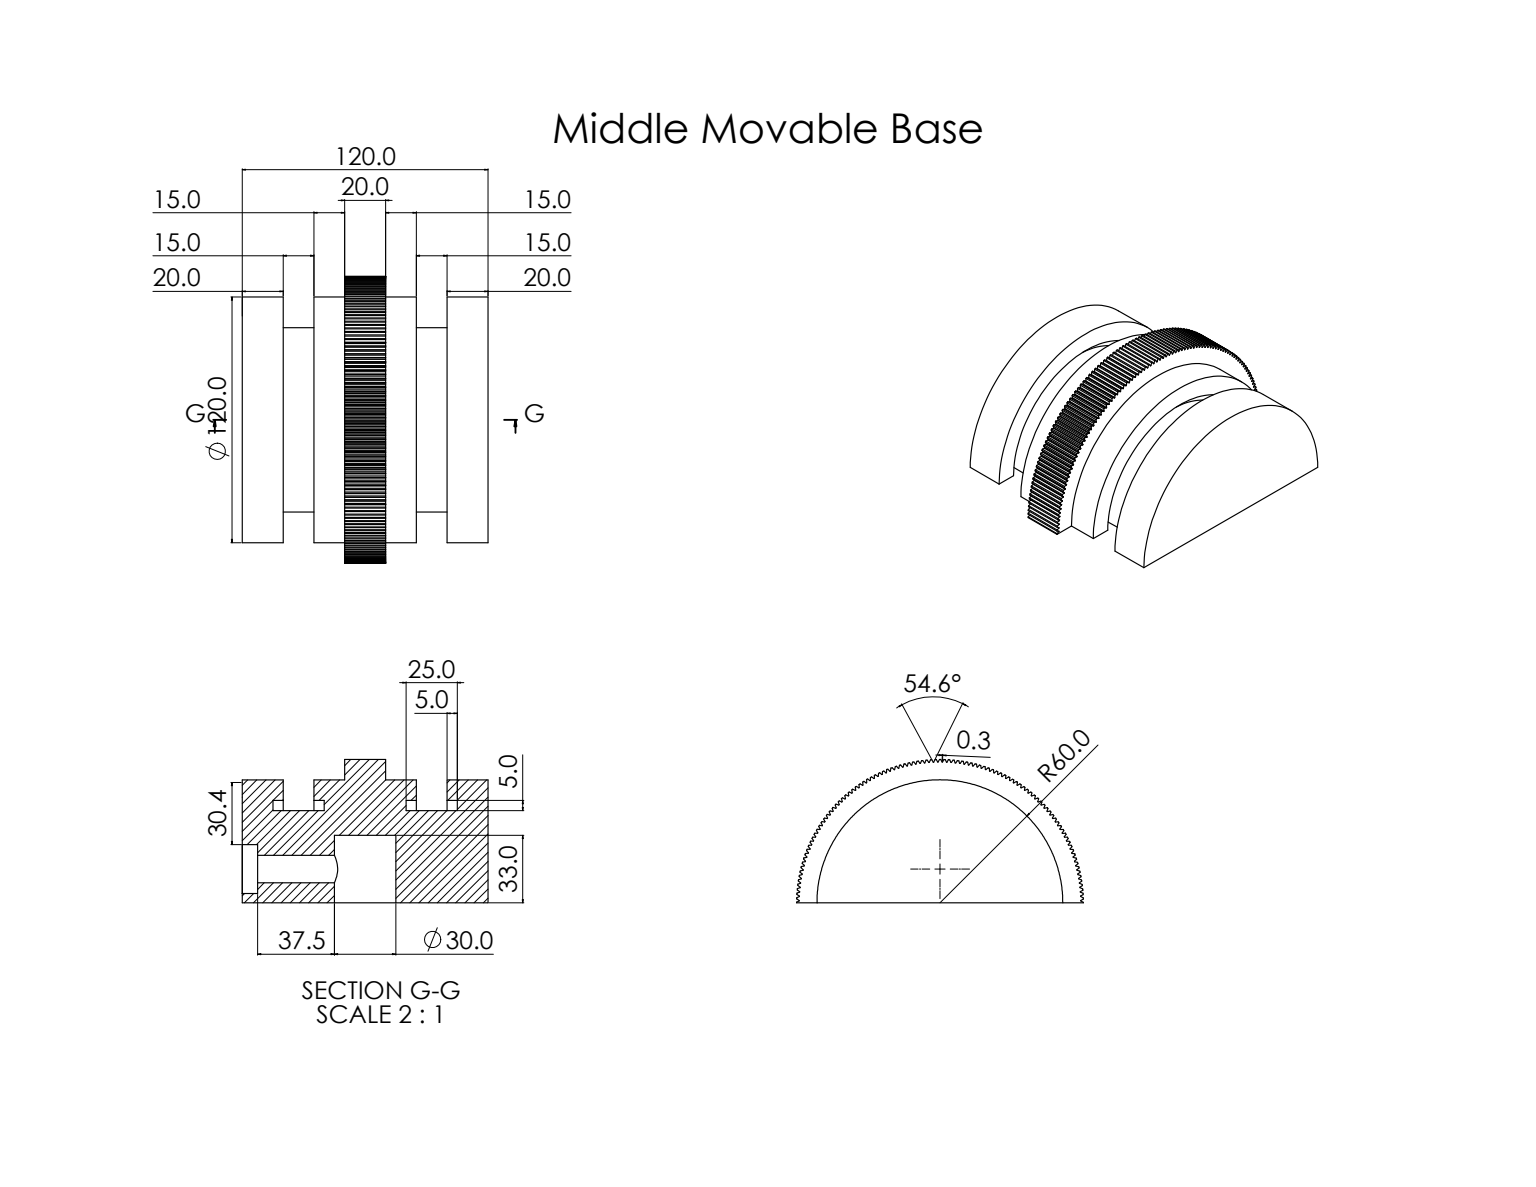
ISO-10303-21;
HEADER;
FILE_DESCRIPTION (('STEP AP214'),
    '1' );
FILE_NAME ('Middle Movable Base.step',
    '2026-10-24T22:31:37',
    ( '' ),
    ( '' ),
    'SwSTEP 2.0',
    'SolidWorks 2025',
    '' );
FILE_SCHEMA (( 'AUTOMOTIVE_DESIGN' ));
ENDSEC;

DATA;
#7=DIRECTION ( 'NONE',  ( -0.5866775868892348811, -0.8098206029990989707, 0.000000000000000000 ) ) ;
#27=DIRECTION ( 'NONE',  ( 0.06115825522547173321, -0.9981280818701455670, 0.000000000000000000 ) ) ;
#30=CARTESIAN_POINT ( 'NONE',  ( 30.34687108590969373, 93.06504152958497400, 45.00000000000000711 ) ) ;
#31=CARTESIAN_POINT ( 'NONE',  ( -19.65312891409030271, 93.06504152958497400, -10.00000000000000888 ) ) ;
#36=VECTOR ( 'NONE', #79966, 1000.000000000000000 ) ;
#39=DIRECTION ( 'NONE',  ( 0.000000000000000000, 0.000000000000000000, 1.000000000000000000 ) ) ;
#58=DIRECTION ( 'NONE',  ( -0.5866775868892348811, -0.8098206029990989707, 0.000000000000000000 ) ) ;
#69=EDGE_LOOP ( 'NONE', ( #91985, #84994, #72800, #59520 ) ) ;
#74=LINE ( 'NONE', #15241, #89935 ) ;
#76=CARTESIAN_POINT ( 'NONE',  ( 47.43014843991451102, 113.9519901285712251, 10.00000000000000000 ) ) ;
#82=LINE ( 'NONE', #92802, #76218 ) ;
#92=ORIENTED_EDGE ( 'NONE', *, *, #79784, .F. ) ;
#93=LINE ( 'NONE', #62359, #20761 ) ;
#99=ORIENTED_EDGE ( 'NONE', *, *, #21399, .F. ) ;
#100=CARTESIAN_POINT ( 'NONE',  ( -11.19568923542803773, 72.02527638617826256, 14.65695210810445737 ) ) ;
#102=FACE_OUTER_BOUND ( 'NONE', #93953, .T. ) ;
#105=ORIENTED_EDGE ( 'NONE', *, *, #46073, .T. ) ;
#118=CARTESIAN_POINT ( 'NONE',  ( 22.66956910419568061, 38.88013629349138256, -10.00000000000000000 ) ) ;
#128=AXIS2_PLACEMENT_3D ( 'NONE', #29113, #74733, #4299 ) ;
#144=DIRECTION ( 'NONE',  ( 1.000000000000000000, 0.000000000000000000, 0.000000000000000000 ) ) ;
#147=DIRECTION ( 'NONE',  ( -0.9979398670145497308, -0.06415622980648832963, 0.000000000000000000 ) ) ;
#157=DIRECTION ( 'NONE',  ( -1.000000000000000000, 0.000000000000000000, 0.000000000000000000 ) ) ;
#166=VERTEX_POINT ( 'NONE', #35811 ) ;
#179=VERTEX_POINT ( 'NONE', #22103 ) ;
#180=CARTESIAN_POINT ( 'NONE',  ( 43.35468487962021555, 120.5828561944265687, -10.00000000000000000 ) ) ;
#182=DIRECTION ( 'NONE',  ( -0.8770933717188628131, -0.4803199113995136327, 0.000000000000000000 ) ) ;
#185=CARTESIAN_POINT ( 'NONE',  ( -77.58047734835668052, 56.02942318228900120, 10.00000000000000000 ) ) ;
#186=EDGE_CURVE ( 'NONE', #58877, #48375, #99124, .T. ) ;
#187=CARTESIAN_POINT ( 'NONE',  ( -37.40701240123932791, 25.35389310390295847, 177.5919119679930134 ) ) ;
#191=VECTOR ( 'NONE', #26487, 1000.000000000000000 ) ;
#192=DIRECTION ( 'NONE',  ( -0.2575544297740129385, 0.9662637919863205083, 0.000000000000000000 ) ) ;
#195=LINE ( 'NONE', #21507, #68091 ) ;
#198=LINE ( 'NONE', #694, #6256 ) ;
#199=DIRECTION ( 'NONE',  ( -0.1269555777209495084, -0.9919084036772447543, 0.000000000000000000 ) ) ;
#201=DIRECTION ( 'NONE',  ( -0.9956898167541090583, 0.09274582908232942291, 0.000000000000000000 ) ) ;
#205=ORIENTED_EDGE ( 'NONE', *, *, #96749, .F. ) ;
#209=ORIENTED_EDGE ( 'NONE', *, *, #18748, .T. ) ;
#210=ADVANCED_FACE ( 'NONE', ( #82475 ), #75330, .F. ) ;
#211=EDGE_CURVE ( 'NONE', #97533, #84233, #8682, .T. ) ;
#212=ORIENTED_EDGE ( 'NONE', *, *, #13551, .F. ) ;
#213=VERTEX_POINT ( 'NONE', #51000 ) ;
#215=ORIENTED_EDGE ( 'NONE', *, *, #48377, .F. ) ;
#216=CARTESIAN_POINT ( 'NONE',  ( -34.42581292930597670, 25.91608375674935161, -10.00000000000000000 ) ) ;
#223=EDGE_CURVE ( 'NONE', #61495, #4321, #98638, .T. ) ;
#226=CARTESIAN_POINT ( 'NONE',  ( -38.08094845355783065, 65.40755614729289391, -10.00000000000000000 ) ) ;
#231=EDGE_LOOP ( 'NONE', ( #23374, #30336, #91707, #91795 ) ) ;
#234=CARTESIAN_POINT ( 'NONE',  ( 32.49301573174289359, 102.6727471919249552, 59.99999999999999289 ) ) ;
#235=EDGE_CURVE ( 'NONE', #80145, #45676, #581, .T. ) ;
#237=PLANE ( 'NONE',  #70015 ) ;
#241=ORIENTED_EDGE ( 'NONE', *, *, #65257, .F. ) ;
#243=CARTESIAN_POINT ( 'NONE',  ( -5.171971415982786979, 24.31384663199769491, -10.00000000000000000 ) ) ;
#249=CARTESIAN_POINT ( 'NONE',  ( 19.31801425620939483, 115.5650415295850451, 45.00000000000000711 ) ) ;
#251=DIRECTION ( 'NONE',  ( -0.7299047266382377996, 0.6835488936653758563, 0.000000000000000000 ) ) ;
#253=LINE ( 'NONE', #93489, #65775 ) ;
#260=VECTOR ( 'NONE', #98642, 1000.000000000000000 ) ;
#270=DIRECTION ( 'NONE',  ( 0.000000000000000000, 0.000000000000000000, 1.000000000000000000 ) ) ;
#280=FACE_OUTER_BOUND ( 'NONE', #77196, .T. ) ;
#282=CARTESIAN_POINT ( 'NONE',  ( 45.86253193465722688, 68.41350641406140198, -10.00000000000000000 ) ) ;
#287=EDGE_CURVE ( 'NONE', #95521, #97948, #4932, .T. ) ;
#289=CARTESIAN_POINT ( 'NONE',  ( 48.58805178314242568, 84.67719436603331928, -10.00000000000000000 ) ) ;
#295=DIRECTION ( 'NONE',  ( -0.000000000000000000, 0.000000000000000000, -1.000000000000000000 ) ) ;
#297=ORIENTED_EDGE ( 'NONE', *, *, #4120, .T. ) ;
#303=EDGE_CURVE ( 'NONE', #60481, #57725, #20128, .T. ) ;
#304=ORIENTED_EDGE ( 'NONE', *, *, #16098, .T. ) ;
#317=CARTESIAN_POINT ( 'NONE',  ( -19.77952770554638207, 93.00072136042149396, 59.99999999999999289 ) ) ;
#326=DIRECTION ( 'NONE',  ( 0.2091919045418403900, 0.9778746070300412541, 0.000000000000000000 ) ) ;
#333=ORIENTED_EDGE ( 'NONE', *, *, #33379, .F. ) ;
#337=CARTESIAN_POINT ( 'NONE',  ( 48.83428215874786815, 87.09189275153327969, -10.00000000000000000 ) ) ;
#353=DIRECTION ( 'NONE',  ( -0.000000000000000000, -0.000000000000000000, 1.000000000000000000 ) ) ;
#354=CARTESIAN_POINT ( 'NONE',  ( -19.56589364647650697, 93.17686168307763239, 59.99999999999999289 ) ) ;
#357=CARTESIAN_POINT ( 'NONE',  ( -54.25007008209492199, 32.21233689110872689, 10.00000000000000000 ) ) ;
#366=LINE ( 'NONE', #79411, #99707 ) ;
#367=ORIENTED_EDGE ( 'NONE', *, *, #49379, .F. ) ;
#372=PLANE ( 'NONE',  #40302 ) ;
#384=CARTESIAN_POINT ( 'NONE',  ( 45.79324619304848909, 117.8999360398438512, 177.5919119679930134 ) ) ;
#390=CARTESIAN_POINT ( 'NONE',  ( -59.85755863633952600, 35.44530052843370527, 10.00000000000000000 ) ) ;
#392=DIRECTION ( 'NONE',  ( -1.000000000000000000, 0.000000000000000000, 0.000000000000000000 ) ) ;
#393=EDGE_CURVE ( 'NONE', #90851, #29361, #37739, .T. ) ;
#414=DIRECTION ( 'NONE',  ( -0.2270762630343793331, 0.9738769792773321887, 0.000000000000000000 ) ) ;
#433=CARTESIAN_POINT ( 'NONE',  ( 32.24342178309110096, 47.97677246190463052, 10.00000000000000000 ) ) ;
#438=CARTESIAN_POINT ( 'NONE',  ( -47.78078991586326651, 28.96484896693080913, -10.00000000000000000 ) ) ;
#442=LINE ( 'NONE', #39415, #16658 ) ;
#451=AXIS2_PLACEMENT_3D ( 'NONE', #67847, #36429, #6548 ) ;
#466=VECTOR ( 'NONE', #65332, 1000.000000000000114 ) ;
#472=ORIENTED_EDGE ( 'NONE', *, *, #57842, .T. ) ;
#477=DIRECTION ( 'NONE',  ( -0.000000000000000000, 0.000000000000000000, 1.000000000000000000 ) ) ;
#484=ADVANCED_BREP_SHAPE_REPRESENTATION ( '', ( #42857, #68784 ), #81782 ) ;
#485=ORIENTED_EDGE ( 'NONE', *, *, #51159, .T. ) ;
#494=CARTESIAN_POINT ( 'NONE',  ( -80.08603253397791377, 57.73992072201551906, 177.5919119679930134 ) ) ;
#498=CARTESIAN_POINT ( 'NONE',  ( -59.87889494062799400, 37.30571521936384016, 10.00000000000000000 ) ) ;
#509=FACE_OUTER_BOUND ( 'NONE', #80990, .T. ) ;
#511=VERTEX_POINT ( 'NONE', #55477 ) ;
#515=CARTESIAN_POINT ( 'NONE',  ( -29.31672308591111431, 23.47304723416778316, -10.00000000000000000 ) ) ;
#518=CIRCLE ( 'NONE', #92746, 0.1418229129680845801 ) ;
#521=FACE_OUTER_BOUND ( 'NONE', #76798, .T. ) ;
#525=CARTESIAN_POINT ( 'NONE',  ( 48.98007068238331385, 88.97864505566217019, 10.00000000000000000 ) ) ;
#526=VERTEX_POINT ( 'NONE', #86463 ) ;
#527=VECTOR ( 'NONE', #79353, 1000.000000000000000 ) ;
#540=EDGE_CURVE ( 'NONE', #56147, #90103, #63596, .T. ) ;
#553=PLANE ( 'NONE',  #11961 ) ;
#560=DIRECTION ( 'NONE',  ( -0.000000000000000000, -0.000000000000000000, -1.000000000000000000 ) ) ;
#561=ORIENTED_EDGE ( 'NONE', *, *, #16214, .T. ) ;
#566=VERTEX_POINT ( 'NONE', #60825 ) ;
#575=ORIENTED_EDGE ( 'NONE', *, *, #83693, .F. ) ;
#581=CIRCLE ( 'NONE', #62027, 70.00000000000001421 ) ;
#582=ORIENTED_EDGE ( 'NONE', *, *, #61102, .F. ) ;
#583=DIRECTION ( 'NONE',  ( -0.000000000000000000, -0.000000000000000000, -1.000000000000000000 ) ) ;
#590=CARTESIAN_POINT ( 'NONE',  ( -8.413379660334708632, 72.70744834316617755, 14.99993878877685916 ) ) ;
#591=LINE ( 'NONE', #85759, #53118 ) ;
#627=ADVANCED_FACE ( 'NONE', ( #24842 ), #553, .F. ) ;
#642=DIRECTION ( 'NONE',  ( -0.000000000000000000, 0.000000000000000000, 1.000000000000000000 ) ) ;
#652=DIRECTION ( 'NONE',  ( 0.000000000000000000, 0.000000000000000000, 1.000000000000000000 ) ) ;
#654=DIRECTION ( 'NONE',  ( 0.3074612162317589825, -0.9515606131578205895, 0.000000000000000000 ) ) ;
#673=VECTOR ( 'NONE', #77839, 1000.000000000000227 ) ;
#676=ORIENTED_EDGE ( 'NONE', *, *, #27395, .T. ) ;
#694=CARTESIAN_POINT ( 'NONE',  ( 48.58805178314242568, 84.67719436603331928, 10.00000000000000000 ) ) ;
#697=CARTESIAN_POINT ( 'NONE',  ( -74.97640825042664403, 52.25402898078436920, -10.00000000000000000 ) ) ;
#701=ORIENTED_EDGE ( 'NONE', *, *, #49835, .T. ) ;
#703=DIRECTION ( 'NONE',  ( 0.000000000000000000, 0.000000000000000000, 1.000000000000000000 ) ) ;
#706=ORIENTED_EDGE ( 'NONE', *, *, #49315, .T. ) ;
#709=VERTEX_POINT ( 'NONE', #54730 ) ;
#710=DIRECTION ( 'NONE',  ( -0.6141984594095433181, -0.7891516029629183082, 0.000000000000000000 ) ) ;
#717=DIRECTION ( 'NONE',  ( 1.000000000000000000, -2.577303450022684150E-15, 0.000000000000000000 ) ) ;
#720=EDGE_CURVE ( 'NONE', #17180, #93223, #32942, .T. ) ;
#724=ORIENTED_EDGE ( 'NONE', *, *, #71091, .F. ) ;
#726=CARTESIAN_POINT ( 'NONE',  ( -72.48190909937208914, 49.06123820388767598, -10.00000000000000000 ) ) ;
#728=DIRECTION ( 'NONE',  ( -0.000000000000000000, -0.000000000000000000, -1.000000000000000000 ) ) ;
#760=CARTESIAN_POINT ( 'NONE',  ( -14.53296615039140960, 35.34728565592875071, 59.99999999999999289 ) ) ;
#764=LINE ( 'NONE', #54961, #11155 ) ;
#771=LINE ( 'NONE', #16967, #7881 ) ;
#775=ORIENTED_EDGE ( 'NONE', *, *, #59166, .F. ) ;
#782=FACE_OUTER_BOUND ( 'NONE', #41307, .T. ) ;
#796=ADVANCED_FACE ( 'NONE', ( #63846 ), #32453, .F. ) ;
#797=ORIENTED_EDGE ( 'NONE', *, *, #34932, .T. ) ;
#802=CARTESIAN_POINT ( 'NONE',  ( 39.77289032284285497, 58.49985355908045648, -10.00000000000000000 ) ) ;
#812=CIRCLE ( 'NONE', #62261, 70.00000000000001421 ) ;
#820=CARTESIAN_POINT ( 'NONE',  ( 18.86034532297697908, 34.61239144260639478, -10.00000000000000000 ) ) ;
#824=ORIENTED_EDGE ( 'NONE', *, *, #18196, .F. ) ;
#843=VECTOR ( 'NONE', #25615, 1000.000000000000000 ) ;
#861=VERTEX_POINT ( 'NONE', #26360 ) ;
#871=ORIENTED_EDGE ( 'NONE', *, *, #19349, .T. ) ;
#877=ADVANCED_FACE ( 'NONE', ( #35443 ), #33453, .F. ) ;
#880=VECTOR ( 'NONE', #94818, 999.9999999999998863 ) ;
#882=FACE_OUTER_BOUND ( 'NONE', #77373, .T. ) ;
#895=DIRECTION ( 'NONE',  ( 1.000000000000000000, 0.000000000000000000, 0.000000000000000000 ) ) ;
#899=EDGE_CURVE ( 'NONE', #47394, #59009, #20762, .T. ) ;
#910=EDGE_CURVE ( 'NONE', #22139, #62627, #36935, .T. ) ;
#913=CARTESIAN_POINT ( 'NONE',  ( -54.24312371938221133, 45.66933727564025247, 59.99999999999999289 ) ) ;
#915=CARTESIAN_POINT ( 'NONE',  ( -37.96271243472389756, 25.23297040071578223, -10.00000000000000000 ) ) ;
#916=VECTOR ( 'NONE', #19818, 1000.000000000000000 ) ;
#926=PLANE ( 'NONE',  #45711 ) ;
#934=VERTEX_POINT ( 'NONE', #51650 ) ;
#942=DIRECTION ( 'NONE',  ( -0.000000000000000000, -0.000000000000000000, -1.000000000000000000 ) ) ;
#943=ORIENTED_EDGE ( 'NONE', *, *, #73759, .T. ) ;
#946=FACE_OUTER_BOUND ( 'NONE', #38925, .T. ) ;
#953=ORIENTED_EDGE ( 'NONE', *, *, #83634, .T. ) ;
#956=AXIS2_PLACEMENT_3D ( 'NONE', #84126, #36465, #99782 ) ;
#961=CYLINDRICAL_SURFACE ( 'NONE', #15742, 70.00000000000002842 ) ;
#981=DIRECTION ( 'NONE',  ( -0.9999990636452668058, -0.001368469433204011270, 0.000000000000000000 ) ) ;
#984=ORIENTED_EDGE ( 'NONE', *, *, #57106, .F. ) ;
#988=LINE ( 'NONE', #76978, #61278 ) ;
#989=EDGE_CURVE ( 'NONE', #100173, #64867, #53135, .T. ) ;
#991=VECTOR ( 'NONE', #68257, 1000.000000000000000 ) ;
#996=EDGE_LOOP ( 'NONE', ( #34380, #44799, #80487, #3308 ) ) ;
#1005=CARTESIAN_POINT ( 'NONE',  ( 50.33662733789741139, 94.26254718190894266, -10.00000000000000000 ) ) ;
#1023=LINE ( 'NONE', #92751, #45256 ) ;
#1027=EDGE_CURVE ( 'NONE', #65437, #26008, #58647, .T. ) ;
#1030=VERTEX_POINT ( 'NONE', #52623 ) ;
#1052=CARTESIAN_POINT ( 'NONE',  ( -4.696103426644111956, 79.65490786025929992, 13.63766756523351020 ) ) ;
#1054=DIRECTION ( 'NONE',  ( -0.9954067278227237692, 0.09573633691163400961, 0.000000000000000000 ) ) ;
#1064=VECTOR ( 'NONE', #92848, 999.9999999999998863 ) ;
#1080=ORIENTED_EDGE ( 'NONE', *, *, #21239, .T. ) ;
#1085=EDGE_CURVE ( 'NONE', #56387, #18338, #31160, .T. ) ;
#1091=CIRCLE ( 'NONE', #54496, 70.00000000000001421 ) ;
#1098=VERTEX_POINT ( 'NONE', #99752 ) ;
#1101=DIRECTION ( 'NONE',  ( 1.000000000000000000, 1.070572202317114942E-14, 0.000000000000000000 ) ) ;
#1102=CIRCLE ( 'NONE', #14042, 70.00000000000001421 ) ;
#1103=VERTEX_POINT ( 'NONE', #60710 ) ;
#1122=DIRECTION ( 'NONE',  ( -1.000000000000000000, 0.000000000000000000, 0.000000000000000000 ) ) ;
#1126=EDGE_CURVE ( 'NONE', #56387, #14902, #59211, .T. ) ;
#1143=ORIENTED_EDGE ( 'NONE', *, *, #74016, .T. ) ;
#1144=CARTESIAN_POINT ( 'NONE',  ( -19.70914744582199774, 92.93475084401866582, 59.99999999999999289 ) ) ;
#1150=CARTESIAN_POINT ( 'NONE',  ( -30.95603806669010183, 23.98360954755323604, 177.5919119679930134 ) ) ;
#1152=VECTOR ( 'NONE', #12982, 1000.000000000000000 ) ;
#1153=EDGE_CURVE ( 'NONE', #7407, #88206, #54605, .T. ) ;
#1156=ORIENTED_EDGE ( 'NONE', *, *, #93985, .F. ) ;
#1161=CIRCLE ( 'NONE', #65869, 0.1418229129681522482 ) ;
#1162=CARTESIAN_POINT ( 'NONE',  ( 49.07456115661583596, 91.13648234292965356, -10.00000000000000000 ) ) ;
#1170=ORIENTED_EDGE ( 'NONE', *, *, #72286, .F. ) ;
#1173=DIRECTION ( 'NONE',  ( -0.8965230319888208843, 0.4429971254010250936, 0.000000000000000000 ) ) ;
#1174=VECTOR ( 'NONE', #10627, 1000.000000000000000 ) ;
#1178=DIRECTION ( 'NONE',  ( 0.000000000000000000, 0.000000000000000000, 1.000000000000000000 ) ) ;
#1184=ORIENTED_EDGE ( 'NONE', *, *, #47229, .T. ) ;
#1186=EDGE_CURVE ( 'NONE', #36969, #71264, #84573, .T. ) ;
#1197=VERTEX_POINT ( 'NONE', #62209 ) ;
#1199=FACE_OUTER_BOUND ( 'NONE', #92317, .T. ) ;
#1203=CARTESIAN_POINT ( 'NONE',  ( 10.24016918245798990, 49.27098784156451217, 59.99999999999999289 ) ) ;
#1204=ORIENTED_EDGE ( 'NONE', *, *, #57213, .F. ) ;
#1210=ORIENTED_EDGE ( 'NONE', *, *, #81477, .F. ) ;
#1216=ORIENTED_EDGE ( 'NONE', *, *, #59052, .T. ) ;
#1217=ORIENTED_EDGE ( 'NONE', *, *, #67248, .F. ) ;
#1218=VERTEX_POINT ( 'NONE', #22738 ) ;
#1220=ORIENTED_EDGE ( 'NONE', *, *, #11993, .T. ) ;
#1228=FACE_OUTER_BOUND ( 'NONE', #56169, .T. ) ;
#1229=DIRECTION ( 'NONE',  ( -0.9515606131578174809, -0.3074612162317687525, 0.000000000000000000 ) ) ;
#1235=VERTEX_POINT ( 'NONE', #433 ) ;
#1247=VECTOR ( 'NONE', #98615, 1000.000000000000000 ) ;
#1257=DIRECTION ( 'NONE',  ( -0.9054088711727240613, 0.4245406647209821749, 0.000000000000000000 ) ) ;
#1261=EDGE_LOOP ( 'NONE', ( #21247, #73872, #79004, #53676 ) ) ;
#1262=ORIENTED_EDGE ( 'NONE', *, *, #86789, .T. ) ;
#1272=AXIS2_PLACEMENT_3D ( 'NONE', #72427, #95248, #88660 ) ;
#1277=CIRCLE ( 'NONE', #57894, 0.1418229129681557177 ) ;
#1280=VECTOR ( 'NONE', #33335, 1000.000000000000227 ) ;
#1281=DIRECTION ( 'NONE',  ( 0.8599083858334037878, -0.5104483989331242144, 0.000000000000000000 ) ) ;
#1290=VERTEX_POINT ( 'NONE', #69581 ) ;
#1297=PLANE ( 'NONE',  #6369 ) ;
#1298=VECTOR ( 'NONE', #47765, 1000.000000000000114 ) ;
#1300=DIRECTION ( 'NONE',  ( 0.9616534368410327716, -0.2742675106749429270, 0.000000000000000000 ) ) ;
#1304=EDGE_CURVE ( 'NONE', #56569, #52500, #99009, .T. ) ;
#1316=EDGE_CURVE ( 'NONE', #35809, #20300, #83330, .T. ) ;
#1319=AXIS2_PLACEMENT_3D ( 'NONE', #28738, #47412, #55498 ) ;
#1320=ORIENTED_EDGE ( 'NONE', *, *, #44937, .T. ) ;
#1324=ORIENTED_EDGE ( 'NONE', *, *, #63685, .T. ) ;
#1333=CARTESIAN_POINT ( 'NONE',  ( 38.19908180566553568, 96.33262850695970769, 59.99999999999999289 ) ) ;
#1334=DIRECTION ( 'NONE',  ( -0.1344185706417126702, 0.9909246428798905715, 0.000000000000000000 ) ) ;
#1336=ORIENTED_EDGE ( 'NONE', *, *, #16346, .T. ) ;
#1339=ORIENTED_EDGE ( 'NONE', *, *, #72669, .F. ) ;
#1353=VECTOR ( 'NONE', #63954, 1000.000000000000000 ) ;
#1359=AXIS2_PLACEMENT_3D ( 'NONE', #81029, #56669, #96213 ) ;
#1363=EDGE_CURVE ( 'NONE', #22179, #13198, #68582, .T. ) ;
#1368=DIRECTION ( 'NONE',  ( 0.9481851146622169990, 0.3177184104407523302, 0.000000000000000000 ) ) ;
#1371=DIRECTION ( 'NONE',  ( -0.000000000000000000, 0.000000000000000000, 1.000000000000000000 ) ) ;
#1376=VERTEX_POINT ( 'NONE', #59470 ) ;
#1377=EDGE_CURVE ( 'NONE', #70239, #29279, #92426, .T. ) ;
#1379=EDGE_CURVE ( 'NONE', #37194, #36369, #53381, .T. ) ;
#1380=VECTOR ( 'NONE', #44212, 1000.000000000000000 ) ;
#1398=AXIS2_PLACEMENT_3D ( 'NONE', #5621, #66429, #99340 ) ;
#1428=EDGE_CURVE ( 'NONE', #28142, #18551, #60972, .T. ) ;
#1434=PLANE ( 'NONE',  #38359 ) ;
#1436=VECTOR ( 'NONE', #17514, 1000.000000000000000 ) ;
#1438=DIRECTION ( 'NONE',  ( 1.000000000000000000, 0.000000000000000000, 0.000000000000000000 ) ) ;
#1442=AXIS2_PLACEMENT_3D ( 'NONE', #13783, #67983, #44661 ) ;
#1454=ORIENTED_EDGE ( 'NONE', *, *, #94923, .T. ) ;
#1455=CARTESIAN_POINT ( 'NONE',  ( -42.18579364100346396, 26.51648975995176372, -10.00000000000000000 ) ) ;
#1459=VECTOR ( 'NONE', #70154, 1000.000000000000227 ) ;
#1466=DIRECTION ( 'NONE',  ( -0.000000000000000000, 0.000000000000000000, -1.000000000000000000 ) ) ;
#1468=LINE ( 'NONE', #48042, #82103 ) ;
#1473=CARTESIAN_POINT ( 'NONE',  ( -19.65312891409030271, 93.06504152958497400, 10.00000000000000888 ) ) ;
#1479=DIRECTION ( 'NONE',  ( -0.4805540241036398430, -0.8769651246872923744, 0.000000000000000000 ) ) ;
#1484=ORIENTED_EDGE ( 'NONE', *, *, #28389, .T. ) ;
#1487=ORIENTED_EDGE ( 'NONE', *, *, #98535, .T. ) ;
#1499=VECTOR ( 'NONE', #42114, 1000.000000000000000 ) ;
#1513=EDGE_CURVE ( 'NONE', #39405, #4020, #94422, .T. ) ;
#1517=CARTESIAN_POINT ( 'NONE',  ( -4.164184202058353712, 36.47075635815506445, 59.99999999999999289 ) ) ;
#1534=LINE ( 'NONE', #95271, #4496 ) ;
#1538=CARTESIAN_POINT ( 'NONE',  ( -19.65312891409030271, 93.06504152958497400, -20.00000000000000355 ) ) ;
#1545=LINE ( 'NONE', #8630, #17652 ) ;
#1568=FACE_OUTER_BOUND ( 'NONE', #50419, .T. ) ;
#1569=ORIENTED_EDGE ( 'NONE', *, *, #56933, .F. ) ;
#1571=LINE ( 'NONE', #30084, #19936 ) ;
#1579=CIRCLE ( 'NONE', #89003, 70.00000000000001421 ) ;
#1583=EDGE_CURVE ( 'NONE', #75006, #51318, #47275, .T. ) ;
#1592=VERTEX_POINT ( 'NONE', #42660 ) ;
#1595=ORIENTED_EDGE ( 'NONE', *, *, #6391, .T. ) ;
#1603=AXIS2_PLACEMENT_3D ( 'NONE', #71225, #8410, #94542 ) ;
#1621=CARTESIAN_POINT ( 'NONE',  ( 20.94141239725287917, 35.71947554534623492, -10.00000000000000000 ) ) ;
#1624=LINE ( 'NONE', #53298, #100278 ) ;
#1628=EDGE_CURVE ( 'NONE', #64662, #76974, #18907, .T. ) ;
#1636=ORIENTED_EDGE ( 'NONE', *, *, #79163, .F. ) ;
#1644=VERTEX_POINT ( 'NONE', #91305 ) ;
#1653=PLANE ( 'NONE',  #7779 ) ;
#1666=ORIENTED_EDGE ( 'NONE', *, *, #83634, .F. ) ;
#1673=DIRECTION ( 'NONE',  ( 0.4140345431502788220, 0.9102611697080897901, 0.000000000000000000 ) ) ;
#1691=CARTESIAN_POINT ( 'NONE',  ( 31.79857739925353499, 98.44139654353648439, 59.99999999999999289 ) ) ;
#1696=CARTESIAN_POINT ( 'NONE',  ( -0.2492734796364602656, 27.10516647459198225, -10.00000000000000000 ) ) ;
#1707=EDGE_CURVE ( 'NONE', #24773, #78854, #42513, .T. ) ;
#1711=ORIENTED_EDGE ( 'NONE', *, *, #9867, .F. ) ;
#1716=CARTESIAN_POINT ( 'NONE',  ( 27.76992210170819675, 43.29297894285233639, -10.00000000000000000 ) ) ;
#1725=VERTEX_POINT ( 'NONE', #61355 ) ;
#1731=CARTESIAN_POINT ( 'NONE',  ( 3.854092266844447501, 28.45370138451379560, 10.00000000000000000 ) ) ;
#1733=VERTEX_POINT ( 'NONE', #59861 ) ;
#1734=VERTEX_POINT ( 'NONE', #21866 ) ;
#1745=ORIENTED_EDGE ( 'NONE', *, *, #19548, .F. ) ;
#1754=ADVANCED_FACE ( 'NONE', ( #98395 ), #22860, .F. ) ;
#1756=LINE ( 'NONE', #79786, #92698 ) ;
#1766=DIRECTION ( 'NONE',  ( -0.9182972510888883777, 0.3958915996110437541, 0.000000000000000000 ) ) ;
#1789=DIRECTION ( 'NONE',  ( -0.5803476755362181327, -0.8143688203140567738, 0.000000000000000000 ) ) ;
#1802=DIRECTION ( 'NONE',  ( -0.2197389712097134185, -0.9755587037855265597, 0.000000000000000000 ) ) ;
#1810=LINE ( 'NONE', #17499, #37592 ) ;
#1821=ORIENTED_EDGE ( 'NONE', *, *, #26693, .F. ) ;
#1822=LINE ( 'NONE', #8908, #48804 ) ;
#1835=DIRECTION ( 'NONE',  ( 0.000000000000000000, 0.000000000000000000, 1.000000000000000000 ) ) ;
#1844=ORIENTED_EDGE ( 'NONE', *, *, #76284, .F. ) ;
#1851=CARTESIAN_POINT ( 'NONE',  ( -8.669243101527598583, 25.19333184544593252, -10.00000000000000000 ) ) ;
#1860=VERTEX_POINT ( 'NONE', #15750 ) ;
#1866=CARTESIAN_POINT ( 'NONE',  ( -31.49789205211705934, 23.81092751074078606, -10.00000000000000000 ) ) ;
#1869=AXIS2_PLACEMENT_3D ( 'NONE', #180, #45756, #59965 ) ;
#1870=CARTESIAN_POINT ( 'NONE',  ( 22.87549206224920084, 39.05096577487528720, -10.00000000000000000 ) ) ;
#1871=ORIENTED_EDGE ( 'NONE', *, *, #27551, .T. ) ;
#1876=PLANE ( 'NONE',  #87255 ) ;
#1879=DIRECTION ( 'NONE',  ( -0.9606745773021557744, 0.2776767122488390527, 0.000000000000000000 ) ) ;
#1880=EDGE_CURVE ( 'NONE', #50442, #29620, #8170, .T. ) ;
#1885=EDGE_LOOP ( 'NONE', ( #41574, #54395, #87632, #40774 ) ) ;
#1888=LINE ( 'NONE', #72303, #26415 ) ;
#1903=FACE_OUTER_BOUND ( 'NONE', #32599, .T. ) ;
#1907=DIRECTION ( 'NONE',  ( 1.000000000000000000, 0.000000000000000000, 0.000000000000000000 ) ) ;
#1919=CARTESIAN_POINT ( 'NONE',  ( -19.65312891409030271, 93.06504152958497400, -10.00000000000000888 ) ) ;
#1921=DIRECTION ( 'NONE',  ( 1.000000000000000000, -1.199437374818249260E-13, 0.000000000000000000 ) ) ;
#1926=EDGE_LOOP ( 'NONE', ( #76923, #39186, #42296, #5688 ) ) ;
#1935=DIRECTION ( 'NONE',  ( 0.4242989612870596283, -0.9055221650797523614, 0.000000000000000000 ) ) ;
#1937=ORIENTED_EDGE ( 'NONE', *, *, #70332, .F. ) ;
#1943=CARTESIAN_POINT ( 'NONE',  ( -53.68831936616819434, 31.89637462494507147, -10.00000000000000000 ) ) ;
#1945=ORIENTED_EDGE ( 'NONE', *, *, #26582, .F. ) ;
#1951=VERTEX_POINT ( 'NONE', #77056 ) ;
#1956=DIRECTION ( 'NONE',  ( -0.1269555777209495362, -0.9919084036772447543, 0.000000000000000000 ) ) ;
#1958=EDGE_LOOP ( 'NONE', ( #58734, #50426 ) ) ;
#1959=VERTEX_POINT ( 'NONE', #54744 ) ;
#1972=VERTEX_POINT ( 'NONE', #93296 ) ;
#1974=LINE ( 'NONE', #48575, #80408 ) ;
#1981=LINE ( 'NONE', #93203, #78611 ) ;
#1989=VERTEX_POINT ( 'NONE', #86721 ) ;
#1995=LINE ( 'NONE', #24779, #44472 ) ;
#2008=DIRECTION ( 'NONE',  ( 0.6361630342459738685, -0.7715546603183444097, 0.000000000000000000 ) ) ;
#2035=VECTOR ( 'NONE', #52050, 1000.000000000000114 ) ;
#2043=EDGE_CURVE ( 'NONE', #50852, #69710, #86222, .T. ) ;
#2062=DIRECTION ( 'NONE',  ( 0.9974094913373514615, 0.07193265315672570104, 0.000000000000000000 ) ) ;
#2070=ORIENTED_EDGE ( 'NONE', *, *, #10876, .T. ) ;
#2073=ADVANCED_FACE ( 'NONE', ( #1903 ), #56585, .F. ) ;
#2078=ORIENTED_EDGE ( 'NONE', *, *, #27213, .T. ) ;
#2081=CARTESIAN_POINT ( 'NONE',  ( -19.65312891409030271, 93.06504152958497400, -10.00000000000000888 ) ) ;
#2097=DIRECTION ( 'NONE',  ( -0.6544109481086123337, -0.7561390817803210762, 0.000000000000000000 ) ) ;
#2112=VERTEX_POINT ( 'NONE', #86063 ) ;
#2115=DIRECTION ( 'NONE',  ( -0.7511915808658273797, -0.6600842437418872333, 0.000000000000000000 ) ) ;
#2128=CARTESIAN_POINT ( 'NONE',  ( 31.50071699975810091, 85.35483982831681260, 59.99999999999999289 ) ) ;
#2129=EDGE_CURVE ( 'NONE', #25226, #26753, #87573, .T. ) ;
#2191=LINE ( 'NONE', #94910, #43241 ) ;
#2192=VERTEX_POINT ( 'NONE', #42862 ) ;
#2200=EDGE_CURVE ( 'NONE', #39565, #54118, #11015, .T. ) ;
#2212=VECTOR ( 'NONE', #60192, 1000.000000000000114 ) ;
#2214=ORIENTED_EDGE ( 'NONE', *, *, #3427, .F. ) ;
#2232=ORIENTED_EDGE ( 'NONE', *, *, #97469, .T. ) ;
#2244=LINE ( 'NONE', #33123, #75801 ) ;
#2248=DIRECTION ( 'NONE',  ( 1.000000000000000000, 0.000000000000000000, 0.000000000000000000 ) ) ;
#2253=DIRECTION ( 'NONE',  ( 0.000000000000000000, 0.000000000000000000, 1.000000000000000000 ) ) ;
#2255=DIRECTION ( 'NONE',  ( -0.4527707594502665689, -0.8916269620120450545, 0.000000000000000000 ) ) ;
#2261=FACE_OUTER_BOUND ( 'NONE', #27980, .T. ) ;
#2262=DIRECTION ( 'NONE',  ( -1.000000000000000000, 0.000000000000000000, 0.000000000000000000 ) ) ;
#2267=CARTESIAN_POINT ( 'NONE',  ( 28.41076618884173044, 115.4572390722850912, 59.99999999999999289 ) ) ;
#2280=LINE ( 'NONE', #79315, #64508 ) ;
#2281=AXIS2_PLACEMENT_3D ( 'NONE', #51796, #83720, #82735 ) ;
#2282=CARTESIAN_POINT ( 'NONE',  ( 49.74924850768368145, 83.93760989710258968, -10.00000000000000000 ) ) ;
#2289=ORIENTED_EDGE ( 'NONE', *, *, #38391, .T. ) ;
#2315=CARTESIAN_POINT ( 'NONE',  ( -10.80656490723494123, 24.88181024604956804, -10.00000000000000000 ) ) ;
#2317=DIRECTION ( 'NONE',  ( 0.000000000000000000, 0.000000000000000000, 1.000000000000000000 ) ) ;
#2318=ORIENTED_EDGE ( 'NONE', *, *, #21665, .T. ) ;
#2324=LINE ( 'NONE', #48409, #843 ) ;
#2325=DIRECTION ( 'NONE',  ( -0.000000000000000000, 0.000000000000000000, 1.000000000000000000 ) ) ;
#2344=DIRECTION ( 'NONE',  ( 0.8263106059122495850, 0.5632146860273895550, 0.000000000000000000 ) ) ;
#2361=DIRECTION ( 'NONE',  ( -0.000000000000000000, 0.000000000000000000, -1.000000000000000000 ) ) ;
#2362=VECTOR ( 'NONE', #18549, 1000.000000000000000 ) ;
#2376=PLANE ( 'NONE',  #7947 ) ;
#2380=DIRECTION ( 'NONE',  ( 0.000000000000000000, 0.000000000000000000, 1.000000000000000000 ) ) ;
#2381=VERTEX_POINT ( 'NONE', #54441 ) ;
#2393=ORIENTED_EDGE ( 'NONE', *, *, #31168, .T. ) ;
#2402=PLANE ( 'NONE',  #90238 ) ;
#2409=ADVANCED_FACE ( 'NONE', ( #94401 ), #47256, .F. ) ;
#2418=LINE ( 'NONE', #65685, #91587 ) ;
#2420=CIRCLE ( 'NONE', #34724, 0.1418229129680828593 ) ;
#2435=CARTESIAN_POINT ( 'NONE',  ( -25.57896346879523364, 41.67372163389741502, 59.99999999999999289 ) ) ;
#2440=LINE ( 'NONE', #86577, #73966 ) ;
#2444=ORIENTED_EDGE ( 'NONE', *, *, #32642, .T. ) ;
#2453=DIRECTION ( 'NONE',  ( 0.08592509128337570690, -0.9963016002636669866, 0.000000000000000000 ) ) ;
#2457=ORIENTED_EDGE ( 'NONE', *, *, #68326, .T. ) ;
#2461=EDGE_CURVE ( 'NONE', #55260, #55159, #55344, .T. ) ;
#2463=VECTOR ( 'NONE', #73111, 1000.000000000000227 ) ;
#2469=PLANE ( 'NONE',  #31919 ) ;
#2471=ORIENTED_EDGE ( 'NONE', *, *, #85259, .F. ) ;
#2475=DIRECTION ( 'NONE',  ( 1.000000000000000000, 0.000000000000000000, 0.000000000000000000 ) ) ;
#2487=ORIENTED_EDGE ( 'NONE', *, *, #17553, .T. ) ;
#2497=ORIENTED_EDGE ( 'NONE', *, *, #47982, .F. ) ;
#2501=EDGE_LOOP ( 'NONE', ( #57636, #79002, #91081, #29969 ) ) ;
#2503=CARTESIAN_POINT ( 'NONE',  ( 47.78135487164287554, 106.4364430393875267, 10.00000000000000000 ) ) ;
#2506=LINE ( 'NONE', #19217, #63935 ) ;
#2517=ORIENTED_EDGE ( 'NONE', *, *, #5755, .T. ) ;
#2525=CARTESIAN_POINT ( 'NONE',  ( -19.65312891409030271, 93.06504152958497400, 10.00000000000000888 ) ) ;
#2526=EDGE_CURVE ( 'NONE', #91993, #81911, #518, .T. ) ;
#2528=AXIS2_PLACEMENT_3D ( 'NONE', #87175, #94239, #88163 ) ;
#2534=DIRECTION ( 'NONE',  ( 1.000000000000000000, 0.000000000000000000, 0.000000000000000000 ) ) ;
#2537=DIRECTION ( 'NONE',  ( -1.000000000000000000, 0.000000000000000000, 0.000000000000000000 ) ) ;
#2538=VECTOR ( 'NONE', #67777, 999.9999999999998863 ) ;
#2543=ORIENTED_EDGE ( 'NONE', *, *, #40393, .T. ) ;
#2551=CARTESIAN_POINT ( 'NONE',  ( -48.71813016832984289, 30.75580926756359901, 10.00000000000000000 ) ) ;
#2565=CARTESIAN_POINT ( 'NONE',  ( -6.349302005936061200, 83.25572239057319734, 13.46179068210798668 ) ) ;
#2578=ORIENTED_EDGE ( 'NONE', *, *, #9324, .T. ) ;
#2583=EDGE_LOOP ( 'NONE', ( #3319, #41235, #86461, #66975 ) ) ;
#2589=ORIENTED_EDGE ( 'NONE', *, *, #37624, .F. ) ;
#2601=AXIS2_PLACEMENT_3D ( 'NONE', #65764, #58169, #89153 ) ;
#2602=EDGE_LOOP ( 'NONE', ( #6268, #31875, #84211, #65507 ) ) ;
#2604=EDGE_LOOP ( 'NONE', ( #91400, #73163, #28488, #84955 ) ) ;
#2614=ORIENTED_EDGE ( 'NONE', *, *, #33649, .F. ) ;
#2618=PLANE ( 'NONE',  #18949 ) ;
#2635=DIRECTION ( 'NONE',  ( 0.6600842437418872333, -0.7511915808658273797, 0.000000000000000000 ) ) ;
#2636=AXIS2_PLACEMENT_3D ( 'NONE', #93637, #31293, #8506 ) ;
#2654=CARTESIAN_POINT ( 'NONE',  ( 45.57373283677818421, 114.7827874512443032, 10.00000000000000000 ) ) ;
#2661=LINE ( 'NONE', #95900, #33993 ) ;
#2664=AXIS2_PLACEMENT_3D ( 'NONE', #33143, #39707, #70636 ) ;
#2668=DIRECTION ( 'NONE',  ( 0.000000000000000000, 0.000000000000000000, 1.000000000000000000 ) ) ;
#2679=VECTOR ( 'NONE', #28253, 1000.000000000000114 ) ;
#2687=DIRECTION ( 'NONE',  ( -0.000000000000000000, -0.000000000000000000, -1.000000000000000000 ) ) ;
#2691=FACE_OUTER_BOUND ( 'NONE', #94966, .T. ) ;
#2700=CIRCLE ( 'NONE', #77076, 70.00000000000001421 ) ;
#2703=CARTESIAN_POINT ( 'NONE',  ( -19.62743117869748843, 92.92556620904963438, 59.99999999999999289 ) ) ;
#2705=ADVANCED_FACE ( 'NONE', ( #82206 ), #95915, .T. ) ;
#2706=EDGE_LOOP ( 'NONE', ( #63491, #62939, #84124, #23159 ) ) ;
#2714=ORIENTED_EDGE ( 'NONE', *, *, #91500, .T. ) ;
#2719=CARTESIAN_POINT ( 'NONE',  ( 47.66616421796181413, 112.2513067263565034, -10.00000000000000000 ) ) ;
#2726=ORIENTED_EDGE ( 'NONE', *, *, #54440, .F. ) ;
#2735=EDGE_CURVE ( 'NONE', #18050, #9815, #68433, .T. ) ;
#2736=VERTEX_POINT ( 'NONE', #6653 ) ;
#2743=LINE ( 'NONE', #33118, #23751 ) ;
#2748=EDGE_LOOP ( 'NONE', ( #90725, #47523, #57705, #11938 ) ) ;
#2751=AXIS2_PLACEMENT_3D ( 'NONE', #2921, #42371, #87571 ) ;
#2756=ORIENTED_EDGE ( 'NONE', *, *, #1186, .T. ) ;
#2757=VECTOR ( 'NONE', #76466, 1000.000000000000227 ) ;
#2760=ADVANCED_FACE ( 'NONE', ( #38018 ), #85181, .F. ) ;
#2764=VECTOR ( 'NONE', #42700, 1000.000000000000227 ) ;
#2776=DIRECTION ( 'NONE',  ( 0.000000000000000000, 0.000000000000000000, 1.000000000000000000 ) ) ;
#2779=EDGE_CURVE ( 'NONE', #38467, #31611, #6145, .T. ) ;
#2780=CARTESIAN_POINT ( 'NONE',  ( 46.43574122514301195, 74.10519008736565638, -10.00000000000000000 ) ) ;
#2791=DIRECTION ( 'NONE',  ( -0.000000000000000000, -0.000000000000000000, 1.000000000000000000 ) ) ;
#2792=CARTESIAN_POINT ( 'NONE',  ( -17.26243516413818924, 24.35187462261285063, -10.00000000000000000 ) ) ;
#2804=LINE ( 'NONE', #8380, #56443 ) ;
#2815=CARTESIAN_POINT ( 'NONE',  ( -19.65312891409030271, 93.06504152958497400, 59.99999999999999289 ) ) ;
#2830=VECTOR ( 'NONE', #51929, 1000.000000000000114 ) ;
#2838=VECTOR ( 'NONE', #15684, 1000.000000000000114 ) ;
#2842=EDGE_LOOP ( 'NONE', ( #16526, #90745, #61506, #34235 ) ) ;
#2846=VERTEX_POINT ( 'NONE', #29446 ) ;
#2852=VECTOR ( 'NONE', #35001, 1000.000000000000114 ) ;
#2857=VERTEX_POINT ( 'NONE', #47130 ) ;
#2862=VERTEX_POINT ( 'NONE', #23828 ) ;
#2863=DIRECTION ( 'NONE',  ( 0.000000000000000000, 0.000000000000000000, 1.000000000000000000 ) ) ;
#2867=CIRCLE ( 'NONE', #61096, 70.00000000000001421 ) ;
#2882=CARTESIAN_POINT ( 'NONE',  ( -29.41917662106829212, 23.74964416229700248, -10.00000000000000000 ) ) ;
#2886=PLANE ( 'NONE',  #49661 ) ;
#2897=VECTOR ( 'NONE', #73906, 1000.000000000000000 ) ;
#2905=DIRECTION ( 'NONE',  ( -0.7299047266382377996, 0.6835488936653758563, 0.000000000000000000 ) ) ;
#2914=VECTOR ( 'NONE', #16336, 1000.000000000000227 ) ;
#2920=CARTESIAN_POINT ( 'NONE',  ( 24.41136278775235269, 63.57149826474137200, 59.99999999999999289 ) ) ;
#2921=CARTESIAN_POINT ( 'NONE',  ( 46.15481705937101964, 68.45315478587873770, -10.00000000000000000 ) ) ;
#2922=VECTOR ( 'NONE', #78983, 1000.000000000000000 ) ;
#2924=AXIS2_PLACEMENT_3D ( 'NONE', #33899, #94213, #54654 ) ;
#2929=CARTESIAN_POINT ( 'NONE',  ( -69.42519150082246426, 45.64199051378594163, -10.00000000000000000 ) ) ;
#2930=CARTESIAN_POINT ( 'NONE',  ( -19.65312891409030271, 93.06504152958497400, -10.00000000000000888 ) ) ;
#2942=DIRECTION ( 'NONE',  ( 1.000000000000000000, 0.000000000000000000, 0.000000000000000000 ) ) ;
#2944=DIRECTION ( 'NONE',  ( 0.000000000000000000, 0.000000000000000000, 1.000000000000000000 ) ) ;
#2949=CARTESIAN_POINT ( 'NONE',  ( 9.827979128326980174, 29.57595373812807082, -10.00000000000000000 ) ) ;
#2950=VERTEX_POINT ( 'NONE', #27836 ) ;
#2957=ORIENTED_EDGE ( 'NONE', *, *, #62836, .T. ) ;
#2958=PLANE ( 'NONE',  #16225 ) ;
#2964=ORIENTED_EDGE ( 'NONE', *, *, #34297, .T. ) ;
#2967=ORIENTED_EDGE ( 'NONE', *, *, #19789, .F. ) ;
#2972=DIRECTION ( 'NONE',  ( 0.000000000000000000, 0.000000000000000000, 1.000000000000000000 ) ) ;
#2985=EDGE_CURVE ( 'NONE', #25441, #81845, #6953, .T. ) ;
#2987=ORIENTED_EDGE ( 'NONE', *, *, #235, .T. ) ;
#2989=VECTOR ( 'NONE', #42260, 1000.000000000000000 ) ;
#2994=CARTESIAN_POINT ( 'NONE',  ( -15.10528209597770299, 24.46087392797018722, -10.00000000000000000 ) ) ;
#3001=ORIENTED_EDGE ( 'NONE', *, *, #87099, .F. ) ;
#3004=ORIENTED_EDGE ( 'NONE', *, *, #31411, .F. ) ;
#3006=CARTESIAN_POINT ( 'NONE',  ( 26.52232502553263416, 56.86189125829066882, 59.99999999999999289 ) ) ;
#3012=ORIENTED_EDGE ( 'NONE', *, *, #97598, .T. ) ;
#3013=VECTOR ( 'NONE', #54314, 1000.000000000000114 ) ;
#3015=EDGE_CURVE ( 'NONE', #38318, #39540, #95797, .T. ) ;
#3021=CARTESIAN_POINT ( 'NONE',  ( -77.58047734835668052, 56.02942318228900120, -10.00000000000000000 ) ) ;
#3024=VERTEX_POINT ( 'NONE', #35433 ) ;
#3030=DIRECTION ( 'NONE',  ( -0.7696402260561132636, -0.6384778167143279060, 0.000000000000000000 ) ) ;
#3031=LINE ( 'NONE', #62788, #30792 ) ;
#3042=ADVANCED_FACE ( 'NONE', ( #73947 ), #34440, .F. ) ;
#3043=AXIS2_PLACEMENT_3D ( 'NONE', #28874, #43561, #89241 ) ;
#3049=CARTESIAN_POINT ( 'NONE',  ( 34.81516168915606357, 51.10768172523390973, 10.00000000000000000 ) ) ;
#3051=DIRECTION ( 'NONE',  ( -0.7891516029629184192, 0.6141984594095433181, 0.000000000000000000 ) ) ;
#3054=VECTOR ( 'NONE', #46166, 1000.000000000000114 ) ;
#3057=ORIENTED_EDGE ( 'NONE', *, *, #68950, .F. ) ;
#3059=PLANE ( 'NONE',  #60521 ) ;
#3063=VECTOR ( 'NONE', #82068, 1000.000000000000000 ) ;
#3064=DIRECTION ( 'NONE',  ( 0.000000000000000000, 0.000000000000000000, 1.000000000000000000 ) ) ;
#3076=DIRECTION ( 'NONE',  ( -0.5369817302126890235, 0.8435938723211464652, 0.000000000000000000 ) ) ;
#3082=CARTESIAN_POINT ( 'NONE',  ( -68.10632939235270555, 44.28490124273479012, -10.00000000000000000 ) ) ;
#3096=CARTESIAN_POINT ( 'NONE',  ( -52.33464467766007289, 32.58262665401804270, -10.00000000000000000 ) ) ;
#3098=CARTESIAN_POINT ( 'NONE',  ( -46.74660806181546491, 29.87360136034011049, 10.00000000000000000 ) ) ;
#3099=ADVANCED_FACE ( 'NONE', ( #51123 ), #59201, .F. ) ;
#3101=CARTESIAN_POINT ( 'NONE',  ( -19.61423149679382050, 93.20142602126372822, 59.99999999999999289 ) ) ;
#3104=EDGE_CURVE ( 'NONE', #49232, #28990, #4036, .T. ) ;
#3108=CARTESIAN_POINT ( 'NONE',  ( -20.39262980780284096, 59.83893478986780678, -10.00000000000000000 ) ) ;
#3112=ADVANCED_FACE ( 'NONE', ( #96786 ), #58227, .F. ) ;
#3114=DIRECTION ( 'NONE',  ( -1.000000000000000000, 0.000000000000000000, 0.000000000000000000 ) ) ;
#3122=AXIS2_PLACEMENT_3D ( 'NONE', #17440, #94987, #27052 ) ;
#3124=VERTEX_POINT ( 'NONE', #72471 ) ;
#3135=LINE ( 'NONE', #34019, #15681 ) ;
#3163=CARTESIAN_POINT ( 'NONE',  ( -19.51143224695965017, 93.05905879050990848, 59.99999999999999289 ) ) ;
#3176=ORIENTED_EDGE ( 'NONE', *, *, #28774, .F. ) ;
#3212=CIRCLE ( 'NONE', #20989, 70.00000000000001421 ) ;
#3227=LINE ( 'NONE', #73120, #69319 ) ;
#3237=LINE ( 'NONE', #96450, #23493 ) ;
#3238=ORIENTED_EDGE ( 'NONE', *, *, #36089, .T. ) ;
#3240=CARTESIAN_POINT ( 'NONE',  ( 36.77241830740854311, 76.97224366495252923, 59.99999999999999289 ) ) ;
#3251=AXIS2_PLACEMENT_3D ( 'NONE', #29631, #89972, #60504 ) ;
#3252=CARTESIAN_POINT ( 'NONE',  ( 11.76667899187106059, 31.90941714274742225, -10.00000000000000000 ) ) ;
#3254=ORIENTED_EDGE ( 'NONE', *, *, #97395, .F. ) ;
#3257=PLANE ( 'NONE',  #87178 ) ;
#3258=LINE ( 'NONE', #34141, #25027 ) ;
#3259=ORIENTED_EDGE ( 'NONE', *, *, #16537, .F. ) ;
#3263=CARTESIAN_POINT ( 'NONE',  ( 50.12332653952445582, 98.65487733484057742, -10.00000000000000000 ) ) ;
#3264=DIRECTION ( 'NONE',  ( -0.000000000000000000, 0.000000000000000000, -1.000000000000000000 ) ) ;
#3266=DIRECTION ( 'NONE',  ( -1.000000000000000000, 0.000000000000000000, 0.000000000000000000 ) ) ;
#3267=AXIS2_PLACEMENT_3D ( 'NONE', #52084, #45958, #52573 ) ;
#3270=FACE_OUTER_BOUND ( 'NONE', #41973, .T. ) ;
#3279=AXIS2_PLACEMENT_3D ( 'NONE', #58574, #89547, #20108 ) ;
#3280=EDGE_CURVE ( 'NONE', #93038, #5980, #56109, .T. ) ;
#3283=ORIENTED_EDGE ( 'NONE', *, *, #54765, .T. ) ;
#3285=EDGE_CURVE ( 'NONE', #94911, #74392, #83065, .T. ) ;
#3288=DIRECTION ( 'NONE',  ( 0.8218955677251033043, 0.5696381972391160176, 0.000000000000000000 ) ) ;
#3295=EDGE_CURVE ( 'NONE', #11375, #28770, #24719, .T. ) ;
#3308=ORIENTED_EDGE ( 'NONE', *, *, #19349, .F. ) ;
#3319=ORIENTED_EDGE ( 'NONE', *, *, #5913, .F. ) ;
#3335=VECTOR ( 'NONE', #66903, 1000.000000000000000 ) ;
#3338=ORIENTED_EDGE ( 'NONE', *, *, #47099, .F. ) ;
#3345=EDGE_CURVE ( 'NONE', #1951, #44012, #85061, .T. ) ;
#3350=CARTESIAN_POINT ( 'NONE',  ( -33.52748748567718451, 62.86531959580030104, -10.00000000000000000 ) ) ;
#3357=ORIENTED_EDGE ( 'NONE', *, *, #33134, .T. ) ;
#3358=FACE_OUTER_BOUND ( 'NONE', #52409, .T. ) ;
#3359=ORIENTED_EDGE ( 'NONE', *, *, #66562, .T. ) ;
#3362=EDGE_LOOP ( 'NONE', ( #1156, #7685, #76376, #61602 ) ) ;
#3375=DIRECTION ( 'NONE',  ( -0.8321961394790213795, 0.5544813661758285495, 0.000000000000000000 ) ) ;
#3381=CARTESIAN_POINT ( 'NONE',  ( -6.542761065016642341, 25.57183462804972507, 10.00000000000000000 ) ) ;
#3390=ORIENTED_EDGE ( 'NONE', *, *, #85117, .T. ) ;
#3392=ORIENTED_EDGE ( 'NONE', *, *, #23167, .F. ) ;
#3405=DIRECTION ( 'NONE',  ( -0.8278489937552534483, 0.5609510170580086497, 0.000000000000000000 ) ) ;
#3406=LINE ( 'NONE', #89059, #22615 ) ;
#3409=CARTESIAN_POINT ( 'NONE',  ( 34.30728256194431225, 70.01911717335251240, 59.99999999999999289 ) ) ;
#3423=EDGE_CURVE ( 'NONE', #72480, #83576, #21144, .T. ) ;
#3427=EDGE_CURVE ( 'NONE', #88229, #56147, #52023, .T. ) ;
#3434=LINE ( 'NONE', #73323, #5297 ) ;
#3438=CARTESIAN_POINT ( 'NONE',  ( 47.28113444070024229, 72.57591296950350568, -10.00000000000000000 ) ) ;
#3439=ORIENTED_EDGE ( 'NONE', *, *, #65985, .T. ) ;
#3454=ORIENTED_EDGE ( 'NONE', *, *, #10699, .F. ) ;
#3457=CARTESIAN_POINT ( 'NONE',  ( -19.65312891409030271, 93.06504152958497400, -40.00000000000000000 ) ) ;
#3458=ORIENTED_EDGE ( 'NONE', *, *, #97604, .F. ) ;
#3459=FACE_OUTER_BOUND ( 'NONE', #71738, .T. ) ;
#3467=ORIENTED_EDGE ( 'NONE', *, *, #38757, .T. ) ;
#3472=DIRECTION ( 'NONE',  ( -1.000000000000000000, 0.000000000000000000, 0.000000000000000000 ) ) ;
#3473=DIRECTION ( 'NONE',  ( 0.7226656227773233798, 0.6911977992267216431, 0.000000000000000000 ) ) ;
#3474=VERTEX_POINT ( 'NONE', #51785 ) ;
#3476=VERTEX_POINT ( 'NONE', #26989 ) ;
#3481=FACE_OUTER_BOUND ( 'NONE', #69465, .T. ) ;
#3482=DIRECTION ( 'NONE',  ( 0.000000000000000000, 0.000000000000000000, 1.000000000000000000 ) ) ;
#3488=VERTEX_POINT ( 'NONE', #73591 ) ;
#3490=CARTESIAN_POINT ( 'NONE',  ( -14.15357965443277877, 60.28889183820906794, -10.00000000000000000 ) ) ;
#3495=CARTESIAN_POINT ( 'NONE',  ( 32.28746131679088904, 82.40185739040765611, 59.99999999999999289 ) ) ;
#3496=CARTESIAN_POINT ( 'NONE',  ( -19.65312891409030271, 93.06504152958497400, 177.5919119679930134 ) ) ;
#3500=ORIENTED_EDGE ( 'NONE', *, *, #30809, .T. ) ;
#3501=ORIENTED_EDGE ( 'NONE', *, *, #1428, .T. ) ;
#3502=LINE ( 'NONE', #88144, #52781 ) ;
#3503=DIRECTION ( 'NONE',  ( -0.2194785493951510180, 0.9756173257765569096, 0.000000000000000000 ) ) ;
#3505=EDGE_CURVE ( 'NONE', #66517, #65850, #29436, .T. ) ;
#3528=CARTESIAN_POINT ( 'NONE',  ( 7.411877368840288582, 73.77757239660104460, -10.00000000000000000 ) ) ;
#3529=ADVANCED_FACE ( 'NONE', ( #90323 ), #66474, .F. ) ;
#3543=CARTESIAN_POINT ( 'NONE',  ( -32.64350997085662698, 85.56504152958518716, 0.000000000000000000 ) ) ;
#3544=VERTEX_POINT ( 'NONE', #77052 ) ;
#3547=CARTESIAN_POINT ( 'NONE',  ( -50.03187330694644430, 79.58717375443625031, -10.00000000000000000 ) ) ;
#3554=DIRECTION ( 'NONE',  ( 0.7891516029629116469, -0.6141984594095518668, 0.000000000000000000 ) ) ;
#3555=CARTESIAN_POINT ( 'NONE',  ( -11.66892150670920891, 34.93507448871975640, 59.99999999999999289 ) ) ;
#3564=CARTESIAN_POINT ( 'NONE',  ( -16.79375656932349870, 82.86235307299436670, 14.77409422163848518 ) ) ;
#3570=DIRECTION ( 'NONE',  ( -0.9994626398093606756, -0.03277852384266333186, 0.000000000000000000 ) ) ;
#3586=VERTEX_POINT ( 'NONE', #78581 ) ;
#3588=DIRECTION ( 'NONE',  ( 0.1239754375649568946, 0.9922852870422788074, 0.000000000000000000 ) ) ;
#3590=ORIENTED_EDGE ( 'NONE', *, *, #39192, .F. ) ;
#3591=FACE_OUTER_BOUND ( 'NONE', #73455, .T. ) ;
#3597=DIRECTION ( 'NONE',  ( 0.000000000000000000, 0.000000000000000000, 1.000000000000000000 ) ) ;
#3600=ORIENTED_EDGE ( 'NONE', *, *, #34182, .F. ) ;
#3612=ADVANCED_FACE ( 'NONE', ( #10173 ), #32954, .F. ) ;
#3615=VERTEX_POINT ( 'NONE', #63859 ) ;
#3622=DIRECTION ( 'NONE',  ( 0.000000000000000000, 0.000000000000000000, 1.000000000000000000 ) ) ;
#3625=CARTESIAN_POINT ( 'NONE',  ( 39.25774830830064133, 55.25619937740606957, 177.5919119679930134 ) ) ;
#3627=ORIENTED_EDGE ( 'NONE', *, *, #50446, .T. ) ;
#3630=ORIENTED_EDGE ( 'NONE', *, *, #1304, .T. ) ;
#3634=CARTESIAN_POINT ( 'NONE',  ( 24.35067441160642687, 40.23626134430271861, -10.00000000000000000 ) ) ;
#3640=DIRECTION ( 'NONE',  ( -0.8082118706970125022, -0.5888918169447047157, 0.000000000000000000 ) ) ;
#3645=CARTESIAN_POINT ( 'NONE',  ( -77.42978507651396569, 55.80833764325424085, -10.00000000000000000 ) ) ;
#3651=FACE_OUTER_BOUND ( 'NONE', #3977, .T. ) ;
#3660=EDGE_CURVE ( 'NONE', #95480, #29721, #41549, .T. ) ;
#3677=FACE_OUTER_BOUND ( 'NONE', #17782, .T. ) ;
#3696=CARTESIAN_POINT ( 'NONE',  ( 26.18314342202568668, 41.82794442100486521, -10.00000000000000000 ) ) ;
#3700=VERTEX_POINT ( 'NONE', #43029 ) ;
#3705=ORIENTED_EDGE ( 'NONE', *, *, #85328, .T. ) ;
#3706=ORIENTED_EDGE ( 'NONE', *, *, #52020, .F. ) ;
#3710=ORIENTED_EDGE ( 'NONE', *, *, #70214, .T. ) ;
#3718=VECTOR ( 'NONE', #72842, 1000.000000000000114 ) ;
#3724=ORIENTED_EDGE ( 'NONE', *, *, #21888, .T. ) ;
#3727=VECTOR ( 'NONE', #91936, 1000.000000000000114 ) ;
#3728=ORIENTED_EDGE ( 'NONE', *, *, #20597, .T. ) ;
#3730=ORIENTED_EDGE ( 'NONE', *, *, #19548, .T. ) ;
#3738=LINE ( 'NONE', #9847, #43625 ) ;
#3741=VECTOR ( 'NONE', #88105, 1000.000000000000227 ) ;
#3742=VERTEX_POINT ( 'NONE', #57247 ) ;
#3748=ORIENTED_EDGE ( 'NONE', *, *, #81477, .T. ) ;
#3751=CARTESIAN_POINT ( 'NONE',  ( -15.23834836788960345, 40.22511121182390070, 59.99999999999999289 ) ) ;
#3755=ORIENTED_EDGE ( 'NONE', *, *, #56258, .T. ) ;
#3756=CARTESIAN_POINT ( 'NONE',  ( -44.49648453423614569, 28.96346851210257967, 10.00000000000000000 ) ) ;
#3757=LINE ( 'NONE', #87431, #80368 ) ;
#3767=ORIENTED_EDGE ( 'NONE', *, *, #10271, .T. ) ;
#3774=LINE ( 'NONE', #34656, #25549 ) ;
#3780=ADVANCED_FACE ( 'NONE', ( #12678 ), #11679, .T. ) ;
#3788=DIRECTION ( 'NONE',  ( -0.8660254037844379305, -0.5000000000000012212, 0.000000000000000000 ) ) ;
#3800=AXIS2_PLACEMENT_3D ( 'NONE', #52280, #74112, #5685 ) ;
#3810=ORIENTED_EDGE ( 'NONE', *, *, #20842, .F. ) ;
#3818=CARTESIAN_POINT ( 'NONE',  ( -69.42519150082246426, 45.64199051378594874, -10.00000000000000000 ) ) ;
#3829=ORIENTED_EDGE ( 'NONE', *, *, #24300, .T. ) ;
#3834=VERTEX_POINT ( 'NONE', #59223 ) ;
#3835=EDGE_LOOP ( 'NONE', ( #34684, #69097, #31191, #76041 ) ) ;
#3839=ORIENTED_EDGE ( 'NONE', *, *, #3660, .T. ) ;
#3849=EDGE_CURVE ( 'NONE', #92132, #44698, #74487, .T. ) ;
#3850=DIRECTION ( 'NONE',  ( -1.000000000000000000, 0.000000000000000000, 0.000000000000000000 ) ) ;
#3871=PLANE ( 'NONE',  #32203 ) ;
#3872=VECTOR ( 'NONE', #44525, 1000.000000000000000 ) ;
#3875=DIRECTION ( 'NONE',  ( 0.000000000000000000, -0.000000000000000000, 1.000000000000000000 ) ) ;
#3880=ORIENTED_EDGE ( 'NONE', *, *, #37565, .F. ) ;
#3885=EDGE_CURVE ( 'NONE', #5196, #29361, #26371, .T. ) ;
#3889=DIRECTION ( 'NONE',  ( 0.4174706225611858335, 0.9086904199442051855, 0.000000000000000000 ) ) ;
#3895=LINE ( 'NONE', #66191, #27036 ) ;
#3896=ADVANCED_FACE ( 'NONE', ( #19777 ), #81598, .F. ) ;
#3901=ADVANCED_FACE ( 'NONE', ( #42540 ), #89709, .F. ) ;
#3902=PLANE ( 'NONE',  #60450 ) ;
#3936=LINE ( 'NONE', #34820, #40234 ) ;
#3937=AXIS2_PLACEMENT_3D ( 'NONE', #78855, #34236, #40312 ) ;
#3947=EDGE_CURVE ( 'NONE', #81604, #81790, #65843, .T. ) ;
#3951=EDGE_LOOP ( 'NONE', ( #33969, #81656, #68752, #43358 ) ) ;
#3957=FACE_OUTER_BOUND ( 'NONE', #84294, .T. ) ;
#3960=ADVANCED_FACE ( 'NONE', ( #6050 ), #76936, .F. ) ;
#3965=PLANE ( 'NONE',  #39871 ) ;
#3967=EDGE_LOOP ( 'NONE', ( #15948, #54520, #89344, #74308 ) ) ;
#3968=ORIENTED_EDGE ( 'NONE', *, *, #86274, .T. ) ;
#3970=EDGE_CURVE ( 'NONE', #3742, #55035, #84588, .T. ) ;
#3977=EDGE_LOOP ( 'NONE', ( #212, #97501, #20928, #87142 ) ) ;
#3979=DIRECTION ( 'NONE',  ( 0.001368469433193686413, -0.9999990636452668058, 0.000000000000000000 ) ) ;
#3987=PLANE ( 'NONE',  #38159 ) ;
#3988=VERTEX_POINT ( 'NONE', #99759 ) ;
#3995=DIRECTION ( 'NONE',  ( -0.6384778167143279060, 0.7696402260561132636, 0.000000000000000000 ) ) ;
#3996=VECTOR ( 'NONE', #17041, 1000.000000000000000 ) ;
#3998=FACE_OUTER_BOUND ( 'NONE', #36994, .T. ) ;
#4015=FACE_OUTER_BOUND ( 'NONE', #9926, .T. ) ;
#4020=VERTEX_POINT ( 'NONE', #62729 ) ;
#4031=CARTESIAN_POINT ( 'NONE',  ( -19.65312891409030271, 93.06504152958497400, 10.00000000000000888 ) ) ;
#4033=CARTESIAN_POINT ( 'NONE',  ( 49.60098510475376088, 81.22027839155747131, -10.00000000000000000 ) ) ;
#4036=LINE ( 'NONE', #42518, #63572 ) ;
#4044=ORIENTED_EDGE ( 'NONE', *, *, #30539, .T. ) ;
#4061=AXIS2_PLACEMENT_3D ( 'NONE', #25282, #39460, #38476 ) ;
#4063=ORIENTED_EDGE ( 'NONE', *, *, #44174, .T. ) ;
#4084=CARTESIAN_POINT ( 'NONE',  ( 4.102725850843912170, 28.55253618238880620, -10.00000000000000000 ) ) ;
#4090=DIRECTION ( 'NONE',  ( -0.6118251767726360368, -0.7909930170786165782, 0.000000000000000000 ) ) ;
#4099=AXIS2_PLACEMENT_3D ( 'NONE', #57184, #65298, #72931 ) ;
#4101=LINE ( 'NONE', #42585, #97868 ) ;
#4107=LINE ( 'NONE', #11242, #86991 ) ;
#4108=CYLINDRICAL_SURFACE ( 'NONE', #34382, 70.00000000000002842 ) ;
#4111=LINE ( 'NONE', #34517, #59913 ) ;
#4113=DIRECTION ( 'NONE',  ( 0.000000000000000000, 0.000000000000000000, 1.000000000000000000 ) ) ;
#4114=EDGE_CURVE ( 'NONE', #27521, #91230, #81373, .T. ) ;
#4120=EDGE_CURVE ( 'NONE', #71865, #16478, #89479, .T. ) ;
#4126=LINE ( 'NONE', #58320, #14331 ) ;
#4128=VECTOR ( 'NONE', #100066, 999.9999999999998863 ) ;
#4162=DIRECTION ( 'NONE',  ( 0.3956464567955563782, -0.9184028970038813355, 0.000000000000000000 ) ) ;
#4167=DIRECTION ( 'NONE',  ( -0.9404163354663408469, -0.3400251696390411693, 0.000000000000000000 ) ) ;
#4169=ORIENTED_EDGE ( 'NONE', *, *, #82733, .T. ) ;
#4173=EDGE_LOOP ( 'NONE', ( #29992, #27784, #33502, #3705 ) ) ;
#4176=VECTOR ( 'NONE', #60511, 1000.000000000000114 ) ;
#4187=ORIENTED_EDGE ( 'NONE', *, *, #45619, .F. ) ;
#4191=CARTESIAN_POINT ( 'NONE',  ( -20.65464553008482795, 23.07220643578491348, -10.00000000000000000 ) ) ;
#4195=AXIS2_PLACEMENT_3D ( 'NONE', #61422, #43731, #14827 ) ;
#4200=ORIENTED_EDGE ( 'NONE', *, *, #25640, .T. ) ;
#4203=AXIS2_PLACEMENT_3D ( 'NONE', #59932, #69539, #30546 ) ;
#4206=DIRECTION ( 'NONE',  ( 0.000000000000000000, 0.000000000000000000, 1.000000000000000000 ) ) ;
#4207=ORIENTED_EDGE ( 'NONE', *, *, #74300, .T. ) ;
#4217=CARTESIAN_POINT ( 'NONE',  ( -49.78034631855286563, 29.87998972566340683, -10.00000000000000000 ) ) ;
#4221=VERTEX_POINT ( 'NONE', #32091 ) ;
#4223=DIRECTION ( 'NONE',  ( 0.3301025504114333264, 0.9439450758449176027, 0.000000000000000000 ) ) ;
#4225=CARTESIAN_POINT ( 'NONE',  ( -71.36129514276957764, 45.88172302328153052, 177.5919119679930134 ) ) ;
#4229=CARTESIAN_POINT ( 'NONE',  ( 49.32130651720206771, 81.12656353050643077, -10.00000000000000000 ) ) ;
#4231=EDGE_CURVE ( 'NONE', #37455, #58141, #39673, .T. ) ;
#4244=AXIS2_PLACEMENT_3D ( 'NONE', #91472, #22034, #14922 ) ;
#4249=VECTOR ( 'NONE', #2008, 1000.000000000000227 ) ;
#4258=EDGE_LOOP ( 'NONE', ( #49715, #3500, #95242, #1937 ) ) ;
#4259=DIRECTION ( 'NONE',  ( 0.7033187449715098127, -0.7108746323872447981, 0.000000000000000000 ) ) ;
#4268=DIRECTION ( 'NONE',  ( 0.4270171210482451851, -0.9042435392811322137, 0.000000000000000000 ) ) ;
#4272=ORIENTED_EDGE ( 'NONE', *, *, #33511, .T. ) ;
#4274=CARTESIAN_POINT ( 'NONE',  ( -19.65312891409030271, 93.06504152958497400, 177.5919119679930134 ) ) ;
#4278=DIRECTION ( 'NONE',  ( 0.000000000000000000, 0.000000000000000000, 1.000000000000000000 ) ) ;
#4283=VERTEX_POINT ( 'NONE', #58754 ) ;
#4286=LINE ( 'NONE', #73212, #52296 ) ;
#4299=DIRECTION ( 'NONE',  ( -0.3668518372888711077, -0.9302793824855948301, 0.000000000000000000 ) ) ;
#4302=ORIENTED_EDGE ( 'NONE', *, *, #72790, .F. ) ;
#4312=ORIENTED_EDGE ( 'NONE', *, *, #48937, .T. ) ;
#4319=ORIENTED_EDGE ( 'NONE', *, *, #43064, .F. ) ;
#4321=VERTEX_POINT ( 'NONE', #10318 ) ;
#4322=EDGE_CURVE ( 'NONE', #84216, #33383, #64004, .T. ) ;
#4324=CIRCLE ( 'NONE', #15581, 0.1418229129681522482 ) ;
#4326=DIRECTION ( 'NONE',  ( -0.000000000000000000, -0.000000000000000000, -1.000000000000000000 ) ) ;
#4328=ORIENTED_EDGE ( 'NONE', *, *, #36213, .T. ) ;
#4329=ADVANCED_FACE ( 'NONE', ( #33106 ), #81615, .F. ) ;
#4338=DIRECTION ( 'NONE',  ( -0.3077152132536331575, -0.9514785060800222682, 0.000000000000000000 ) ) ;
#4344=ORIENTED_EDGE ( 'NONE', *, *, #1379, .T. ) ;
#4345=DIRECTION ( 'NONE',  ( -0.5544813661758285495, -0.8321961394790213795, 0.000000000000000000 ) ) ;
#4346=ORIENTED_EDGE ( 'NONE', *, *, #1707, .T. ) ;
#4350=CIRCLE ( 'NONE', #36730, 70.00000000000001421 ) ;
#4362=ORIENTED_EDGE ( 'NONE', *, *, #83987, .T. ) ;
#4365=CARTESIAN_POINT ( 'NONE',  ( 37.44155836008122407, 106.5941701475231724, 59.99999999999999289 ) ) ;
#4367=CARTESIAN_POINT ( 'NONE',  ( 49.54000814145099696, 103.6626726051169527, -10.00000000000000000 ) ) ;
#4371=VERTEX_POINT ( 'NONE', #72124 ) ;
#4373=LINE ( 'NONE', #35272, #92151 ) ;
#4385=AXIS2_PLACEMENT_3D ( 'NONE', #5734, #75645, #98459 ) ;
#4394=EDGE_CURVE ( 'NONE', #28770, #40778, #52157, .T. ) ;
#4395=VECTOR ( 'NONE', #97820, 1000.000000000000227 ) ;
#4409=CYLINDRICAL_SURFACE ( 'NONE', #40994, 70.00000000000002842 ) ;
#4412=CIRCLE ( 'NONE', #95072, 11.91750000000000043 ) ;
#4414=CARTESIAN_POINT ( 'NONE',  ( -52.87923565380747704, 93.80454242329714987, -10.00000000000000000 ) ) ;
#4423=VECTOR ( 'NONE', #44882, 1000.000000000000114 ) ;
#4429=VERTEX_POINT ( 'NONE', #53157 ) ;
#4431=ORIENTED_EDGE ( 'NONE', *, *, #95511, .T. ) ;
#4441=LINE ( 'NONE', #59619, #74054 ) ;
#4445=CARTESIAN_POINT ( 'NONE',  ( 42.33744422746375591, 122.7866300363639169, -10.00000000000000000 ) ) ;
#4456=LINE ( 'NONE', #66264, #87262 ) ;
#4461=DIRECTION ( 'NONE',  ( 1.000000000000000000, 0.000000000000000000, 0.000000000000000000 ) ) ;
#4465=AXIS2_PLACEMENT_3D ( 'NONE', #63752, #73361, #41946 ) ;
#4474=ORIENTED_EDGE ( 'NONE', *, *, #48621, .F. ) ;
#4478=ORIENTED_EDGE ( 'NONE', *, *, #94253, .F. ) ;
#4484=LINE ( 'NONE', #74901, #51114 ) ;
#4494=DIRECTION ( 'NONE',  ( -0.000000000000000000, -0.000000000000000000, -1.000000000000000000 ) ) ;
#4496=VECTOR ( 'NONE', #18224, 1000.000000000000114 ) ;
#4501=ADVANCED_FACE ( 'NONE', ( #73368 ), #59630, .F. ) ;
#4506=CARTESIAN_POINT ( 'NONE',  ( -19.75907871001397353, 92.97076332750987149, 59.99999999999999289 ) ) ;
#4511=ORIENTED_EDGE ( 'NONE', *, *, #77236, .T. ) ;
#4529=LINE ( 'NONE', #14131, #47689 ) ;
#4530=VECTOR ( 'NONE', #20222, 1000.000000000000114 ) ;
#4533=DIRECTION ( 'NONE',  ( 1.000000000000000000, 0.000000000000000000, 0.000000000000000000 ) ) ;
#4538=CARTESIAN_POINT ( 'NONE',  ( -6.649575753788274923, 83.58322560409861524, 13.50909007041568621 ) ) ;
#4550=ADVANCED_FACE ( 'NONE', ( #3481 ), #82511, .T. ) ;
#4552=CARTESIAN_POINT ( 'NONE',  ( -16.10531488956837975, 22.89493580087430402, -10.00000000000000000 ) ) ;
#4555=EDGE_CURVE ( 'NONE', #39135, #93866, #4967, .T. ) ;
#4560=VERTEX_POINT ( 'NONE', #74873 ) ;
#4561=VERTEX_POINT ( 'NONE', #5455 ) ;
#4563=VECTOR ( 'NONE', #36815, 1000.000000000000227 ) ;
#4565=DIRECTION ( 'NONE',  ( 1.000000000000000000, 0.000000000000000000, 0.000000000000000000 ) ) ;
#4567=ORIENTED_EDGE ( 'NONE', *, *, #30771, .F. ) ;
#4583=EDGE_CURVE ( 'NONE', #11342, #55246, #5949, .T. ) ;
#4584=FACE_BOUND ( 'NONE', #53871, .T. ) ;
#4596=AXIS2_PLACEMENT_3D ( 'NONE', #87904, #48846, #2248 ) ;
#4597=ORIENTED_EDGE ( 'NONE', *, *, #25713, .F. ) ;
#4599=DIRECTION ( 'NONE',  ( -0.000000000000000000, 0.000000000000000000, -1.000000000000000000 ) ) ;
#4605=VECTOR ( 'NONE', #31513, 1000.000000000000227 ) ;
#4608=CARTESIAN_POINT ( 'NONE',  ( -23.47208873469913115, 24.42380372261332155, 10.00000000000000000 ) ) ;
#4610=VECTOR ( 'NONE', #92711, 999.9999999999998863 ) ;
#4625=CARTESIAN_POINT ( 'NONE',  ( 1.023347710557717782, 26.18841396516313935, 177.5919119679930134 ) ) ;
#4641=VERTEX_POINT ( 'NONE', #69732 ) ;
#4643=PLANE ( 'NONE',  #42733 ) ;
#4664=AXIS2_PLACEMENT_3D ( 'NONE', #7336, #78258, #23523 ) ;
#4670=AXIS2_PLACEMENT_3D ( 'NONE', #92154, #70284, #895 ) ;
#4672=LINE ( 'NONE', #49771, #7671 ) ;
#4688=EDGE_LOOP ( 'NONE', ( #46285, #11240, #56332, #33994 ) ) ;
#4690=CARTESIAN_POINT ( 'NONE',  ( 1.813001633210440611, 27.74720351945397923, 10.00000000000000000 ) ) ;
#4691=DIRECTION ( 'NONE',  ( 0.9598361373656965068, -0.2805612043866717031, 0.000000000000000000 ) ) ;
#4693=ORIENTED_EDGE ( 'NONE', *, *, #39398, .T. ) ;
#4694=CIRCLE ( 'NONE', #61360, 70.00000000000001421 ) ;
#4695=ORIENTED_EDGE ( 'NONE', *, *, #22610, .F. ) ;
#4698=DIRECTION ( 'NONE',  ( -0.000000000000000000, -0.000000000000000000, -1.000000000000000000 ) ) ;
#4700=ORIENTED_EDGE ( 'NONE', *, *, #31697, .F. ) ;
#4709=AXIS2_PLACEMENT_3D ( 'NONE', #93260, #47616, #9650 ) ;
#4718=EDGE_CURVE ( 'NONE', #53015, #66626, #47739, .T. ) ;
#4722=ORIENTED_EDGE ( 'NONE', *, *, #83014, .T. ) ;
#4723=CARTESIAN_POINT ( 'NONE',  ( 47.89168550319195106, 74.68847913791599069, 177.5919119679930134 ) ) ;
#4732=DIRECTION ( 'NONE',  ( -1.000000000000000000, 0.000000000000000000, 0.000000000000000000 ) ) ;
#4749=ORIENTED_EDGE ( 'NONE', *, *, #8795, .F. ) ;
#4765=VECTOR ( 'NONE', #49586, 1000.000000000000000 ) ;
#4773=LINE ( 'NONE', #43740, #22282 ) ;
#4778=ORIENTED_EDGE ( 'NONE', *, *, #86915, .T. ) ;
#4782=CIRCLE ( 'NONE', #33870, 0.1418229129683812317 ) ;
#4802=DIRECTION ( 'NONE',  ( 0.5344452582589497291, -0.8452030915256549815, 0.000000000000000000 ) ) ;
#4803=PLANE ( 'NONE',  #19375 ) ;
#4815=LINE ( 'NONE', #60466, #61975 ) ;
#4829=ORIENTED_EDGE ( 'NONE', *, *, #29214, .T. ) ;
#4831=DIRECTION ( 'NONE',  ( -0.8261602328994366307, 0.5634352399127593447, 0.000000000000000000 ) ) ;
#4837=AXIS2_PLACEMENT_3D ( 'NONE', #12393, #43258, #25589 ) ;
#4842=ORIENTED_EDGE ( 'NONE', *, *, #83291, .T. ) ;
#4848=ORIENTED_EDGE ( 'NONE', *, *, #72790, .T. ) ;
#4849=DIRECTION ( 'NONE',  ( 0.000000000000000000, -0.000000000000000000, -1.000000000000000000 ) ) ;
#4859=ORIENTED_EDGE ( 'NONE', *, *, #65273, .T. ) ;
#4864=VECTOR ( 'NONE', #2325, 1000.000000000000000 ) ;
#4872=CARTESIAN_POINT ( 'NONE',  ( -58.62427208439002158, 70.56504152958493137, 60.00000000000000000 ) ) ;
#4878=ORIENTED_EDGE ( 'NONE', *, *, #87099, .T. ) ;
#4881=CARTESIAN_POINT ( 'NONE',  ( -44.49648453423614569, 28.96346851210257967, -10.00000000000000000 ) ) ;
#4884=DIRECTION ( 'NONE',  ( 0.000000000000000000, 0.000000000000000000, 1.000000000000000000 ) ) ;
#4886=CARTESIAN_POINT ( 'NONE',  ( -62.83817737799399339, 37.97373922903764765, -10.00000000000000000 ) ) ;
#4892=DIRECTION ( 'NONE',  ( -0.000000000000000000, 0.000000000000000000, 1.000000000000000000 ) ) ;
#4912=ADVANCED_FACE ( 'NONE', ( #17225 ), #93268, .F. ) ;
#4913=AXIS2_PLACEMENT_3D ( 'NONE', #28402, #73530, #59282 ) ;
#4926=DIRECTION ( 'NONE',  ( -0.8614378286617561109, 0.5078630399532132467, 0.000000000000000000 ) ) ;
#4932=LINE ( 'NONE', #97159, #57192 ) ;
#4934=DIRECTION ( 'NONE',  ( 0.000000000000000000, 0.000000000000000000, 1.000000000000000000 ) ) ;
#4940=PLANE ( 'NONE',  #16114 ) ;
#4951=ORIENTED_EDGE ( 'NONE', *, *, #55441, .T. ) ;
#4962=ORIENTED_EDGE ( 'NONE', *, *, #29227, .F. ) ;
#4967=LINE ( 'NONE', #13073, #27917 ) ;
#4971=LINE ( 'NONE', #65258, #66283 ) ;
#4975=EDGE_LOOP ( 'NONE', ( #44909, #6067, #30840, #99599 ) ) ;
#4979=EDGE_CURVE ( 'NONE', #83740, #81604, #80585, .T. ) ;
#4981=ORIENTED_EDGE ( 'NONE', *, *, #97350, .F. ) ;
#4987=ORIENTED_EDGE ( 'NONE', *, *, #85853, .T. ) ;
#4988=AXIS2_PLACEMENT_3D ( 'NONE', #91943, #14883, #84338 ) ;
#4989=DIRECTION ( 'NONE',  ( 0.9291732088853837945, -0.3696446237802449297, 0.000000000000000000 ) ) ;
#4999=CARTESIAN_POINT ( 'NONE',  ( -62.95439910331221256, 68.06504152958493137, -20.00000000000000355 ) ) ;
#5008=CARTESIAN_POINT ( 'NONE',  ( -38.61298035630893111, 26.97617139035147460, -10.00000000000000000 ) ) ;
#5015=LINE ( 'NONE', #6000, #85432 ) ;
#5020=DIRECTION ( 'NONE',  ( 0.000000000000000000, 0.000000000000000000, 1.000000000000000000 ) ) ;
#5021=FACE_OUTER_BOUND ( 'NONE', #87155, .T. ) ;
#5025=VERTEX_POINT ( 'NONE', #96782 ) ;
#5028=CARTESIAN_POINT ( 'NONE',  ( 50.13870555935886841, 87.67061469898740711, 10.00000000000000000 ) ) ;
#5042=VECTOR ( 'NONE', #77082, 1000.000000000000000 ) ;
#5045=DIRECTION ( 'NONE',  ( 0.5607300124661794838, -0.8279987035736700030, 0.000000000000000000 ) ) ;
#5049=EDGE_LOOP ( 'NONE', ( #58869, #15624, #55007, #64286, #86903, #68242, #98636, #58129, #90068, #85847, #45803, #93430, #43793, #27597, #77616, #11333, #80130, #85501, #94732, #86887, #63105, #49953, #7048, #32473, #18175, #3012, #61368, #41291, #41332, #44445, #2987, #6249, #53388, #61150, #57126, #46852, #86351, #63422, #35026, #97672, #85968, #36179, #77643, #93211, #86414, #97596, #47092, #44156, #18159, #84786, #47947, #30373, #98782, #38835, #91106, #42666, #69576, #70660, #17799, #87660, #58903, #77066, #42670, #39040, #80089, #61255, #65096, #88362, #2078, #17053, #71113, #35367, #83210, #29392, #46160, #30103, #70263, #91549, #11976, #26677, #62257, #4848, #22370, #16521, #56477, #2957, #94570, #62755, #40026, #15631, #5555, #35242, #20533, #59528, #24128, #18786, #72152, #5842, #69227, #37495, #3359, #68323, #48970, #26879, #32118, #71984, #10946, #73522, #92940, #96534, #17960, #15418, #16627, #22465, #92339, #79532, #14303, #64292, #37804, #31203, #28758, #63599, #81469, #88773, #9834, #65501, #78203, #86331, #53738, #11320, #96670, #53141, #35098, #43915, #74995, #28221, #4272, #25915, #10815, #2578, #95581, #19916, #77730, #92936, #39438, #49531, #43694, #44669, #2070, #16907, #41415, #27990, #65868, #48319, #15672, #20295, #6578, #13156, #89616, #51405, #67267, #38478, #86479, #39633, #69490, #88384, #60995, #33243, #20694, #38413, #69828, #4842, #71861, #38066, #39455, #77951, #82820, #16498, #81107, #38579, #24241, #89135, #706, #15393, #12149, #59601, #96220, #20050, #42411, #63513, #90855, #46289, #12394, #72729, #41700, #50520, #55494, #50307, #70607, #60758, #75018, #6321, #55114, #12732, #67862, #97072, #34576, #60626, #64323, #77977, #6320, #4431, #56890, #12834, #73873, #40430, #52902, #90073, #14904, #676, #561, #70603, #45313, #75606, #4044, #21011, #85348, #47908, #72130, #59404, #57601, #52279, #19690, #15060, #77075, #66665, #56995, #68377, #2964, #18190, #33218, #57881, #20794, #97488, #11917, #97157, #65043, #47157, #85238, #44783, #58854, #18659, #83121, #96426, #43296, #47077, #14026, #34970, #84761, #26174, #88728, #95014, #97806, #93088, #95489, #79350, #69592, #40567, #71116, #4344, #21145, #55149, #2393, #43471, #86977, #45290, #14183, #72901, #64397, #94548, #67648, #30882, #47817, #3724, #97216, #87796, #21541, #17878, #60715, #31320, #37801, #13317, #8548, #65342, #8791, #48807, #32369, #83075, #23132, #78712, #35254, #30008, #14209, #66963, #97212, #35463, #16757, #58644, #84892, #99400, #88865, #48043, #76384, #43109, #17949, #97407, #60774, #9878, #32242, #52842, #35842, #34953, #4346, #99004, #56250, #49572, #87019, #22936, #3839, #92980, #22138, #85378, #8431, #16296, #12562, #83401, #67138, #74892, #71250, #37726, #31710, #53146, #52759, #11224, #46087, #94352, #30237, #16648, #91493, #32474, #54198, #91759, #41213, #71891, #43230, #83092, #24622, #37579, #12049, #35504, #75453, #58033, #63625, #56143, #16193, #20790, #87885, #91297, #91970, #85120, #51562, #25639, #29614, #7254, #72129, #64348, #61001, #39408, #64744, #70857, #61466, #60231, #56903, #21977, #12125, #32095, #47302, #65621, #70091, #797, #35092, #68360, #47789, #65134, #36132, #58508, #16513, #26067, #28209, #58772, #55120, #42767, #97757, #42589 ) ) ;
#5053=VERTEX_POINT ( 'NONE', #54471 ) ;
#5068=LINE ( 'NONE', #82110, #66204 ) ;
#5073=CARTESIAN_POINT ( 'NONE',  ( -43.51495119940489786, 40.26192753957666071, 59.99999999999999289 ) ) ;
#5081=DIRECTION ( 'NONE',  ( 1.000000000000000000, 0.000000000000000000, 0.000000000000000000 ) ) ;
#5083=EDGE_CURVE ( 'NONE', #42705, #26065, #44511, .T. ) ;
#5085=FACE_OUTER_BOUND ( 'NONE', #8579, .T. ) ;
#5086=VERTEX_POINT ( 'NONE', #70184 ) ;
#5087=ORIENTED_EDGE ( 'NONE', *, *, #12355, .T. ) ;
#5091=DIRECTION ( 'NONE',  ( -0.9292718480896766664, -0.3693965786901617365, 0.000000000000000000 ) ) ;
#5100=DIRECTION ( 'NONE',  ( 0.9331105242498740626, -0.3595896960900372696, 0.000000000000000000 ) ) ;
#5101=ORIENTED_EDGE ( 'NONE', *, *, #85291, .F. ) ;
#5106=LINE ( 'NONE', #90246, #57535 ) ;
#5123=LINE ( 'NONE', #19356, #38137 ) ;
#5124=LINE ( 'NONE', #4625, #21708 ) ;
#5130=ADVANCED_FACE ( 'NONE', ( #10411 ), #18514, .F. ) ;
#5131=EDGE_CURVE ( 'NONE', #93052, #53210, #64100, .T. ) ;
#5138=EDGE_CURVE ( 'NONE', #71477, #84728, #71726, .T. ) ;
#5170=DIRECTION ( 'NONE',  ( 1.000000000000000000, 0.000000000000000000, 0.000000000000000000 ) ) ;
#5175=DIRECTION ( 'NONE',  ( -0.3400251696390411693, 0.9404163354663408469, 0.000000000000000000 ) ) ;
#5178=CYLINDRICAL_SURFACE ( 'NONE', #33397, 70.00000000000002842 ) ;
#5182=DIRECTION ( 'NONE',  ( 0.5076330711061761702, -0.8615733660689098850, 0.000000000000000000 ) ) ;
#5196=VERTEX_POINT ( 'NONE', #47878 ) ;
#5199=EDGE_CURVE ( 'NONE', #98479, #69834, #1810, .T. ) ;
#5210=ORIENTED_EDGE ( 'NONE', *, *, #44566, .F. ) ;
#5217=CARTESIAN_POINT ( 'NONE',  ( 50.27371054362191671, 89.86549102125590593, 177.5919119679930134 ) ) ;
#5223=EDGE_LOOP ( 'NONE', ( #62211, #68488, #6769, #86872 ) ) ;
#5230=LINE ( 'NONE', #51308, #85225 ) ;
#5235=CARTESIAN_POINT ( 'NONE',  ( 20.67738335769525904, 35.85097175740956743, -10.00000000000000000 ) ) ;
#5236=EDGE_CURVE ( 'NONE', #30076, #24137, #68083, .T. ) ;
#5251=CARTESIAN_POINT ( 'NONE',  ( -1.087500518889665591, 25.57194971796827332, 10.00000000000000000 ) ) ;
#5252=ORIENTED_EDGE ( 'NONE', *, *, #63640, .T. ) ;
#5273=DIRECTION ( 'NONE',  ( 0.8325133752583725455, -0.5540049458406594018, 0.000000000000000000 ) ) ;
#5281=ORIENTED_EDGE ( 'NONE', *, *, #98009, .T. ) ;
#5290=LINE ( 'NONE', #92902, #43565 ) ;
#5297=VECTOR ( 'NONE', #57094, 1000.000000000000114 ) ;
#5302=AXIS2_PLACEMENT_3D ( 'NONE', #96695, #34356, #90092 ) ;
#5309=PLANE ( 'NONE',  #88938 ) ;
#5314=PLANE ( 'NONE',  #82263 ) ;
#5317=CARTESIAN_POINT ( 'NONE',  ( 22.96769398916923421, 37.53608102203548214, 177.5919119679930134 ) ) ;
#5322=VECTOR ( 'NONE', #87299, 1000.000000000000000 ) ;
#5330=ORIENTED_EDGE ( 'NONE', *, *, #25246, .T. ) ;
#5331=ORIENTED_EDGE ( 'NONE', *, *, #32346, .T. ) ;
#5333=VERTEX_POINT ( 'NONE', #7784 ) ;
#5335=VERTEX_POINT ( 'NONE', #185 ) ;
#5338=ORIENTED_EDGE ( 'NONE', *, *, #13491, .F. ) ;
#5342=EDGE_CURVE ( 'NONE', #20462, #79982, #38157, .T. ) ;
#5345=VERTEX_POINT ( 'NONE', #78193 ) ;
#5348=VERTEX_POINT ( 'NONE', #14395 ) ;
#5358=CARTESIAN_POINT ( 'NONE',  ( -74.97640825042664403, 52.25402898078436920, 10.00000000000000000 ) ) ;
#5359=ADVANCED_FACE ( 'NONE', ( #41665 ), #48796, .T. ) ;
#5362=VERTEX_POINT ( 'NONE', #79727 ) ;
#5368=LINE ( 'NONE', #67154, #61137 ) ;
#5381=DIRECTION ( 'NONE',  ( 0.1237105541964823863, -0.9923183454821336014, 0.000000000000000000 ) ) ;
#5383=DIRECTION ( 'NONE',  ( 0.000000000000000000, 0.000000000000000000, 1.000000000000000000 ) ) ;
#5384=EDGE_CURVE ( 'NONE', #72718, #30899, #63974, .T. ) ;
#5391=ADVANCED_FACE ( 'NONE', ( #94917 ), #95931, .F. ) ;
#5400=CARTESIAN_POINT ( 'NONE',  ( -19.51131409799570093, 93.06655697632794499, 59.99999999999999289 ) ) ;
#5403=CARTESIAN_POINT ( 'NONE',  ( -36.83782344121361518, 37.72751643289125667, 59.99999999999999289 ) ) ;
#5427=CARTESIAN_POINT ( 'NONE',  ( -22.85267942241863537, 23.13820207187275457, 177.5919119679930134 ) ) ;
#5443=FACE_OUTER_BOUND ( 'NONE', #92756, .T. ) ;
#5444=AXIS2_PLACEMENT_3D ( 'NONE', #29706, #59589, #36800 ) ;
#5447=CARTESIAN_POINT ( 'NONE',  ( -65.03992292888628413, 39.77302590755693501, 10.00000000000000000 ) ) ;
#5455=CARTESIAN_POINT ( 'NONE',  ( 43.53831125515428369, 65.97156238185917232, -10.00000000000000000 ) ) ;
#5461=VECTOR ( 'NONE', #57892, 1000.000000000000114 ) ;
#5467=VERTEX_POINT ( 'NONE', #89811 ) ;
#5475=EDGE_LOOP ( 'NONE', ( #81507, #2444, #12685, #36000 ) ) ;
#5476=ADVANCED_FACE ( 'NONE', ( #5664 ), #50761, .F. ) ;
#5478=FACE_OUTER_BOUND ( 'NONE', #2583, .T. ) ;
#5483=CARTESIAN_POINT ( 'NONE',  ( 40.70814378237798081, 60.14496435084704018, 10.00000000000000000 ) ) ;
#5486=DIRECTION ( 'NONE',  ( -0.7061384650677096086, -0.7080737730998225565, 0.000000000000000000 ) ) ;
#5487=ORIENTED_EDGE ( 'NONE', *, *, #80178, .F. ) ;
#5489=FACE_OUTER_BOUND ( 'NONE', #68693, .T. ) ;
#5492=DIRECTION ( 'NONE',  ( 0.000000000000000000, 0.000000000000000000, 1.000000000000000000 ) ) ;
#5497=ADVANCED_FACE ( 'NONE', ( #12287 ), #73103, .F. ) ;
#5501=CYLINDRICAL_SURFACE ( 'NONE', #49922, 70.00000000000002842 ) ;
#5503=APPLICATION_CONTEXT ( 'automotive_design' ) ;
#5506=DIRECTION ( 'NONE',  ( -0.000000000000000000, 0.000000000000000000, -1.000000000000000000 ) ) ;
#5513=AXIS2_PLACEMENT_3D ( 'NONE', #83597, #74495, #67864 ) ;
#5517=LINE ( 'NONE', #29319, #62180 ) ;
#5521=EDGE_CURVE ( 'NONE', #36208, #25628, #92677, .T. ) ;
#5533=LINE ( 'NONE', #28837, #72022 ) ;
#5546=CARTESIAN_POINT ( 'NONE',  ( 47.92671612011951510, 80.40884667711614497, 10.00000000000000000 ) ) ;
#5550=EDGE_LOOP ( 'NONE', ( #85454, #64015, #22018, #26631 ) ) ;
#5555=ORIENTED_EDGE ( 'NONE', *, *, #82689, .T. ) ;
#5559=ORIENTED_EDGE ( 'NONE', *, *, #81366, .T. ) ;
#5561=DIRECTION ( 'NONE',  ( 0.000000000000000000, 0.000000000000000000, 1.000000000000000000 ) ) ;
#5571=DIRECTION ( 'NONE',  ( -0.9762722099447388446, -0.2165469281463391626, 0.000000000000000000 ) ) ;
#5577=CARTESIAN_POINT ( 'NONE',  ( -32.04500338604974985, 25.44370296803430520, -10.00000000000000000 ) ) ;
#5584=ORIENTED_EDGE ( 'NONE', *, *, #60442, .T. ) ;
#5585=VECTOR ( 'NONE', #94859, 1000.000000000000000 ) ;
#5590=VERTEX_POINT ( 'NONE', #27962 ) ;
#5597=CARTESIAN_POINT ( 'NONE',  ( -78.71521058394759507, 57.86724000996476747, 10.00000000000000000 ) ) ;
#5600=ORIENTED_EDGE ( 'NONE', *, *, #29657, .T. ) ;
#5604=LINE ( 'NONE', #53195, #83752 ) ;
#5606=CARTESIAN_POINT ( 'NONE',  ( -4.300976545156382613, 36.43331849613671380, 59.99999999999999289 ) ) ;
#5608=LINE ( 'NONE', #43603, #56674 ) ;
#5609=EDGE_LOOP ( 'NONE', ( #17454, #71606, #16795, #31414 ) ) ;
#5610=DIRECTION ( 'NONE',  ( 0.000000000000000000, -0.000000000000000000, -1.000000000000000000 ) ) ;
#5618=DIRECTION ( 'NONE',  ( 1.000000000000000000, 0.000000000000000000, 0.000000000000000000 ) ) ;
#5620=LINE ( 'NONE', #14717, #59644 ) ;
#5621=CARTESIAN_POINT ( 'NONE',  ( -19.65312891409030271, 93.06504152958497400, 10.00000000000000888 ) ) ;
#5637=FACE_OUTER_BOUND ( 'NONE', #49533, .T. ) ;
#5638=LINE ( 'NONE', #28952, #88035 ) ;
#5644=EDGE_CURVE ( 'NONE', #1734, #46146, #23341, .T. ) ;
#5647=DIRECTION ( 'NONE',  ( -0.000000000000000000, -0.000000000000000000, -1.000000000000000000 ) ) ;
#5659=PLANE ( 'NONE',  #13232 ) ;
#5664=FACE_OUTER_BOUND ( 'NONE', #8960, .T. ) ;
#5667=FACE_OUTER_BOUND ( 'NONE', #21316, .T. ) ;
#5672=DIRECTION ( 'NONE',  ( 1.000000000000000000, -9.773927698932179522E-14, 0.000000000000000000 ) ) ;
#5676=ORIENTED_EDGE ( 'NONE', *, *, #71364, .F. ) ;
#5678=CARTESIAN_POINT ( 'NONE',  ( 44.10470679282203577, 121.9603419428074460, 177.5919119679930134 ) ) ;
#5681=ORIENTED_EDGE ( 'NONE', *, *, #55658, .F. ) ;
#5685=DIRECTION ( 'NONE',  ( -0.8614378286617615510, 0.5078630399532038098, 0.000000000000000000 ) ) ;
#5687=AXIS2_PLACEMENT_3D ( 'NONE', #53264, #85208, #91307 ) ;
#5688=ORIENTED_EDGE ( 'NONE', *, *, #59691, .T. ) ;
#5691=ORIENTED_EDGE ( 'NONE', *, *, #71320, .F. ) ;
#5695=VERTEX_POINT ( 'NONE', #11181 ) ;
#5697=LINE ( 'NONE', #4723, #48288 ) ;
#5728=CYLINDRICAL_SURFACE ( 'NONE', #17698, 49.99999999999999289 ) ;
#5734=CARTESIAN_POINT ( 'NONE',  ( -19.65312891409030271, 93.06504152958497400, -10.00000000000000888 ) ) ;
#5740=ORIENTED_EDGE ( 'NONE', *, *, #17098, .T. ) ;
#5742=CARTESIAN_POINT ( 'NONE',  ( 37.30626620713776731, 103.7037781670604204, 59.99999999999999289 ) ) ;
#5755=EDGE_CURVE ( 'NONE', #30892, #35128, #35448, .T. ) ;
#5765=DIRECTION ( 'NONE',  ( -1.000000000000000000, 0.000000000000000000, 0.000000000000000000 ) ) ;
#5768=VECTOR ( 'NONE', #99056, 1000.000000000000000 ) ;
#5776=LINE ( 'NONE', #67572, #51309 ) ;
#5786=ORIENTED_EDGE ( 'NONE', *, *, #15936, .T. ) ;
#5790=ADVANCED_FACE ( 'NONE', ( #58728 ), #88216, .F. ) ;
#5805=CARTESIAN_POINT ( 'NONE',  ( 50.23025173566475132, 97.10399052176643409, -10.00000000000000000 ) ) ;
#5807=EDGE_LOOP ( 'NONE', ( #34590, #16460, #13308, #46550 ) ) ;
#5812=VERTEX_POINT ( 'NONE', #7038 ) ;
#5819=ORIENTED_EDGE ( 'NONE', *, *, #61708, .T. ) ;
#5825=ORIENTED_EDGE ( 'NONE', *, *, #66008, .T. ) ;
#5826=ADVANCED_FACE ( 'NONE', ( #69339 ), #75978, .T. ) ;
#5832=EDGE_CURVE ( 'NONE', #82529, #85923, #53139, .T. ) ;
#5838=VECTOR ( 'NONE', #91720, 1000.000000000000114 ) ;
#5839=EDGE_CURVE ( 'NONE', #83863, #59100, #84583, .T. ) ;
#5840=CARTESIAN_POINT ( 'NONE',  ( -29.41917662106829212, 23.74964416229699893, 177.5919119679930134 ) ) ;
#5842=ORIENTED_EDGE ( 'NONE', *, *, #4555, .T. ) ;
#5857=ORIENTED_EDGE ( 'NONE', *, *, #89622, .F. ) ;
#5861=CARTESIAN_POINT ( 'NONE',  ( 47.39496755818312579, 108.2889530649357681, -10.00000000000000000 ) ) ;
#5869=VECTOR ( 'NONE', #31768, 1000.000000000000000 ) ;
#5870=ORIENTED_EDGE ( 'NONE', *, *, #20040, .T. ) ;
#5875=CARTESIAN_POINT ( 'NONE',  ( -19.64547786486492598, 92.92342514603942050, 59.99999999999999289 ) ) ;
#5888=DIRECTION ( 'NONE',  ( 0.8435938723211464652, 0.5369817302126890235, 0.000000000000000000 ) ) ;
#5893=CARTESIAN_POINT ( 'NONE',  ( -49.85285084787511067, 106.9394001011715574, -10.00000000000000000 ) ) ;
#5897=CARTESIAN_POINT ( 'NONE',  ( -19.65312891409030271, 93.06504152958497400, -10.00000000000000888 ) ) ;
#5905=DIRECTION ( 'NONE',  ( 0.2126238682951520631, -0.9771341211068242938, 0.000000000000000000 ) ) ;
#5907=ORIENTED_EDGE ( 'NONE', *, *, #47331, .T. ) ;
#5909=DIRECTION ( 'NONE',  ( 0.001368469433193631119, -0.9999990636452669168, 0.000000000000000000 ) ) ;
#5913=EDGE_CURVE ( 'NONE', #82593, #22789, #38424, .T. ) ;
#5915=EDGE_CURVE ( 'NONE', #74024, #95321, #27211, .T. ) ;
#5919=CARTESIAN_POINT ( 'NONE',  ( -51.02451589650411989, 104.0357803128446506, -10.00000000000000000 ) ) ;
#5925=CYLINDRICAL_SURFACE ( 'NONE', #87042, 70.00000000000002842 ) ;
#5926=VERTEX_POINT ( 'NONE', #28854 ) ;
#5928=ORIENTED_EDGE ( 'NONE', *, *, #80627, .T. ) ;
#5933=LINE ( 'NONE', #43922, #98454 ) ;
#5934=VECTOR ( 'NONE', #44733, 1000.000000000000114 ) ;
#5939=FACE_OUTER_BOUND ( 'NONE', #87722, .T. ) ;
#5941=VECTOR ( 'NONE', #2668, 1000.000000000000000 ) ;
#5949=LINE ( 'NONE', #337, #2035 ) ;
#5962=ORIENTED_EDGE ( 'NONE', *, *, #1186, .F. ) ;
#5972=ORIENTED_EDGE ( 'NONE', *, *, #42937, .F. ) ;
#5977=CARTESIAN_POINT ( 'NONE',  ( 30.34687108590969373, 93.06504152958497400, 20.00000000000000355 ) ) ;
#5978=DIRECTION ( 'NONE',  ( -0.6835488936653838499, -0.7299047266382302501, 0.000000000000000000 ) ) ;
#5980=VERTEX_POINT ( 'NONE', #94678 ) ;
#5981=AXIS2_PLACEMENT_3D ( 'NONE', #51156, #82120, #50173 ) ;
#5987=CARTESIAN_POINT ( 'NONE',  ( 26.69679556076013327, 57.08553156527587902, 59.99999999999999289 ) ) ;
#5988=ADVANCED_FACE ( 'NONE', ( #946 ), #24246, .F. ) ;
#5996=DIRECTION ( 'NONE',  ( -0.000000000000000000, 0.000000000000000000, -1.000000000000000000 ) ) ;
#5997=EDGE_CURVE ( 'NONE', #11925, #26012, #56122, .T. ) ;
#6000=CARTESIAN_POINT ( 'NONE',  ( 45.86253193465722688, 68.41350641406140198, 177.5919119679930134 ) ) ;
#6005=LINE ( 'NONE', #28297, #67671 ) ;
#6006=CARTESIAN_POINT ( 'NONE',  ( 46.60452734134890562, 70.48356709729735314, 10.00000000000000000 ) ) ;
#6010=DIRECTION ( 'NONE',  ( -1.000000000000000000, 0.000000000000000000, 0.000000000000000000 ) ) ;
#6011=ADVANCED_FACE ( 'NONE', ( #16141 ), #77956, .F. ) ;
#6031=ORIENTED_EDGE ( 'NONE', *, *, #32862, .F. ) ;
#6033=ORIENTED_EDGE ( 'NONE', *, *, #82743, .T. ) ;
#6043=CIRCLE ( 'NONE', #38353, 0.1418229129681557177 ) ;
#6044=CARTESIAN_POINT ( 'NONE',  ( 12.00096474099108512, 32.03863464977598596, -10.00000000000000000 ) ) ;
#6050=FACE_OUTER_BOUND ( 'NONE', #46410, .T. ) ;
#6051=VERTEX_POINT ( 'NONE', #31336 ) ;
#6052=CARTESIAN_POINT ( 'NONE',  ( 48.38981961164311940, 109.5014996615669105, -10.00000000000000000 ) ) ;
#6053=DIRECTION ( 'NONE',  ( -0.9055221650797523614, -0.4242989612870595728, 0.000000000000000000 ) ) ;
#6055=EDGE_LOOP ( 'NONE', ( #61402, #24511, #21152, #90923 ) ) ;
#6056=VECTOR ( 'NONE', #74434, 1000.000000000000114 ) ;
#6067=ORIENTED_EDGE ( 'NONE', *, *, #24192, .F. ) ;
#6071=ORIENTED_EDGE ( 'NONE', *, *, #85123, .T. ) ;
#6075=ORIENTED_EDGE ( 'NONE', *, *, #73317, .T. ) ;
#6090=LINE ( 'NONE', #96843, #6545 ) ;
#6103=CARTESIAN_POINT ( 'NONE',  ( 28.75210520338636044, 111.3165232727998415, 59.99999999999999289 ) ) ;
#6115=VECTOR ( 'NONE', #20375, 1000.000000000000114 ) ;
#6119=CARTESIAN_POINT ( 'NONE',  ( 47.84007798744509898, 106.1754093786579318, -10.00000000000000000 ) ) ;
#6135=LINE ( 'NONE', #36528, #20600 ) ;
#6145=LINE ( 'NONE', #76076, #40922 ) ;
#6148=EDGE_CURVE ( 'NONE', #36369, #79500, #25619, .T. ) ;
#6151=EDGE_CURVE ( 'NONE', #96434, #77358, #82289, .T. ) ;
#6154=CARTESIAN_POINT ( 'NONE',  ( 50.15574305400770072, 101.0118721476823964, -10.00000000000000000 ) ) ;
#6157=DIRECTION ( 'NONE',  ( 0.5607300124661794838, -0.8279987035736700030, 0.000000000000000000 ) ) ;
#6169=DIRECTION ( 'NONE',  ( 0.9628097264997651505, -0.2701803667135113662, 0.000000000000000000 ) ) ;
#6179=AXIS2_PLACEMENT_3D ( 'NONE', #59047, #88050, #34284 ) ;
#6182=DIRECTION ( 'NONE',  ( -0.7909930170786233505, 0.6118251767726273771, 0.000000000000000000 ) ) ;
#6194=VERTEX_POINT ( 'NONE', #19665 ) ;
#6200=ORIENTED_EDGE ( 'NONE', *, *, #85678, .F. ) ;
#6201=AXIS2_PLACEMENT_3D ( 'NONE', #52779, #22394, #15272 ) ;
#6219=CARTESIAN_POINT ( 'NONE',  ( 36.38358746446922254, 51.11404133282110962, 177.5919119679930134 ) ) ;
#6225=VECTOR ( 'NONE', #82490, 1000.000000000000000 ) ;
#6236=VECTOR ( 'NONE', #49109, 1000.000000000000114 ) ;
#6238=ORIENTED_EDGE ( 'NONE', *, *, #100231, .F. ) ;
#6248=VECTOR ( 'NONE', #46702, 1000.000000000000000 ) ;
#6249=ORIENTED_EDGE ( 'NONE', *, *, #59634, .T. ) ;
#6251=VECTOR ( 'NONE', #40125, 1000.000000000000114 ) ;
#6253=CARTESIAN_POINT ( 'NONE',  ( -69.57603038520839789, 62.23413909710347980, 59.99999999999999289 ) ) ;
#6256=VECTOR ( 'NONE', #22984, 1000.000000000000227 ) ;
#6264=CARTESIAN_POINT ( 'NONE',  ( -23.73952538801239598, 24.43184193311134678, -10.00000000000000000 ) ) ;
#6268=ORIENTED_EDGE ( 'NONE', *, *, #92878, .T. ) ;
#6275=CARTESIAN_POINT ( 'NONE',  ( -9.517469918280088592, 23.54023200771947799, -10.00000000000000000 ) ) ;
#6276=EDGE_CURVE ( 'NONE', #63506, #91070, #5933, .T. ) ;
#6289=AXIS2_PLACEMENT_3D ( 'NONE', #43508, #51103, #19741 ) ;
#6297=CARTESIAN_POINT ( 'NONE',  ( 9.837252142675987798, 71.98620320469845524, 1.836970198720989751E-15 ) ) ;
#6302=FACE_OUTER_BOUND ( 'NONE', #74654, .T. ) ;
#6303=VERTEX_POINT ( 'NONE', #30731 ) ;
#6305=PLANE ( 'NONE',  #27315 ) ;
#6309=DIRECTION ( 'NONE',  ( -0.5634352399127593447, -0.8261602328994366307, 0.000000000000000000 ) ) ;
#6310=DIRECTION ( 'NONE',  ( -0.000000000000000000, -0.000000000000000000, -1.000000000000000000 ) ) ;
#6314=ORIENTED_EDGE ( 'NONE', *, *, #48937, .F. ) ;
#6320=ORIENTED_EDGE ( 'NONE', *, *, #29714, .T. ) ;
#6321=ORIENTED_EDGE ( 'NONE', *, *, #17732, .T. ) ;
#6322=ORIENTED_EDGE ( 'NONE', *, *, #78793, .T. ) ;
#6326=DIRECTION ( 'NONE',  ( -1.000000000000000000, 0.000000000000000000, 0.000000000000000000 ) ) ;
#6327=ORIENTED_EDGE ( 'NONE', *, *, #85853, .F. ) ;
#6332=AXIS2_PLACEMENT_3D ( 'NONE', #71612, #71109, #24980 ) ;
#6334=LINE ( 'NONE', #29633, #12246 ) ;
#6339=ORIENTED_EDGE ( 'NONE', *, *, #94964, .F. ) ;
#6340=ADVANCED_FACE ( 'NONE', ( #5443 ), #98155, .F. ) ;
#6342=DIRECTION ( 'NONE',  ( -0.9874733399847794857, -0.1577859398657057433, 0.000000000000000000 ) ) ;
#6343=CIRCLE ( 'NONE', #51604, 70.00000000000001421 ) ;
#6350=DIRECTION ( 'NONE',  ( -0.000000000000000000, 0.000000000000000000, -1.000000000000000000 ) ) ;
#6359=EDGE_CURVE ( 'NONE', #50322, #83565, #57934, .T. ) ;
#6361=CARTESIAN_POINT ( 'NONE',  ( -52.57320609282758994, 32.70376883311633520, -10.00000000000000000 ) ) ;
#6363=LINE ( 'NONE', #5861, #79431 ) ;
#6366=PLANE ( 'NONE',  #61347 ) ;
#6369=AXIS2_PLACEMENT_3D ( 'NONE', #31175, #15470, #94030 ) ;
#6372=VERTEX_POINT ( 'NONE', #1333 ) ;
#6373=FACE_OUTER_BOUND ( 'NONE', #33608, .T. ) ;
#6374=FACE_OUTER_BOUND ( 'NONE', #43332, .T. ) ;
#6391=EDGE_CURVE ( 'NONE', #63506, #35869, #40800, .T. ) ;
#6392=EDGE_CURVE ( 'NONE', #31723, #71916, #63120, .T. ) ;
#6397=EDGE_CURVE ( 'NONE', #39676, #31611, #24010, .T. ) ;
#6404=VECTOR ( 'NONE', #98362, 1000.000000000000000 ) ;
#6411=DIRECTION ( 'NONE',  ( -0.9820299053580098247, -0.1887253692075822886, 0.000000000000000000 ) ) ;
#6432=ORIENTED_EDGE ( 'NONE', *, *, #57621, .F. ) ;
#6435=ORIENTED_EDGE ( 'NONE', *, *, #88569, .F. ) ;
#6442=LINE ( 'NONE', #69719, #28418 ) ;
#6449=DIRECTION ( 'NONE',  ( 1.000000000000000000, 0.000000000000000000, 0.000000000000000000 ) ) ;
#6453=LINE ( 'NONE', #91572, #48156 ) ;
#6461=ORIENTED_EDGE ( 'NONE', *, *, #14894, .T. ) ;
#6469=DIRECTION ( 'NONE',  ( 0.5011331959107268030, 0.8653701635463872943, 0.000000000000000000 ) ) ;
#6476=LINE ( 'NONE', #84018, #31696 ) ;
#6477=VERTEX_POINT ( 'NONE', #11198 ) ;
#6479=EDGE_CURVE ( 'NONE', #75209, #26122, #47658, .T. ) ;
#6480=AXIS2_PLACEMENT_3D ( 'NONE', #55516, #94577, #16040 ) ;
#6482=FACE_OUTER_BOUND ( 'NONE', #37960, .T. ) ;
#6484=LINE ( 'NONE', #99190, #32228 ) ;
#6487=ORIENTED_EDGE ( 'NONE', *, *, #37774, .F. ) ;
#6498=AXIS2_PLACEMENT_3D ( 'NONE', #73295, #80430, #11003 ) ;
#6513=CARTESIAN_POINT ( 'NONE',  ( -19.65312891409030271, 93.06504152958497400, -10.00000000000000888 ) ) ;
#6516=ADVANCED_FACE ( 'NONE', ( #3591 ), #59235, .T. ) ;
#6536=LINE ( 'NONE', #51121, #16956 ) ;
#6540=ORIENTED_EDGE ( 'NONE', *, *, #15936, .F. ) ;
#6545=VECTOR ( 'NONE', #4599, 1000.000000000000000 ) ;
#6548=DIRECTION ( 'NONE',  ( 1.000000000000000000, 1.855658484016332714E-13, 0.000000000000000000 ) ) ;
#6552=CARTESIAN_POINT ( 'NONE',  ( -3.376183997657045133, 64.08949848310733444, -10.00000000000000000 ) ) ;
#6558=DIRECTION ( 'NONE',  ( 0.4270171210482451851, -0.9042435392811322137, 0.000000000000000000 ) ) ;
#6560=CARTESIAN_POINT ( 'NONE',  ( 47.05668214639808156, 76.45164061169337799, 10.00000000000000000 ) ) ;
#6562=ORIENTED_EDGE ( 'NONE', *, *, #77355, .F. ) ;
#6563=VECTOR ( 'NONE', #69889, 1000.000000000000114 ) ;
#6567=DIRECTION ( 'NONE',  ( -1.000000000000000000, 0.000000000000000000, 0.000000000000000000 ) ) ;
#6570=DIRECTION ( 'NONE',  ( -0.6857383512133925496, -0.7278481391575704063, 0.000000000000000000 ) ) ;
#6573=EDGE_CURVE ( 'NONE', #73457, #24730, #91065, .T. ) ;
#6578=ORIENTED_EDGE ( 'NONE', *, *, #73874, .T. ) ;
#6581=CARTESIAN_POINT ( 'NONE',  ( -6.542761065016642341, 25.57183462804972507, -10.00000000000000000 ) ) ;
#6582=VERTEX_POINT ( 'NONE', #14024 ) ;
#6585=ORIENTED_EDGE ( 'NONE', *, *, #1126, .T. ) ;
#6586=DIRECTION ( 'NONE',  ( -1.000000000000000000, 0.000000000000000000, 0.000000000000000000 ) ) ;
#6598=EDGE_CURVE ( 'NONE', #66853, #49704, #40122, .T. ) ;
#6602=DIRECTION ( 'NONE',  ( -0.7510153523339188064, 0.6602847420308604054, 0.000000000000000000 ) ) ;
#6606=DIRECTION ( 'NONE',  ( 0.5866775868892262213, 0.8098206029991052990, 0.000000000000000000 ) ) ;
#6628=DIRECTION ( 'NONE',  ( 0.9995565931350004485, 0.02977611660964677581, 0.000000000000000000 ) ) ;
#6633=CARTESIAN_POINT ( 'NONE',  ( 36.81131572470497559, 77.10862815663108449, 59.99999999999999289 ) ) ;
#6634=EDGE_CURVE ( 'NONE', #37194, #94538, #27738, .T. ) ;
#6636=LINE ( 'NONE', #525, #80880 ) ;
#6647=DIRECTION ( 'NONE',  ( -0.7492053821869066876, -0.6623377501714446947, 0.000000000000000000 ) ) ;
#6648=DIRECTION ( 'NONE',  ( -0.8917477921037005872, -0.4525327339300165286, 0.000000000000000000 ) ) ;
#6649=EDGE_CURVE ( 'NONE', #53961, #70584, #21148, .T. ) ;
#6653=CARTESIAN_POINT ( 'NONE',  ( 37.35766167792363746, 103.4248275259887748, 59.99999999999999289 ) ) ;
#6656=LINE ( 'NONE', #68932, #81233 ) ;
#6668=ORIENTED_EDGE ( 'NONE', *, *, #37258, .F. ) ;
#6675=DIRECTION ( 'NONE',  ( 0.000000000000000000, 0.000000000000000000, 1.000000000000000000 ) ) ;
#6681=CYLINDRICAL_SURFACE ( 'NONE', #76667, 70.00000000000002842 ) ;
#6688=VERTEX_POINT ( 'NONE', #2792 ) ;
#6690=EDGE_LOOP ( 'NONE', ( #89887, #38743, #67976, #1636 ) ) ;
#6693=VERTEX_POINT ( 'NONE', #26071 ) ;
#6697=CARTESIAN_POINT ( 'NONE',  ( -16.74804229723488191, 74.64713832601701426, 13.42402697601097117 ) ) ;
#6700=CARTESIAN_POINT ( 'NONE',  ( -19.72006729068866804, 93.19007349502240345, 59.99999999999999289 ) ) ;
#6703=AXIS2_PLACEMENT_3D ( 'NONE', #84323, #45273, #77174 ) ;
#6716=CARTESIAN_POINT ( 'NONE',  ( 45.88188149789386472, 72.29567966924399514, -10.00000000000000000 ) ) ;
#6727=ADVANCED_FACE ( 'NONE', ( #49362 ), #72694, .F. ) ;
#6734=DIRECTION ( 'NONE',  ( -0.9689225787001356505, 0.2473641778533817170, 0.000000000000000000 ) ) ;
#6748=LINE ( 'NONE', #38113, #80524 ) ;
#6751=DIRECTION ( 'NONE',  ( -0.000000000000000000, 0.000000000000000000, -1.000000000000000000 ) ) ;
#6761=CARTESIAN_POINT ( 'NONE',  ( -2.073866539663252073, 26.60322154129611505, -10.00000000000000000 ) ) ;
#6769=ORIENTED_EDGE ( 'NONE', *, *, #34632, .F. ) ;
#6770=AXIS2_PLACEMENT_3D ( 'NONE', #94788, #87233, #39523 ) ;
#6779=CARTESIAN_POINT ( 'NONE',  ( -17.26243516413818924, 24.35187462261283997, -10.00000000000000000 ) ) ;
#6783=EDGE_CURVE ( 'NONE', #22179, #73260, #9411, .T. ) ;
#6787=ORIENTED_EDGE ( 'NONE', *, *, #11107, .T. ) ;
#6789=CARTESIAN_POINT ( 'NONE',  ( -78.94662368502558536, 55.85910816071121587, -10.00000000000000000 ) ) ;
#6793=CARTESIAN_POINT ( 'NONE',  ( -38.61298035630893111, 26.97617139035147460, 10.00000000000000000 ) ) ;
#6796=VERTEX_POINT ( 'NONE', #58443 ) ;
#6799=CARTESIAN_POINT ( 'NONE',  ( -19.65312891409030271, 93.06504152958497400, 177.5919119679930134 ) ) ;
#6800=ORIENTED_EDGE ( 'NONE', *, *, #72412, .F. ) ;
#6801=CARTESIAN_POINT ( 'NONE',  ( -69.85371643402891095, 44.28081239092799848, 10.00000000000000000 ) ) ;
#6804=VERTEX_POINT ( 'NONE', #49856 ) ;
#6817=ORIENTED_EDGE ( 'NONE', *, *, #8245, .T. ) ;
#6821=EDGE_LOOP ( 'NONE', ( #4200, #1217, #85881, #89360 ) ) ;
#6824=CYLINDRICAL_SURFACE ( 'NONE', #3251, 70.00000000000002842 ) ;
#6826=EDGE_LOOP ( 'NONE', ( #36094, #31480, #84349, #19910 ) ) ;
#6831=DIRECTION ( 'NONE',  ( 0.000000000000000000, 0.000000000000000000, 1.000000000000000000 ) ) ;
#6838=EDGE_CURVE ( 'NONE', #21034, #5053, #41243, .T. ) ;
#6843=DIRECTION ( 'NONE',  ( -0.1032265479692960342, 0.9946578707245736783, 0.000000000000000000 ) ) ;
#6854=VERTEX_POINT ( 'NONE', #50845 ) ;
#6855=ORIENTED_EDGE ( 'NONE', *, *, #45141, .F. ) ;
#6856=CARTESIAN_POINT ( 'NONE',  ( -30.95603806669010538, 23.98360954755322183, -10.00000000000000000 ) ) ;
#6857=CARTESIAN_POINT ( 'NONE',  ( -75.18208942163934694, 50.44421862632483311, -10.00000000000000000 ) ) ;
#6874=CARTESIAN_POINT ( 'NONE',  ( -19.65312891409030271, 93.06504152958497400, 177.5919119679930134 ) ) ;
#6875=VECTOR ( 'NONE', #30591, 1000.000000000000000 ) ;
#6882=LINE ( 'NONE', #83429, #44861 ) ;
#6917=ORIENTED_EDGE ( 'NONE', *, *, #45891, .T. ) ;
#6919=DIRECTION ( 'NONE',  ( -0.8951289669282589401, 0.4458072818673421422, 0.000000000000000000 ) ) ;
#6925=FACE_OUTER_BOUND ( 'NONE', #70462, .T. ) ;
#6934=DIRECTION ( 'NONE',  ( -0.6857383512134002101, -0.7278481391575631898, 0.000000000000000000 ) ) ;
#6935=DIRECTION ( 'NONE',  ( -0.9795703749556662343, 0.2011016670970565412, 0.000000000000000000 ) ) ;
#6944=LINE ( 'NONE', #61134, #41479 ) ;
#6947=ORIENTED_EDGE ( 'NONE', *, *, #75984, .T. ) ;
#6952=EDGE_CURVE ( 'NONE', #60043, #79260, #9243, .T. ) ;
#6953=CIRCLE ( 'NONE', #60370, 70.00000000000001421 ) ;
#6962=PLANE ( 'NONE',  #26949 ) ;
#6966=AXIS2_PLACEMENT_3D ( 'NONE', #61474, #53859, #96287 ) ;
#6967=EDGE_CURVE ( 'NONE', #56880, #78230, #38628, .T. ) ;
#6973=VERTEX_POINT ( 'NONE', #40118 ) ;
#6977=LINE ( 'NONE', #14086, #67802 ) ;
#6990=FACE_OUTER_BOUND ( 'NONE', #25679, .T. ) ;
#7007=EDGE_CURVE ( 'NONE', #31723, #20265, #46214, .T. ) ;
#7018=EDGE_CURVE ( 'NONE', #67254, #82333, #70027, .T. ) ;
#7031=ORIENTED_EDGE ( 'NONE', *, *, #14781, .T. ) ;
#7032=CIRCLE ( 'NONE', #50709, 70.00000000000001421 ) ;
#7033=DIRECTION ( 'NONE',  ( 1.000000000000000000, 0.000000000000000000, 0.000000000000000000 ) ) ;
#7038=CARTESIAN_POINT ( 'NONE',  ( -66.55019942848203129, 42.78701949053055387, -10.00000000000000000 ) ) ;
#7039=VERTEX_POINT ( 'NONE', #53817 ) ;
#7042=DIRECTION ( 'NONE',  ( -0.8770933717188629242, -0.4803199113995137437, 0.000000000000000000 ) ) ;
#7043=EDGE_CURVE ( 'NONE', #58283, #10175, #70532, .T. ) ;
#7048=ORIENTED_EDGE ( 'NONE', *, *, #19660, .T. ) ;
#7055=CARTESIAN_POINT ( 'NONE',  ( -19.65312891409030271, 93.06504152958497400, 10.00000000000000888 ) ) ;
#7063=ORIENTED_EDGE ( 'NONE', *, *, #11979, .F. ) ;
#7064=CARTESIAN_POINT ( 'NONE',  ( 32.30839531297598199, 123.0650415295850593, -60.00000000000000000 ) ) ;
#7065=ORIENTED_EDGE ( 'NONE', *, *, #85582, .F. ) ;
#7079=EDGE_CURVE ( 'NONE', #78204, #68063, #17852, .T. ) ;
#7080=ADVANCED_FACE ( 'NONE', ( #3651 ), #34531, .F. ) ;
#7082=VECTOR ( 'NONE', #55718, 999.9999999999998863 ) ;
#7083=EDGE_CURVE ( 'NONE', #67877, #76666, #72051, .T. ) ;
#7087=ORIENTED_EDGE ( 'NONE', *, *, #68019, .F. ) ;
#7090=DIRECTION ( 'NONE',  ( -1.000000000000000000, 0.000000000000000000, 0.000000000000000000 ) ) ;
#7091=EDGE_CURVE ( 'NONE', #18050, #24730, #4126, .T. ) ;
#7095=CIRCLE ( 'NONE', #2281, 0.1418229129684506207 ) ;
#7097=ORIENTED_EDGE ( 'NONE', *, *, #20698, .T. ) ;
#7099=CARTESIAN_POINT ( 'NONE',  ( -19.65312891409030271, 93.06504152958497400, -10.00000000000000888 ) ) ;
#7103=ORIENTED_EDGE ( 'NONE', *, *, #50199, .F. ) ;
#7107=DIRECTION ( 'NONE',  ( -0.7561390817803210762, 0.6544109481086124447, 0.000000000000000000 ) ) ;
#7111=LINE ( 'NONE', #76048, #82351 ) ;
#7116=PLANE ( 'NONE',  #24194 ) ;
#7117=EDGE_LOOP ( 'NONE', ( #367, #26154, #1745, #35741 ) ) ;
#7131=DIRECTION ( 'NONE',  ( 0.9981280818701453450, 0.06115825522547521653, 0.000000000000000000 ) ) ;
#7134=CARTESIAN_POINT ( 'NONE',  ( -14.83894680564148238, 24.48641780169620219, -10.00000000000000000 ) ) ;
#7137=CARTESIAN_POINT ( 'NONE',  ( 42.45923888023187232, 122.5484010731363043, 10.00000000000000000 ) ) ;
#7148=VERTEX_POINT ( 'NONE', #82180 ) ;
#7151=CARTESIAN_POINT ( 'NONE',  ( -19.10035114162887737, 41.33634930963552279, 59.99999999999999289 ) ) ;
#7153=EDGE_CURVE ( 'NONE', #30262, #70893, #60791, .T. ) ;
#7161=EDGE_LOOP ( 'NONE', ( #92672, #19343, #85360, #2232 ) ) ;
#7168=DIRECTION ( 'NONE',  ( 0.5544813661758196677, 0.8321961394790273747, 0.000000000000000000 ) ) ;
#7172=CIRCLE ( 'NONE', #39549, 0.1418229129684575596 ) ;
#7180=ORIENTED_EDGE ( 'NONE', *, *, #78042, .T. ) ;
#7181=DIRECTION ( 'NONE',  ( 0.000000000000000000, 0.000000000000000000, 1.000000000000000000 ) ) ;
#7196=EDGE_CURVE ( 'NONE', #66499, #6194, #58004, .T. ) ;
#7213=ORIENTED_EDGE ( 'NONE', *, *, #78877, .T. ) ;
#7222=DIRECTION ( 'NONE',  ( 0.000000000000000000, 0.000000000000000000, 1.000000000000000000 ) ) ;
#7226=EDGE_LOOP ( 'NONE', ( #49077, #100262, #35616, #57875 ) ) ;
#7231=CARTESIAN_POINT ( 'NONE',  ( 46.32860941106298469, 116.4404604047837779, 177.5919119679930134 ) ) ;
#7232=VECTOR ( 'NONE', #19733, 1000.000000000000227 ) ;
#7235=CARTESIAN_POINT ( 'NONE',  ( -25.86065208768103219, 41.70698537633906255, 59.99999999999999289 ) ) ;
#7254=ORIENTED_EDGE ( 'NONE', *, *, #54717, .T. ) ;
#7262=DIRECTION ( 'NONE',  ( 0.000000000000000000, 0.000000000000000000, 1.000000000000000000 ) ) ;
#7264=EDGE_CURVE ( 'NONE', #90523, #11943, #13724, .T. ) ;
#7268=ORIENTED_EDGE ( 'NONE', *, *, #85914, .F. ) ;
#7274=ORIENTED_EDGE ( 'NONE', *, *, #22277, .F. ) ;
#7276=VECTOR ( 'NONE', #26233, 1000.000000000000000 ) ;
#7287=CARTESIAN_POINT ( 'NONE',  ( -22.72465050930169994, 22.87247442008841958, 10.00000000000000000 ) ) ;
#7288=CARTESIAN_POINT ( 'NONE',  ( -71.61465314115659453, 63.06504152958490295, 10.00000000000000888 ) ) ;
#7289=ORIENTED_EDGE ( 'NONE', *, *, #84191, .F. ) ;
#7294=ORIENTED_EDGE ( 'NONE', *, *, #95774, .F. ) ;
#7295=DIRECTION ( 'NONE',  ( 1.000000000000000000, 0.000000000000000000, 0.000000000000000000 ) ) ;
#7308=ORIENTED_EDGE ( 'NONE', *, *, #68211, .T. ) ;
#7310=AXIS2_PLACEMENT_3D ( 'NONE', #27249, #66729, #28230 ) ;
#7311=VERTEX_POINT ( 'NONE', #14718 ) ;
#7319=CIRCLE ( 'NONE', #65608, 70.00000000000001421 ) ;
#7334=VERTEX_POINT ( 'NONE', #30 ) ;
#7336=CARTESIAN_POINT ( 'NONE',  ( -22.72465050930169994, 22.87247442008841958, -10.00000000000000000 ) ) ;
#7339=LINE ( 'NONE', #100068, #27621 ) ;
#7352=VECTOR ( 'NONE', #44199, 1000.000000000000000 ) ;
#7353=LINE ( 'NONE', #67669, #95506 ) ;
#7367=VECTOR ( 'NONE', #16895, 1000.000000000000114 ) ;
#7368=CARTESIAN_POINT ( 'NONE',  ( 15.82905546192370494, 46.33330469044422983, 59.99999999999999289 ) ) ;
#7373=DIRECTION ( 'NONE',  ( -0.5280678506503699854, -0.8492021815265776707, 0.000000000000000000 ) ) ;
#7376=CIRCLE ( 'NONE', #76942, 70.00000000000001421 ) ;
#7377=CARTESIAN_POINT ( 'NONE',  ( -67.91103796225580425, 44.10201266000169085, -10.00000000000000000 ) ) ;
#7383=DIRECTION ( 'NONE',  ( -0.5951734788405994570, 0.8035972437015812542, 0.000000000000000000 ) ) ;
#7389=LINE ( 'NONE', #24091, #67747 ) ;
#7396=ADVANCED_FACE ( 'NONE', ( #521 ), #31408, .T. ) ;
#7397=DIRECTION ( 'NONE',  ( -1.000000000000000000, 0.000000000000000000, 0.000000000000000000 ) ) ;
#7398=DIRECTION ( 'NONE',  ( -0.9762722099447388446, -0.2165469281463391626, 0.000000000000000000 ) ) ;
#7400=EDGE_CURVE ( 'NONE', #76991, #97421, #66683, .T. ) ;
#7405=ADVANCED_FACE ( 'NONE', ( #80562 ), #18227, .F. ) ;
#7407=VERTEX_POINT ( 'NONE', #94749 ) ;
#7418=VECTOR ( 'NONE', #20191, 1000.000000000000000 ) ;
#7424=CIRCLE ( 'NONE', #73826, 11.89249999999999652 ) ;
#7444=VERTEX_POINT ( 'NONE', #10123 ) ;
#7445=CYLINDRICAL_SURFACE ( 'NONE', #83823, 6.749999999999988454 ) ;
#7447=DIRECTION ( 'NONE',  ( -1.000000000000000000, 0.000000000000000000, 0.000000000000000000 ) ) ;
#7451=ORIENTED_EDGE ( 'NONE', *, *, #90040, .T. ) ;
#7452=AXIS2_PLACEMENT_3D ( 'NONE', #81552, #20225, #82062 ) ;
#7453=LINE ( 'NONE', #77367, #52834 ) ;
#7454=ORIENTED_EDGE ( 'NONE', *, *, #97583, .T. ) ;
#7457=EDGE_LOOP ( 'NONE', ( #68987, #39055, #19288, #64040 ) ) ;
#7466=EDGE_LOOP ( 'NONE', ( #16361, #29232, #8163, #52616 ) ) ;
#7480=ADVANCED_FACE ( 'NONE', ( #24809 ), #34414, .F. ) ;
#7483=VECTOR ( 'NONE', #19716, 1000.000000000000000 ) ;
#7485=CARTESIAN_POINT ( 'NONE',  ( -19.65312891409030271, 93.06504152958497400, -10.00000000000000888 ) ) ;
#7486=VECTOR ( 'NONE', #39821, 1000.000000000000000 ) ;
#7490=PLANE ( 'NONE',  #24890 ) ;
#7496=CARTESIAN_POINT ( 'NONE',  ( -19.65312891409030271, 93.06504152958497400, -59.99999999999999289 ) ) ;
#7502=VECTOR ( 'NONE', #62413, 1000.000000000000000 ) ;
#7510=DIRECTION ( 'NONE',  ( 0.9919084036772433111, -0.1269555777209603609, 0.000000000000000000 ) ) ;
#7514=AXIS2_PLACEMENT_3D ( 'NONE', #60263, #38468, #93213 ) ;
#7530=ORIENTED_EDGE ( 'NONE', *, *, #62985, .F. ) ;
#7534=CARTESIAN_POINT ( 'NONE',  ( 50.06890205215325551, 99.29708757740750968, 10.00000000000000000 ) ) ;
#7542=DIRECTION ( 'NONE',  ( 0.7071067811865474617, 0.000000000000000000, 0.7071067811865474617 ) ) ;
#7565=ORIENTED_EDGE ( 'NONE', *, *, #15260, .F. ) ;
#7577=ORIENTED_EDGE ( 'NONE', *, *, #94957, .T. ) ;
#7579=CARTESIAN_POINT ( 'NONE',  ( -0.2492734796364602656, 27.10516647459198225, 10.00000000000000000 ) ) ;
#7580=ORIENTED_EDGE ( 'NONE', *, *, #96113, .F. ) ;
#7585=AXIS2_PLACEMENT_3D ( 'NONE', #29665, #90525, #21096 ) ;
#7589=AXIS2_PLACEMENT_3D ( 'NONE', #91727, #61779, #45091 ) ;
#7614=DIRECTION ( 'NONE',  ( -0.000000000000000000, -0.000000000000000000, 1.000000000000000000 ) ) ;
#7619=CARTESIAN_POINT ( 'NONE',  ( 49.91331508509971826, 100.8438505198844553, 177.5919119679930134 ) ) ;
#7622=DIRECTION ( 'NONE',  ( -0.000000000000000000, 0.000000000000000000, -1.000000000000000000 ) ) ;
#7625=CARTESIAN_POINT ( 'NONE',  ( 49.93482446054089507, 85.48106202472366988, 10.00000000000000000 ) ) ;
#7631=CARTESIAN_POINT ( 'NONE',  ( 38.52196584993465223, 56.41980893122115504, 10.00000000000000000 ) ) ;
#7636=AXIS2_PLACEMENT_3D ( 'NONE', #53078, #60160, #74419 ) ;
#7642=CARTESIAN_POINT ( 'NONE',  ( -33.12036098009136964, 24.37273002035945169, -10.00000000000000000 ) ) ;
#7655=ORIENTED_EDGE ( 'NONE', *, *, #47099, .T. ) ;
#7656=AXIS2_PLACEMENT_3D ( 'NONE', #84596, #23243, #15639 ) ;
#7669=ORIENTED_EDGE ( 'NONE', *, *, #82733, .F. ) ;
#7671=VECTOR ( 'NONE', #25991, 1000.000000000000114 ) ;
#7676=CARTESIAN_POINT ( 'NONE',  ( -50.66096862766640641, 31.69950886434491721, -10.00000000000000000 ) ) ;
#7678=CARTESIAN_POINT ( 'NONE',  ( -63.08903959183645327, 39.77784189046417396, 10.00000000000000000 ) ) ;
#7679=ORIENTED_EDGE ( 'NONE', *, *, #1880, .F. ) ;
#7682=ORIENTED_EDGE ( 'NONE', *, *, #26998, .F. ) ;
#7685=ORIENTED_EDGE ( 'NONE', *, *, #55264, .F. ) ;
#7689=CARTESIAN_POINT ( 'NONE',  ( -6.294050206057209884, 74.34147604373191598, 14.84309344784631080 ) ) ;
#7692=CARTESIAN_POINT ( 'NONE',  ( -78.71521058394759507, 57.86724000996476747, 10.00000000000000000 ) ) ;
#7693=ORIENTED_EDGE ( 'NONE', *, *, #2779, .T. ) ;
#7709=VECTOR ( 'NONE', #2453, 999.9999999999998863 ) ;
#7717=CARTESIAN_POINT ( 'NONE',  ( 39.64431452495995245, 58.26521502737223557, 10.00000000000000000 ) ) ;
#7721=VECTOR ( 'NONE', #53627, 1000.000000000000000 ) ;
#7727=VECTOR ( 'NONE', #7542, 1000.000000000000114 ) ;
#7733=CIRCLE ( 'NONE', #69194, 0.1418229129680858847 ) ;
#7737=DIRECTION ( 'NONE',  ( 0.000000000000000000, 0.000000000000000000, 1.000000000000000000 ) ) ;
#7740=EDGE_CURVE ( 'NONE', #54118, #54173, #63842, .T. ) ;
#7742=CARTESIAN_POINT ( 'NONE',  ( -8.109353775345800486, 61.89996032967495410, -10.00000000000000000 ) ) ;
#7745=AXIS2_PLACEMENT_3D ( 'NONE', #65694, #18115, #81446 ) ;
#7747=LINE ( 'NONE', #46739, #6251 ) ;
#7755=DIRECTION ( 'NONE',  ( -0.9263643838751195458, -0.3766285016932073293, 0.000000000000000000 ) ) ;
#7775=EDGE_CURVE ( 'NONE', #3488, #53634, #84283, .T. ) ;
#7777=ORIENTED_EDGE ( 'NONE', *, *, #78793, .F. ) ;
#7779=AXIS2_PLACEMENT_3D ( 'NONE', #47223, #17846, #86290 ) ;
#7784=CARTESIAN_POINT ( 'NONE',  ( -33.79156961297667294, 36.11817918669349581, 59.99999999999999289 ) ) ;
#7785=CIRCLE ( 'NONE', #45009, 70.00000000000001421 ) ;
#7786=EDGE_CURVE ( 'NONE', #37787, #34490, #58232, .T. ) ;
#7791=DIRECTION ( 'NONE',  ( 0.09547062131715944311, -0.9954322480537364237, 0.000000000000000000 ) ) ;
#7793=LINE ( 'NONE', #60976, #87261 ) ;
#7795=VECTOR ( 'NONE', #68295, 1000.000000000000000 ) ;
#7803=VERTEX_POINT ( 'NONE', #72477 ) ;
#7817=EDGE_LOOP ( 'NONE', ( #1320, #44662, #61100, #72372 ) ) ;
#7824=AXIS2_PLACEMENT_3D ( 'NONE', #25236, #70847, #63242 ) ;
#7827=CARTESIAN_POINT ( 'NONE',  ( -19.57455831887243036, 93.18311100154903670, 59.99999999999999289 ) ) ;
#7828=EDGE_CURVE ( 'NONE', #72764, #95045, #35438, .T. ) ;
#7829=DIRECTION ( 'NONE',  ( 0.9942962326340548662, 0.1066536533351087890, 0.000000000000000000 ) ) ;
#7832=DIRECTION ( 'NONE',  ( -0.3105719460338542404, -0.9505498757754611283, 0.000000000000000000 ) ) ;
#7834=VECTOR ( 'NONE', #68400, 1000.000000000000000 ) ;
#7837=LINE ( 'NONE', #46304, #23424 ) ;
#7848=CIRCLE ( 'NONE', #79037, 70.00000000000001421 ) ;
#7855=FACE_OUTER_BOUND ( 'NONE', #51529, .T. ) ;
#7857=VECTOR ( 'NONE', #96091, 1000.000000000000000 ) ;
#7863=VERTEX_POINT ( 'NONE', #37911 ) ;
#7869=EDGE_CURVE ( 'NONE', #9430, #40063, #49690, .T. ) ;
#7871=AXIS2_PLACEMENT_3D ( 'NONE', #69574, #99002, #23460 ) ;
#7881=VECTOR ( 'NONE', #69671, 1000.000000000000000 ) ;
#7886=CARTESIAN_POINT ( 'NONE',  ( -40.67952639183666008, 27.60432558407080350, -10.00000000000000000 ) ) ;
#7895=CARTESIAN_POINT ( 'NONE',  ( 32.30839531297598910, 123.0650415295850593, 203.6502102582797420 ) ) ;
#7898=CARTESIAN_POINT ( 'NONE',  ( 30.62257814894733698, 105.2525989182601194, 59.99999999999999289 ) ) ;
#7903=DIRECTION ( 'NONE',  ( -0.3473448497826165382, 0.9377374661009827417, 0.000000000000000000 ) ) ;
#7917=EDGE_CURVE ( 'NONE', #98290, #59369, #13646, .T. ) ;
#7919=LINE ( 'NONE', #17379, #50220 ) ;
#7920=CARTESIAN_POINT ( 'NONE',  ( 49.63464994930628649, 103.0251469596019120, -10.00000000000000000 ) ) ;
#7922=CARTESIAN_POINT ( 'NONE',  ( 44.18536904650256503, 64.34838820550514527, -10.00000000000000000 ) ) ;
#7924=VERTEX_POINT ( 'NONE', #74470 ) ;
#7926=AXIS2_PLACEMENT_3D ( 'NONE', #70764, #70255, #16561 ) ;
#7936=DIRECTION ( 'NONE',  ( 1.000000000000000000, 0.000000000000000000, 0.000000000000000000 ) ) ;
#7939=CARTESIAN_POINT ( 'NONE',  ( 23.64814127513158937, 118.0650415295850451, -24.99999999999999289 ) ) ;
#7944=ORIENTED_EDGE ( 'NONE', *, *, #12713, .T. ) ;
#7945=ORIENTED_EDGE ( 'NONE', *, *, #10017, .T. ) ;
#7947=AXIS2_PLACEMENT_3D ( 'NONE', #41847, #72795, #81398 ) ;
#7948=EDGE_LOOP ( 'NONE', ( #22873, #24495, #78486, #63746 ) ) ;
#7953=CARTESIAN_POINT ( 'NONE',  ( 30.34687108590969373, 93.06504152958497400, -45.00000000000001421 ) ) ;
#7955=CARTESIAN_POINT ( 'NONE',  ( 32.24342178309110096, 47.97677246190463052, -10.00000000000000000 ) ) ;
#7962=AXIS2_PLACEMENT_3D ( 'NONE', #63084, #40268, #15987 ) ;
#7964=FACE_OUTER_BOUND ( 'NONE', #38206, .T. ) ;
#7972=DIRECTION ( 'NONE',  ( -0.000000000000000000, 0.000000000000000000, 1.000000000000000000 ) ) ;
#7986=EDGE_LOOP ( 'NONE', ( #83273, #55679, #63909, #41721 ) ) ;
#8000=EDGE_CURVE ( 'NONE', #88645, #88734, #60942, .T. ) ;
#8020=VECTOR ( 'NONE', #97593, 999.9999999999998863 ) ;
#8028=CIRCLE ( 'NONE', #95445, 70.00000000000001421 ) ;
#8033=DIRECTION ( 'NONE',  ( 0.000000000000000000, -0.000000000000000000, 1.000000000000000000 ) ) ;
#8050=VERTEX_POINT ( 'NONE', #93391 ) ;
#8051=CARTESIAN_POINT ( 'NONE',  ( -19.65312891409030271, 93.06504152958497400, 177.5919119679930134 ) ) ;
#8058=LINE ( 'NONE', #53631, #53268 ) ;
#8060=ORIENTED_EDGE ( 'NONE', *, *, #52765, .T. ) ;
#8064=CARTESIAN_POINT ( 'NONE',  ( -19.78401074640790469, 93.01041841532075694, 59.99999999999999289 ) ) ;
#8072=ADVANCED_FACE ( 'NONE', ( #31540 ), #70040, .T. ) ;
#8078=VERTEX_POINT ( 'NONE', #1162 ) ;
#8082=DIRECTION ( 'NONE',  ( -0.9054088711727241723, 0.4245406647209821194, 0.000000000000000000 ) ) ;
#8087=DIRECTION ( 'NONE',  ( 0.6835488936653759673, 0.7299047266382376886, 0.000000000000000000 ) ) ;
#8091=AXIS2_PLACEMENT_3D ( 'NONE', #68663, #36276, #99586 ) ;
#8092=VERTEX_POINT ( 'NONE', #85823 ) ;
#8099=CIRCLE ( 'NONE', #90656, 0.1418229129681557177 ) ;
#8101=DIRECTION ( 'NONE',  ( -0.000000000000000000, -0.000000000000000000, -1.000000000000000000 ) ) ;
#8102=FACE_OUTER_BOUND ( 'NONE', #11429, .T. ) ;
#8117=DIRECTION ( 'NONE',  ( -0.000000000000000000, 0.000000000000000000, -1.000000000000000000 ) ) ;
#8118=ADVANCED_FACE ( 'NONE', ( #15842 ), #22943, .F. ) ;
#8123=FACE_OUTER_BOUND ( 'NONE', #33475, .T. ) ;
#8133=AXIS2_PLACEMENT_3D ( 'NONE', #89744, #20308, #27893 ) ;
#8153=DIRECTION ( 'NONE',  ( -0.000000000000000000, 0.000000000000000000, 1.000000000000000000 ) ) ;
#8154=CARTESIAN_POINT ( 'NONE',  ( 48.29091023345864642, 82.53782597618220507, -10.00000000000000000 ) ) ;
#8163=ORIENTED_EDGE ( 'NONE', *, *, #98832, .F. ) ;
#8170=LINE ( 'NONE', #55732, #8553 ) ;
#8174=EDGE_CURVE ( 'NONE', #80145, #57629, #84792, .T. ) ;
#8179=ORIENTED_EDGE ( 'NONE', *, *, #1363, .F. ) ;
#8184=EDGE_CURVE ( 'NONE', #57534, #13459, #9261, .T. ) ;
#8190=EDGE_LOOP ( 'NONE', ( #11816, #3710, #17508, #3501 ) ) ;
#8200=VERTEX_POINT ( 'NONE', #46751 ) ;
#8201=LINE ( 'NONE', #92340, #96599 ) ;
#8208=LINE ( 'NONE', #16300, #93651 ) ;
#8219=EDGE_CURVE ( 'NONE', #43051, #45411, #54327, .T. ) ;
#8222=DIRECTION ( 'NONE',  ( 0.000000000000000000, 0.000000000000000000, 1.000000000000000000 ) ) ;
#8227=ORIENTED_EDGE ( 'NONE', *, *, #41239, .F. ) ;
#8232=ADVANCED_FACE ( 'NONE', ( #65944 ), #96897, .T. ) ;
#8235=ADVANCED_FACE ( 'NONE', ( #89313 ), #76069, .T. ) ;
#8241=VERTEX_POINT ( 'NONE', #74831 ) ;
#8245=EDGE_CURVE ( 'NONE', #68766, #73260, #52003, .T. ) ;
#8254=ORIENTED_EDGE ( 'NONE', *, *, #65508, .T. ) ;
#8270=ORIENTED_EDGE ( 'NONE', *, *, #32550, .F. ) ;
#8295=AXIS2_PLACEMENT_3D ( 'NONE', #55879, #71634, #90347 ) ;
#8298=EDGE_LOOP ( 'NONE', ( #27743, #92476, #47293, #4169 ) ) ;
#8299=DIRECTION ( 'NONE',  ( -0.7059494278973847958, 0.7082622432767082810, 0.000000000000000000 ) ) ;
#8300=DIRECTION ( 'NONE',  ( -1.000000000000000000, 0.000000000000000000, 0.000000000000000000 ) ) ;
#8306=CARTESIAN_POINT ( 'NONE',  ( -19.65312891409030271, 93.06504152958497400, -10.00000000000000888 ) ) ;
#8310=VERTEX_POINT ( 'NONE', #53484 ) ;
#8313=DIRECTION ( 'NONE',  ( -0.7033187449715098127, 0.7108746323872447981, 0.000000000000000000 ) ) ;
#8314=ORIENTED_EDGE ( 'NONE', *, *, #65131, .T. ) ;
#8320=ORIENTED_EDGE ( 'NONE', *, *, #59425, .T. ) ;
#8334=VERTEX_POINT ( 'NONE', #85962 ) ;
#8341=CARTESIAN_POINT ( 'NONE',  ( -33.75225536883275623, 24.49963747467413100, 177.5919119679930134 ) ) ;
#8347=DIRECTION ( 'NONE',  ( 0.2776767122488391082, 0.9606745773021556634, 0.000000000000000000 ) ) ;
#8357=EDGE_CURVE ( 'NONE', #75006, #66118, #88458, .T. ) ;
#8360=EDGE_CURVE ( 'NONE', #92132, #85089, #97511, .T. ) ;
#8366=CIRCLE ( 'NONE', #6770, 0.1418229129681557177 ) ;
#8373=EDGE_LOOP ( 'NONE', ( #82400, #81364, #79540, #5600 ) ) ;
#8380=CARTESIAN_POINT ( 'NONE',  ( 43.33680334696484948, 124.1889737374328462, 10.00000000000000000 ) ) ;
#8383=LINE ( 'NONE', #37766, #48222 ) ;
#8387=CARTESIAN_POINT ( 'NONE',  ( -19.65312891409030271, 93.06504152958497400, 45.00000000000000711 ) ) ;
#8398=DIRECTION ( 'NONE',  ( -0.6855440362341557181, 0.7280311630581363103, 0.000000000000000000 ) ) ;
#8402=VERTEX_POINT ( 'NONE', #42765 ) ;
#8406=ORIENTED_EDGE ( 'NONE', *, *, #55999, .T. ) ;
#8410=DIRECTION ( 'NONE',  ( 0.000000000000000000, 0.000000000000000000, 1.000000000000000000 ) ) ;
#8412=ORIENTED_EDGE ( 'NONE', *, *, #41376, .F. ) ;
#8415=VERTEX_POINT ( 'NONE', #96041 ) ;
#8419=ORIENTED_EDGE ( 'NONE', *, *, #82703, .T. ) ;
#8431=ORIENTED_EDGE ( 'NONE', *, *, #21816, .T. ) ;
#8434=ORIENTED_EDGE ( 'NONE', *, *, #80875, .F. ) ;
#8436=VERTEX_POINT ( 'NONE', #30075 ) ;
#8438=PLANE ( 'NONE',  #42869 ) ;
#8439=ORIENTED_EDGE ( 'NONE', *, *, #36258, .F. ) ;
#8443=LINE ( 'NONE', #25130, #17252 ) ;
#8446=DIRECTION ( 'NONE',  ( -0.000000000000000000, -0.000000000000000000, -1.000000000000000000 ) ) ;
#8460=DIRECTION ( 'NONE',  ( -0.9054088711727241723, 0.4245406647209821194, 0.000000000000000000 ) ) ;
#8461=CARTESIAN_POINT ( 'NONE',  ( 45.11483101423404918, 69.99284853207299761, -10.00000000000000000 ) ) ;
#8463=VERTEX_POINT ( 'NONE', #82832 ) ;
#8465=ADVANCED_FACE ( 'NONE', ( #13401 ), #60962, .F. ) ;
#8469=EDGE_CURVE ( 'NONE', #22887, #63648, #2191, .T. ) ;
#8473=FACE_OUTER_BOUND ( 'NONE', #44070, .T. ) ;
#8476=AXIS2_PLACEMENT_3D ( 'NONE', #35070, #36558, #12293 ) ;
#8477=LINE ( 'NONE', #78390, #55943 ) ;
#8483=DIRECTION ( 'NONE',  ( 0.1857746241280557320, -0.9825923819316327856, 0.000000000000000000 ) ) ;
#8494=CARTESIAN_POINT ( 'NONE',  ( 49.06003799288187395, 95.45573527953635562, 10.00000000000000000 ) ) ;
#8495=CARTESIAN_POINT ( 'NONE',  ( -26.67497870591645537, 34.81099221456150872, 59.99999999999999289 ) ) ;
#8496=VECTOR ( 'NONE', #19471, 1000.000000000000000 ) ;
#8498=DIRECTION ( 'NONE',  ( -0.5000000000000012212, 0.8660254037844379305, -0.000000000000000000 ) ) ;
#8506=DIRECTION ( 'NONE',  ( -0.9762722099447388446, -0.2165469281463391349, 0.000000000000000000 ) ) ;
#8507=EDGE_CURVE ( 'NONE', #25441, #15769, #79721, .T. ) ;
#8510=EDGE_CURVE ( 'NONE', #2857, #10423, #4672, .T. ) ;
#8527=DIRECTION ( 'NONE',  ( -0.1269555777209603886, -0.9919084036772434221, 0.000000000000000000 ) ) ;
#8531=DIRECTION ( 'NONE',  ( 0.000000000000000000, 0.000000000000000000, 1.000000000000000000 ) ) ;
#8546=VECTOR ( 'NONE', #38148, 1000.000000000000000 ) ;
#8547=VECTOR ( 'NONE', #8896, 999.9999999999998863 ) ;
#8548=ORIENTED_EDGE ( 'NONE', *, *, #27020, .T. ) ;
#8553=VECTOR ( 'NONE', #23349, 1000.000000000000000 ) ;
#8556=EDGE_CURVE ( 'NONE', #36369, #43912, #19404, .T. ) ;
#8575=DIRECTION ( 'NONE',  ( -1.000000000000000000, 0.000000000000000000, 0.000000000000000000 ) ) ;
#8578=ORIENTED_EDGE ( 'NONE', *, *, #7083, .T. ) ;
#8579=EDGE_LOOP ( 'NONE', ( #68111, #44555, #69335, #6435 ) ) ;
#8581=CYLINDRICAL_SURFACE ( 'NONE', #30061, 70.00000000000002842 ) ;
#8583=DIRECTION ( 'NONE',  ( 1.000000000000000000, 0.000000000000000000, 0.000000000000000000 ) ) ;
#8587=EDGE_LOOP ( 'NONE', ( #42546, #1569, #55202, #20271 ) ) ;
#8597=EDGE_LOOP ( 'NONE', ( #81403, #71522, #74868, #60209 ) ) ;
#8602=PLANE ( 'NONE',  #80570 ) ;
#8603=CARTESIAN_POINT ( 'NONE',  ( -19.65312891409030271, 93.06504152958497400, 10.00000000000000888 ) ) ;
#8615=FACE_OUTER_BOUND ( 'NONE', #47774, .T. ) ;
#8622=DIRECTION ( 'NONE',  ( -0.000000000000000000, -0.000000000000000000, -1.000000000000000000 ) ) ;
#8627=DIRECTION ( 'NONE',  ( -0.4552093898365321412, 0.8903844177683323258, 0.000000000000000000 ) ) ;
#8628=VERTEX_POINT ( 'NONE', #41155 ) ;
#8630=CARTESIAN_POINT ( 'NONE',  ( -62.95439910331221256, 68.06504152958493137, 60.00000000000000000 ) ) ;
#8633=DIRECTION ( 'NONE',  ( -0.8917477921037005872, -0.4525327339300165286, 0.000000000000000000 ) ) ;
#8648=DIRECTION ( 'NONE',  ( -1.000000000000000000, 0.000000000000000000, 0.000000000000000000 ) ) ;
#8650=CARTESIAN_POINT ( 'NONE',  ( -19.53857018403403956, 92.98143509436215481, 59.99999999999999289 ) ) ;
#8652=PLANE ( 'NONE',  #95773 ) ;
#8657=ORIENTED_EDGE ( 'NONE', *, *, #42942, .F. ) ;
#8662=ORIENTED_EDGE ( 'NONE', *, *, #16471, .F. ) ;
#8674=EDGE_LOOP ( 'NONE', ( #19926, #40194, #28069, #5331 ) ) ;
#8682=CIRCLE ( 'NONE', #5444, 0.1418229129684228651 ) ;
#8683=EDGE_LOOP ( 'NONE', ( #34598, #94985, #15901, #4207 ) ) ;
#8689=LINE ( 'NONE', #22390, #57963 ) ;
#8691=ORIENTED_EDGE ( 'NONE', *, *, #61102, .T. ) ;
#8694=LINE ( 'NONE', #10206, #100082 ) ;
#8702=VERTEX_POINT ( 'NONE', #48491 ) ;
#8715=VERTEX_POINT ( 'NONE', #79432 ) ;
#8718=LINE ( 'NONE', #61897, #78669 ) ;
#8723=ORIENTED_EDGE ( 'NONE', *, *, #33511, .F. ) ;
#8726=DIRECTION ( 'NONE',  ( -0.000000000000000000, 0.000000000000000000, 1.000000000000000000 ) ) ;
#8733=ADVANCED_FACE ( 'NONE', ( #40859 ), #2402, .F. ) ;
#8735=VERTEX_POINT ( 'NONE', #57570 ) ;
#8752=PLANE ( 'NONE',  #67799 ) ;
#8762=ORIENTED_EDGE ( 'NONE', *, *, #87455, .T. ) ;
#8763=CIRCLE ( 'NONE', #58923, 70.00000000000001421 ) ;
#8766=CARTESIAN_POINT ( 'NONE',  ( -12.48997110076107830, 41.83172881028752954, 59.99999999999999289 ) ) ;
#8785=CARTESIAN_POINT ( 'NONE',  ( 49.04287251715432916, 95.72274150194785136, -10.00000000000000000 ) ) ;
#8789=CARTESIAN_POINT ( 'NONE',  ( 43.63646518856938172, 66.22046553916848666, -10.00000000000000000 ) ) ;
#8791=ORIENTED_EDGE ( 'NONE', *, *, #11979, .T. ) ;
#8794=ORIENTED_EDGE ( 'NONE', *, *, #68953, .F. ) ;
#8795=EDGE_CURVE ( 'NONE', #65497, #57017, #2867, .T. ) ;
#8806=DIRECTION ( 'NONE',  ( 0.000000000000000000, 0.000000000000000000, 1.000000000000000000 ) ) ;
#8826=ORIENTED_EDGE ( 'NONE', *, *, #61576, .F. ) ;
#8830=DIRECTION ( 'NONE',  ( -0.3077152132536331575, -0.9514785060800222682, 0.000000000000000000 ) ) ;
#8843=DIRECTION ( 'NONE',  ( -0.9303772761487930643, -0.3666034970181715757, 0.000000000000000000 ) ) ;
#8852=DIRECTION ( 'NONE',  ( 1.000000000000000000, 0.000000000000000000, 0.000000000000000000 ) ) ;
#8854=EDGE_CURVE ( 'NONE', #41771, #52454, #40242, .T. ) ;
#8855=LINE ( 'NONE', #61548, #61490 ) ;
#8862=VERTEX_POINT ( 'NONE', #86423 ) ;
#8863=EDGE_CURVE ( 'NONE', #15769, #40576, #54952, .T. ) ;
#8866=AXIS2_PLACEMENT_3D ( 'NONE', #60202, #29826, #67323 ) ;
#8875=CARTESIAN_POINT ( 'NONE',  ( -25.04755574468712354, 23.27320705613571050, 177.5919119679930134 ) ) ;
#8878=CARTESIAN_POINT ( 'NONE',  ( -4.731736819106161285, 24.67387208536691290, 177.5919119679930134 ) ) ;
#8879=EDGE_CURVE ( 'NONE', #70239, #7803, #28795, .T. ) ;
#8896=DIRECTION ( 'NONE',  ( -0.5104483989331149996, -0.8599083858334093389, 0.000000000000000000 ) ) ;
#8902=AXIS2_PLACEMENT_3D ( 'NONE', #96080, #18550, #34237 ) ;
#8903=DIRECTION ( 'NONE',  ( -0.06442261589618514250, -0.9979227057047518334, 0.000000000000000000 ) ) ;
#8908=CARTESIAN_POINT ( 'NONE',  ( 42.65610334793076674, 64.00004027534475881, -10.00000000000000000 ) ) ;
#8921=ADVANCED_FACE ( 'NONE', ( #35152 ), #58446, .F. ) ;
#8929=CARTESIAN_POINT ( 'NONE',  ( 47.84007798744509898, 106.1754093786579318, -10.00000000000000000 ) ) ;
#8932=ORIENTED_EDGE ( 'NONE', *, *, #16727, .F. ) ;
#8935=ORIENTED_EDGE ( 'NONE', *, *, #42370, .T. ) ;
#8936=CARTESIAN_POINT ( 'NONE',  ( -52.33464467766007289, 32.58262665401804270, -10.00000000000000000 ) ) ;
#8939=DIRECTION ( 'NONE',  ( 0.000000000000000000, 0.000000000000000000, 1.000000000000000000 ) ) ;
#8947=VERTEX_POINT ( 'NONE', #56949 ) ;
#8948=AXIS2_PLACEMENT_3D ( 'NONE', #51727, #50703, #82670 ) ;
#8950=ORIENTED_EDGE ( 'NONE', *, *, #90749, .F. ) ;
#8953=CARTESIAN_POINT ( 'NONE',  ( 11.47080329375824981, 30.07510926853015221, -10.00000000000000000 ) ) ;
#8960=EDGE_LOOP ( 'NONE', ( #97277, #84475, #91819, #20163 ) ) ;
#8977=CARTESIAN_POINT ( 'NONE',  ( 44.35815684012577265, 67.96982248125696913, 10.00000000000000000 ) ) ;
#8978=VECTOR ( 'NONE', #8082, 1000.000000000000114 ) ;
#8988=EDGE_CURVE ( 'NONE', #65735, #30076, #3774, .T. ) ;
#9012=AXIS2_PLACEMENT_3D ( 'NONE', #14594, #61172, #31760 ) ;
#9023=CIRCLE ( 'NONE', #63983, 70.00000000000001421 ) ;
#9038=DIRECTION ( 'NONE',  ( -1.000000000000000000, 0.000000000000000000, 0.000000000000000000 ) ) ;
#9039=EDGE_CURVE ( 'NONE', #56147, #54118, #4773, .T. ) ;
#9048=CARTESIAN_POINT ( 'NONE',  ( -12.63042782814763143, 41.81209092917440273, 59.99999999999999289 ) ) ;
#9056=EDGE_LOOP ( 'NONE', ( #35442, #73136, #28121, #69613 ) ) ;
#9061=DIRECTION ( 'NONE',  ( -0.000000000000000000, -0.000000000000000000, 1.000000000000000000 ) ) ;
#9072=DIRECTION ( 'NONE',  ( 0.000000000000000000, 0.000000000000000000, -1.000000000000000000 ) ) ;
#9074=ORIENTED_EDGE ( 'NONE', *, *, #59634, .F. ) ;
#9077=ORIENTED_EDGE ( 'NONE', *, *, #57001, .F. ) ;
#9088=EDGE_CURVE ( 'NONE', #37455, #99166, #1534, .T. ) ;
#9091=LINE ( 'NONE', #22794, #28981 ) ;
#9096=DIRECTION ( 'NONE',  ( 0.000000000000000000, 0.000000000000000000, 1.000000000000000000 ) ) ;
#9097=CARTESIAN_POINT ( 'NONE',  ( -75.14068524134967220, 52.46521621197197760, 10.00000000000000000 ) ) ;
#9100=VECTOR ( 'NONE', #96967, 1000.000000000000114 ) ;
#9104=CARTESIAN_POINT ( 'NONE',  ( 48.17894221477870786, 74.75545800895066861, 10.00000000000000000 ) ) ;
#9113=AXIS2_PLACEMENT_3D ( 'NONE', #79901, #33784, #57043 ) ;
#9121=DIRECTION ( 'NONE',  ( 1.000000000000000000, 0.000000000000000000, 0.000000000000000000 ) ) ;
#9122=VECTOR ( 'NONE', #4989, 1000.000000000000227 ) ;
#9123=DIRECTION ( 'NONE',  ( -0.8917477921037005872, -0.4525327339300165286, 0.000000000000000000 ) ) ;
#9144=DIRECTION ( 'NONE',  ( -0.000000000000000000, -0.000000000000000000, -1.000000000000000000 ) ) ;
#9148=PLANE ( 'NONE',  #94163 ) ;
#9160=ORIENTED_EDGE ( 'NONE', *, *, #57691, .F. ) ;
#9175=DIRECTION ( 'NONE',  ( -0.9724945078367508433, -0.2329258084183800648, 0.000000000000000000 ) ) ;
#9181=DIRECTION ( 'NONE',  ( 0.000000000000000000, 0.000000000000000000, 1.000000000000000000 ) ) ;
#9185=ORIENTED_EDGE ( 'NONE', *, *, #44566, .T. ) ;
#9187=CARTESIAN_POINT ( 'NONE',  ( 45.98627256186106393, 118.1229683434676900, 10.00000000000000000 ) ) ;
#9197=AXIS2_PLACEMENT_3D ( 'NONE', #82028, #98200, #67273 ) ;
#9199=EDGE_LOOP ( 'NONE', ( #6033, #44341, #80743, #37000 ) ) ;
#9200=DIRECTION ( 'NONE',  ( -0.000000000000000000, -0.000000000000000000, 1.000000000000000000 ) ) ;
#9218=DIRECTION ( 'NONE',  ( 0.000000000000000000, 0.000000000000000000, 1.000000000000000000 ) ) ;
#9232=CARTESIAN_POINT ( 'NONE',  ( 37.48526053816526371, 54.83666944042810343, 10.00000000000000000 ) ) ;
#9237=ORIENTED_EDGE ( 'NONE', *, *, #87798, .F. ) ;
#9238=CARTESIAN_POINT ( 'NONE',  ( 15.54467260552930341, 34.00295985972733348, -10.00000000000000000 ) ) ;
#9242=CARTESIAN_POINT ( 'NONE',  ( -19.65312891409030271, 93.06504152958497400, 177.5919119679930134 ) ) ;
#9243=LINE ( 'NONE', #7231, #43383 ) ;
#9250=VECTOR ( 'NONE', #75810, 1000.000000000000227 ) ;
#9254=EDGE_CURVE ( 'NONE', #46305, #94453, #18722, .T. ) ;
#9261=LINE ( 'NONE', #40132, #27074 ) ;
#9262=DIRECTION ( 'NONE',  ( 0.2165469281463284212, -0.9762722099447411761, 0.000000000000000000 ) ) ;
#9263=FACE_OUTER_BOUND ( 'NONE', #29365, .T. ) ;
#9269=VERTEX_POINT ( 'NONE', #89658 ) ;
#9276=DIRECTION ( 'NONE',  ( -1.000000000000000000, 0.000000000000000000, 0.000000000000000000 ) ) ;
#9286=CARTESIAN_POINT ( 'NONE',  ( -51.65147001822730033, 102.0443063789018652, -10.00000000000000000 ) ) ;
#9290=DIRECTION ( 'NONE',  ( 0.000000000000000000, -0.000000000000000000, 1.000000000000000000 ) ) ;
#9291=DIRECTION ( 'NONE',  ( -0.9919422576440838357, -0.1266907948509199411, 0.000000000000000000 ) ) ;
#9294=EDGE_LOOP ( 'NONE', ( #42218, #78268, #24274, #871 ) ) ;
#9296=PLANE ( 'NONE',  #98850 ) ;
#9298=ORIENTED_EDGE ( 'NONE', *, *, #99162, .T. ) ;
#9299=DIRECTION ( 'NONE',  ( -0.9825923819316306762, -0.1857746241280658628, 0.000000000000000000 ) ) ;
#9301=EDGE_LOOP ( 'NONE', ( #9077, #8434, #92845, #50816 ) ) ;
#9309=CARTESIAN_POINT ( 'NONE',  ( -19.65312891409030271, 93.06504152958497400, -10.00000000000000888 ) ) ;
#9310=VECTOR ( 'NONE', #51888, 999.9999999999998863 ) ;
#9321=AXIS2_PLACEMENT_3D ( 'NONE', #37875, #22705, #75416 ) ;
#9324=EDGE_CURVE ( 'NONE', #45024, #15783, #11136, .T. ) ;
#9326=CARTESIAN_POINT ( 'NONE',  ( -25.04755574468711643, 23.27320705613571761, 10.00000000000000000 ) ) ;
#9327=DIRECTION ( 'NONE',  ( -1.000000000000000000, 0.000000000000000000, 0.000000000000000000 ) ) ;
#9328=AXIS2_PLACEMENT_3D ( 'NONE', #95708, #9570, #79991 ) ;
#9329=DIRECTION ( 'NONE',  ( 0.6363689690731033632, 0.7713848165480284846, 0.000000000000000000 ) ) ;
#9335=AXIS2_PLACEMENT_3D ( 'NONE', #66874, #20296, #19805 ) ;
#9350=CARTESIAN_POINT ( 'NONE',  ( -48.47243291925848752, 30.64988553008148031, -10.00000000000000000 ) ) ;
#9355=EDGE_LOOP ( 'NONE', ( #20399, #14686, #45178, #3467 ) ) ;
#9356=VERTEX_POINT ( 'NONE', #44488 ) ;
#9366=VECTOR ( 'NONE', #3076, 1000.000000000000000 ) ;
#9372=VECTOR ( 'NONE', #47441, 1000.000000000000227 ) ;
#9387=CARTESIAN_POINT ( 'NONE',  ( 37.48526053816526371, 54.83666944042810343, -10.00000000000000000 ) ) ;
#9393=CIRCLE ( 'NONE', #91954, 0.1418229129680880773 ) ;
#9401=DIRECTION ( 'NONE',  ( 0.9919084036772433111, -0.1269555777209603886, 0.000000000000000000 ) ) ;
#9403=DIRECTION ( 'NONE',  ( -0.8660254037844379305, -0.5000000000000011102, -0.000000000000000000 ) ) ;
#9408=CARTESIAN_POINT ( 'NONE',  ( -19.65312891409030271, 93.06504152958497400, 59.99999999999999289 ) ) ;
#9411=CIRCLE ( 'NONE', #66041, 70.00000000000001421 ) ;
#9426=DIRECTION ( 'NONE',  ( 1.000000000000000000, 0.000000000000000000, 0.000000000000000000 ) ) ;
#9430=VERTEX_POINT ( 'NONE', #54077 ) ;
#9438=DIRECTION ( 'NONE',  ( -0.8600446134263880493, -0.5102188382608534578, 0.000000000000000000 ) ) ;
#9441=LINE ( 'NONE', #85486, #20695 ) ;
#9448=EDGE_CURVE ( 'NONE', #11831, #18551, #46480, .T. ) ;
#9458=AXIS2_PLACEMENT_3D ( 'NONE', #15664, #8087, #55155 ) ;
#9466=DIRECTION ( 'NONE',  ( -0.000000000000000000, -0.000000000000000000, -1.000000000000000000 ) ) ;
#9470=CARTESIAN_POINT ( 'NONE',  ( 48.58227110419246486, 77.44677708231242264, 177.5919119679930134 ) ) ;
#9472=ORIENTED_EDGE ( 'NONE', *, *, #42849, .F. ) ;
#9487=EDGE_CURVE ( 'NONE', #32467, #10367, #38887, .T. ) ;
#9490=DIRECTION ( 'NONE',  ( 1.000000000000000000, 0.000000000000000000, 0.000000000000000000 ) ) ;
#9496=ADVANCED_FACE ( 'NONE', ( #36281 ), #43875, .F. ) ;
#9504=EDGE_CURVE ( 'NONE', #81911, #98268, #45852, .T. ) ;
#9507=VECTOR ( 'NONE', #97237, 1000.000000000000000 ) ;
#9511=PLANE ( 'NONE',  #19313 ) ;
#9513=EDGE_CURVE ( 'NONE', #67607, #49038, #29197, .T. ) ;
#9515=EDGE_CURVE ( 'NONE', #17295, #56255, #60065, .T. ) ;
#9516=CARTESIAN_POINT ( 'NONE',  ( 46.50192534792603283, 74.36443251879779837, -10.00000000000000000 ) ) ;
#9523=VECTOR ( 'NONE', #84866, 1000.000000000000000 ) ;
#9527=CIRCLE ( 'NONE', #58100, 60.00000000000002132 ) ;
#9530=LINE ( 'NONE', #92648, #42504 ) ;
#9531=VECTOR ( 'NONE', #87413, 1000.000000000000227 ) ;
#9540=DIRECTION ( 'NONE',  ( 0.02977611660965746518, -0.9995565931350001154, 0.000000000000000000 ) ) ;
#9541=VECTOR ( 'NONE', #73604, 1000.000000000000000 ) ;
#9553=EDGE_LOOP ( 'NONE', ( #45729, #11598, #50195, #69957 ) ) ;
#9563=ORIENTED_EDGE ( 'NONE', *, *, #87191, .F. ) ;
#9568=ADVANCED_FACE ( 'NONE', ( #75428 ), #53108, .F. ) ;
#9570=DIRECTION ( 'NONE',  ( -0.000000000000000000, -0.000000000000000000, -1.000000000000000000 ) ) ;
#9572=ORIENTED_EDGE ( 'NONE', *, *, #98923, .T. ) ;
#9573=ORIENTED_EDGE ( 'NONE', *, *, #40056, .T. ) ;
#9576=DIRECTION ( 'NONE',  ( 1.000000000000000000, 0.000000000000000000, 0.000000000000000000 ) ) ;
#9582=CARTESIAN_POINT ( 'NONE',  ( -52.76723787663020460, 95.88936769132961047, -10.00000000000000000 ) ) ;
#9585=VERTEX_POINT ( 'NONE', #98234 ) ;
#9587=CARTESIAN_POINT ( 'NONE',  ( 8.106622824862185439, 30.17147933776455204, -10.00000000000000000 ) ) ;
#9588=CARTESIAN_POINT ( 'NONE',  ( -19.65312891409030271, 93.06504152958497400, 59.99999999999999289 ) ) ;
#9589=VERTEX_POINT ( 'NONE', #67818 ) ;
#9593=CARTESIAN_POINT ( 'NONE',  ( -19.65312891409030271, 93.06504152958497400, 10.00000000000000888 ) ) ;
#9605=AXIS2_PLACEMENT_3D ( 'NONE', #51637, #20748, #53122 ) ;
#9606=ORIENTED_EDGE ( 'NONE', *, *, #7091, .F. ) ;
#9607=VECTOR ( 'NONE', #45303, 1000.000000000000000 ) ;
#9613=EDGE_LOOP ( 'NONE', ( #48193, #75501, #54470, #86242 ) ) ;
#9622=ORIENTED_EDGE ( 'NONE', *, *, #84564, .T. ) ;
#9624=VECTOR ( 'NONE', #54120, 1000.000000000000000 ) ;
#9630=DIRECTION ( 'NONE',  ( -0.2877784213863818774, 0.9576970189910596343, 0.000000000000000000 ) ) ;
#9635=EDGE_CURVE ( 'NONE', #23644, #68477, #83789, .T. ) ;
#9650=DIRECTION ( 'NONE',  ( -0.9932214622066116716, 0.1162373735601425623, 0.000000000000000000 ) ) ;
#9654=DIRECTION ( 'NONE',  ( -0.8756465943326132706, -0.4829524219151362097, 0.000000000000000000 ) ) ;
#9666=DIRECTION ( 'NONE',  ( -0.000000000000000000, -0.000000000000000000, -1.000000000000000000 ) ) ;
#9668=FACE_OUTER_BOUND ( 'NONE', #5609, .T. ) ;
#9676=CARTESIAN_POINT ( 'NONE',  ( 50.34596055286379368, 92.70800680107760172, -10.00000000000000000 ) ) ;
#9686=DIRECTION ( 'NONE',  ( -0.9999580202055560196, -0.009162850352621043637, 0.000000000000000000 ) ) ;
#9690=DIRECTION ( 'NONE',  ( -0.000000000000000000, 0.000000000000000000, 1.000000000000000000 ) ) ;
#9693=CIRCLE ( 'NONE', #12956, 14.99999999999967493 ) ;
#9697=ORIENTED_EDGE ( 'NONE', *, *, #61318, .T. ) ;
#9707=CARTESIAN_POINT ( 'NONE',  ( -19.69918098444705379, 92.93090374423474032, 59.99999999999999289 ) ) ;
#9715=VECTOR ( 'NONE', #15201, 1000.000000000000000 ) ;
#9716=EDGE_CURVE ( 'NONE', #68082, #24137, #40048, .T. ) ;
#9723=DIRECTION ( 'NONE',  ( 0.9981280818701453450, 0.06115825522547521653, 0.000000000000000000 ) ) ;
#9726=LINE ( 'NONE', #26408, #72316 ) ;
#9738=DIRECTION ( 'NONE',  ( 1.000000000000000000, 0.000000000000000000, 0.000000000000000000 ) ) ;
#9740=ORIENTED_EDGE ( 'NONE', *, *, #66562, .F. ) ;
#9747=ORIENTED_EDGE ( 'NONE', *, *, #27443, .T. ) ;
#9773=CARTESIAN_POINT ( 'NONE',  ( -48.41313092940755070, 109.7198701005979302, -10.00000000000000000 ) ) ;
#9783=ORIENTED_EDGE ( 'NONE', *, *, #46979, .F. ) ;
#9792=EDGE_CURVE ( 'NONE', #39443, #96352, #19062, .T. ) ;
#9798=VERTEX_POINT ( 'NONE', #51495 ) ;
#9814=LINE ( 'NONE', #47768, #90489 ) ;
#9815=VERTEX_POINT ( 'NONE', #59577 ) ;
#9828=CARTESIAN_POINT ( 'NONE',  ( -35.89898968889472997, 24.97633462685643124, 10.00000000000000000 ) ) ;
#9834=ORIENTED_EDGE ( 'NONE', *, *, #89614, .T. ) ;
#9837=DIRECTION ( 'NONE',  ( 0.000000000000000000, 0.000000000000000000, 1.000000000000000000 ) ) ;
#9839=EDGE_CURVE ( 'NONE', #38656, #89858, #78934, .T. ) ;
#9843=EDGE_CURVE ( 'NONE', #80773, #11356, #20614, .T. ) ;
#9847=CARTESIAN_POINT ( 'NONE',  ( -50.34886203176066033, 29.86533669878861375, 10.00000000000000000 ) ) ;
#9851=ORIENTED_EDGE ( 'NONE', *, *, #23401, .F. ) ;
#9867=EDGE_CURVE ( 'NONE', #34967, #85106, #91038, .T. ) ;
#9869=DIRECTION ( 'NONE',  ( -1.000000000000000000, -4.892646582057337723E-14, 0.000000000000000000 ) ) ;
#9878=ORIENTED_EDGE ( 'NONE', *, *, #38578, .T. ) ;
#9879=UNCERTAINTY_MEASURE_WITH_UNIT (LENGTH_MEASURE( 1.000000000000000082E-05 ), #84711, 'distance_accuracy_value', 'NONE');
#9884=DIRECTION ( 'NONE',  ( 0.2194785493951409983, -0.9756173257765590190, 0.000000000000000000 ) ) ;
#9895=CARTESIAN_POINT ( 'NONE',  ( 36.25628400652970384, 53.06077264917335867, 10.00000000000000000 ) ) ;
#9907=CARTESIAN_POINT ( 'NONE',  ( 48.32408078245682503, 82.80331927372955647, -10.00000000000000000 ) ) ;
#9909=DIRECTION ( 'NONE',  ( -0.5891075386695773242, -0.8080546441192405505, 0.000000000000000000 ) ) ;
#9923=DIRECTION ( 'NONE',  ( 1.000000000000000000, 0.000000000000000000, 0.000000000000000000 ) ) ;
#9926=EDGE_LOOP ( 'NONE', ( #66352, #68980, #94718, #21660 ) ) ;
#9932=CARTESIAN_POINT ( 'NONE',  ( -19.65312891409034179, 93.06504152958504505, 0.000000000000000000 ) ) ;
#9933=DIRECTION ( 'NONE',  ( -1.000000000000000000, 0.000000000000000000, 0.000000000000000000 ) ) ;
#9940=ORIENTED_EDGE ( 'NONE', *, *, #85926, .F. ) ;
#9958=EDGE_CURVE ( 'NONE', #66829, #65714, #44384, .T. ) ;
#9963=ORIENTED_EDGE ( 'NONE', *, *, #29406, .T. ) ;
#9971=DIRECTION ( 'NONE',  ( 1.000000000000000000, 0.000000000000000000, 0.000000000000000000 ) ) ;
#9977=ORIENTED_EDGE ( 'NONE', *, *, #39458, .F. ) ;
#9981=FACE_OUTER_BOUND ( 'NONE', #79409, .T. ) ;
#9998=CARTESIAN_POINT ( 'NONE',  ( -74.33658418421376268, 48.94984639172533747, -10.00000000000000000 ) ) ;
#10017=EDGE_CURVE ( 'NONE', #61038, #43732, #25762, .T. ) ;
#10037=PLANE ( 'NONE',  #29912 ) ;
#10045=LINE ( 'NONE', #71856, #7709 ) ;
#10052=DIRECTION ( 'NONE',  ( 0.000000000000000000, -0.000000000000000000, 1.000000000000000000 ) ) ;
#10065=DIRECTION ( 'NONE',  ( 0.4525327339300069251, -0.8917477921037054722, 0.000000000000000000 ) ) ;
#10077=ORIENTED_EDGE ( 'NONE', *, *, #78563, .F. ) ;
#10078=VECTOR ( 'NONE', #703, 1000.000000000000000 ) ;
#10089=ORIENTED_EDGE ( 'NONE', *, *, #75425, .T. ) ;
#10090=EDGE_LOOP ( 'NONE', ( #76602, #16388, #28224, #81739 ) ) ;
#10094=CARTESIAN_POINT ( 'NONE',  ( -4.170157060006060235, 26.08383846222962887, 10.00000000000000000 ) ) ;
#10098=ORIENTED_EDGE ( 'NONE', *, *, #87110, .F. ) ;
#10108=CARTESIAN_POINT ( 'NONE',  ( 42.65610334793076674, 64.00004027534475881, -10.00000000000000000 ) ) ;
#10113=EDGE_LOOP ( 'NONE', ( #31331, #22240, #86098, #30978 ) ) ;
#10114=CARTESIAN_POINT ( 'NONE',  ( 38.68775240272602645, 99.32300362076651368, 59.99999999999999289 ) ) ;
#10115=ADVANCED_FACE ( 'NONE', ( #782 ), #1297, .F. ) ;
#10119=EDGE_CURVE ( 'NONE', #83740, #21633, #16485, .T. ) ;
#10123=CARTESIAN_POINT ( 'NONE',  ( -61.61048871844075592, 38.59675092633816007, 10.00000000000000000 ) ) ;
#10124=DIRECTION ( 'NONE',  ( -0.000000000000000000, -0.000000000000000000, -1.000000000000000000 ) ) ;
#10126=CARTESIAN_POINT ( 'NONE',  ( 2.064617007569734319, 27.83817977871672511, -10.00000000000000000 ) ) ;
#10136=VECTOR ( 'NONE', #65571, 1000.000000000000000 ) ;
#10137=AXIS2_PLACEMENT_3D ( 'NONE', #55969, #78817, #72736 ) ;
#10147=VECTOR ( 'NONE', #99506, 1000.000000000000000 ) ;
#10150=ADVANCED_FACE ( 'NONE', ( #62564 ), #85438, .T. ) ;
#10157=CARTESIAN_POINT ( 'NONE',  ( -5.552095647868114270, 82.17113873493018161, 13.38795332614766309 ) ) ;
#10160=ORIENTED_EDGE ( 'NONE', *, *, #34297, .F. ) ;
#10161=CIRCLE ( 'NONE', #23075, 0.1418229129680828593 ) ;
#10169=VERTEX_POINT ( 'NONE', #46887 ) ;
#10173=FACE_OUTER_BOUND ( 'NONE', #34481, .T. ) ;
#10175=VERTEX_POINT ( 'NONE', #9907 ) ;
#10180=VERTEX_POINT ( 'NONE', #47868 ) ;
#10181=VERTEX_POINT ( 'NONE', #78805 ) ;
#10184=( NAMED_UNIT ( * ) SI_UNIT ( $, .STERADIAN. ) SOLID_ANGLE_UNIT ( ) );
#10187=DIRECTION ( 'NONE',  ( -0.4831861483251663203, -0.8755176446346986108, 0.000000000000000000 ) ) ;
#10191=ADVANCED_FACE ( 'NONE', ( #61577 ), #86953, .F. ) ;
#10206=CARTESIAN_POINT ( 'NONE',  ( 1.764981905019474828, 67.65273034797039031, -10.00000000000000000 ) ) ;
#10222=PLANE ( 'NONE',  #83643 ) ;
#10228=DIRECTION ( 'NONE',  ( -0.8082118706970123911, -0.5888918169447047157, 0.000000000000000000 ) ) ;
#10236=CARTESIAN_POINT ( 'NONE',  ( 42.87860686303043423, 124.5258428655388769, 177.5919119679930134 ) ) ;
#10261=DIRECTION ( 'NONE',  ( -0.9042435392811277728, -0.4270171210482543445, 0.000000000000000000 ) ) ;
#10268=EDGE_CURVE ( 'NONE', #59479, #35906, #4782, .T. ) ;
#10271=EDGE_CURVE ( 'NONE', #28238, #40468, #33706, .T. ) ;
#10285=DIRECTION ( 'NONE',  ( 0.000000000000000000, 0.000000000000000000, 1.000000000000000000 ) ) ;
#10293=ORIENTED_EDGE ( 'NONE', *, *, #15197, .F. ) ;
#10296=LINE ( 'NONE', #33088, #46090 ) ;
#10300=ORIENTED_EDGE ( 'NONE', *, *, #63793, .T. ) ;
#10302=DIRECTION ( 'NONE',  ( 0.000000000000000000, 0.000000000000000000, 1.000000000000000000 ) ) ;
#10303=VECTOR ( 'NONE', #2317, 1000.000000000000000 ) ;
#10310=CARTESIAN_POINT ( 'NONE',  ( -10.80656490723494123, 24.88181024604956804, 10.00000000000000000 ) ) ;
#10311=VECTOR ( 'NONE', #654, 1000.000000000000114 ) ;
#10313=DIRECTION ( 'NONE',  ( 0.9994538543569184696, -0.03304531753667278721, 0.000000000000000000 ) ) ;
#10318=CARTESIAN_POINT ( 'NONE',  ( 42.76202708541288899, 64.24573752441608576, 10.00000000000000000 ) ) ;
#10319=LINE ( 'NONE', #26024, #94712 ) ;
#10322=EDGE_CURVE ( 'NONE', #60097, #48601, #19521, .T. ) ;
#10324=CARTESIAN_POINT ( 'NONE',  ( -10.54235908185773418, 24.92402704602492847, -10.00000000000000000 ) ) ;
#10326=ORIENTED_EDGE ( 'NONE', *, *, #9487, .T. ) ;
#10337=DIRECTION ( 'NONE',  ( 0.000000000000000000, 0.000000000000000000, 1.000000000000000000 ) ) ;
#10338=CARTESIAN_POINT ( 'NONE',  ( -19.65312891409030271, 93.06504152958497400, -10.00000000000000888 ) ) ;
#10339=ORIENTED_EDGE ( 'NONE', *, *, #28353, .T. ) ;
#10344=CARTESIAN_POINT ( 'NONE',  ( -47.78078991586326651, 28.96484896693080913, 10.00000000000000000 ) ) ;
#10350=CARTESIAN_POINT ( 'NONE',  ( 10.35730516091175701, 49.35094346172001423, 59.99999999999999289 ) ) ;
#10358=CARTESIAN_POINT ( 'NONE',  ( -40.42249077443059235, 27.53003111760058630, -10.00000000000000000 ) ) ;
#10359=EDGE_CURVE ( 'NONE', #22179, #32899, #66088, .T. ) ;
#10367=VERTEX_POINT ( 'NONE', #49389 ) ;
#10382=EDGE_CURVE ( 'NONE', #8334, #67265, #97034, .T. ) ;
#10404=ORIENTED_EDGE ( 'NONE', *, *, #7917, .F. ) ;
#10411=FACE_OUTER_BOUND ( 'NONE', #10804, .T. ) ;
#10423=VERTEX_POINT ( 'NONE', #83816 ) ;
#10433=CARTESIAN_POINT ( 'NONE',  ( -45.72565977301701423, 72.45571923938835823, -10.00000000000000000 ) ) ;
#10435=ORIENTED_EDGE ( 'NONE', *, *, #49730, .T. ) ;
#10440=AXIS2_PLACEMENT_3D ( 'NONE', #96147, #27217, #2942 ) ;
#10444=ORIENTED_EDGE ( 'NONE', *, *, #81227, .T. ) ;
#10451=AXIS2_PLACEMENT_3D ( 'NONE', #32928, #63832, #95790 ) ;
#10454=ORIENTED_EDGE ( 'NONE', *, *, #41133, .F. ) ;
#10466=DIRECTION ( 'NONE',  ( -0.8143688203140631021, 0.5803476755362091399, 0.000000000000000000 ) ) ;
#10468=FACE_OUTER_BOUND ( 'NONE', #40606, .T. ) ;
#10471=CARTESIAN_POINT ( 'NONE',  ( -19.65312891409030271, 93.06504152958497400, 10.00000000000000888 ) ) ;
#10473=VERTEX_POINT ( 'NONE', #43266 ) ;
#10479=CARTESIAN_POINT ( 'NONE',  ( 22.96769398916923777, 37.53608102203546792, -10.00000000000000000 ) ) ;
#10481=FACE_OUTER_BOUND ( 'NONE', #20029, .T. ) ;
#10493=FACE_OUTER_BOUND ( 'NONE', #72429, .T. ) ;
#10505=VECTOR ( 'NONE', #41595, 1000.000000000000114 ) ;
#10512=EDGE_CURVE ( 'NONE', #78854, #81228, #37655, .T. ) ;
#10516=VECTOR ( 'NONE', #18118, 1000.000000000000000 ) ;
#10519=DIRECTION ( 'NONE',  ( -1.000000000000000000, 0.000000000000000000, 0.000000000000000000 ) ) ;
#10525=FACE_OUTER_BOUND ( 'NONE', #41837, .T. ) ;
#10533=ORIENTED_EDGE ( 'NONE', *, *, #97782, .F. ) ;
#10547=ORIENTED_EDGE ( 'NONE', *, *, #63113, .T. ) ;
#10548=LINE ( 'NONE', #65720, #48362 ) ;
#10550=LINE ( 'NONE', #95701, #3741 ) ;
#10555=AXIS2_PLACEMENT_3D ( 'NONE', #9408, #17504, #57490 ) ;
#10560=CYLINDRICAL_SURFACE ( 'NONE', #4465, 70.00000000000002842 ) ;
#10561=EDGE_LOOP ( 'NONE', ( #82408, #57906, #86639, #7103 ) ) ;
#10562=ORIENTED_EDGE ( 'NONE', *, *, #27206, .F. ) ;
#10575=ORIENTED_EDGE ( 'NONE', *, *, #46602, .T. ) ;
#10576=DIRECTION ( 'NONE',  ( -0.000000000000000000, 0.000000000000000000, -1.000000000000000000 ) ) ;
#10579=VERTEX_POINT ( 'NONE', #28574 ) ;
#10589=ORIENTED_EDGE ( 'NONE', *, *, #82041, .F. ) ;
#10590=VECTOR ( 'NONE', #44667, 1000.000000000000000 ) ;
#10593=EDGE_CURVE ( 'NONE', #4283, #49899, #22473, .T. ) ;
#10618=CIRCLE ( 'NONE', #51026, 11.89249999999999652 ) ;
#10627=DIRECTION ( 'NONE',  ( -0.000000000000000000, -0.000000000000000000, 1.000000000000000000 ) ) ;
#10629=VECTOR ( 'NONE', #69501, 1000.000000000000114 ) ;
#10638=LINE ( 'NONE', #56722, #37010 ) ;
#10639=DIRECTION ( 'NONE',  ( -0.7911563084720435457, -0.6116140086401625764, 0.000000000000000000 ) ) ;
#10649=CARTESIAN_POINT ( 'NONE',  ( 3.113790753877909712, 26.87087736965101570, 10.00000000000000000 ) ) ;
#10653=CARTESIAN_POINT ( 'NONE',  ( -36.26652983198114555, 26.35523046909639788, -10.00000000000000000 ) ) ;
#10657=CARTESIAN_POINT ( 'NONE',  ( -5.341514567247151568, 81.77868734245731730, 13.39505696618104302 ) ) ;
#10660=ORIENTED_EDGE ( 'NONE', *, *, #93453, .F. ) ;
#10682=VERTEX_POINT ( 'NONE', #78689 ) ;
#10691=CIRCLE ( 'NONE', #28460, 50.00000000000000711 ) ;
#10692=EDGE_CURVE ( 'NONE', #98414, #77450, #66245, .T. ) ;
#10699=EDGE_CURVE ( 'NONE', #14070, #29175, #41940, .T. ) ;
#10709=DIRECTION ( 'NONE',  ( -0.8600446134263897147, -0.5102188382608503492, 0.000000000000000000 ) ) ;
#10724=CIRCLE ( 'NONE', #83497, 70.00000000000001421 ) ;
#10726=DIRECTION ( 'NONE',  ( 0.000000000000000000, 0.000000000000000000, 1.000000000000000000 ) ) ;
#10728=EDGE_CURVE ( 'NONE', #71229, #84849, #96910, .T. ) ;
#10729=VECTOR ( 'NONE', #70029, 1000.000000000000227 ) ;
#10740=LINE ( 'NONE', #3645, #74192 ) ;
#10750=FACE_OUTER_BOUND ( 'NONE', #57380, .T. ) ;
#10754=ORIENTED_EDGE ( 'NONE', *, *, #16214, .F. ) ;
#10763=DIRECTION ( 'NONE',  ( 0.000000000000000000, -0.000000000000000000, 1.000000000000000000 ) ) ;
#10769=CARTESIAN_POINT ( 'NONE',  ( -19.65312891409030271, 93.06504152958497400, 10.00000000000000888 ) ) ;
#10776=DIRECTION ( 'NONE',  ( 0.000000000000000000, 0.000000000000000000, 1.000000000000000000 ) ) ;
#10780=CARTESIAN_POINT ( 'NONE',  ( -74.33658418421376268, 48.94984639172533747, 10.00000000000000000 ) ) ;
#10785=DIRECTION ( 'NONE',  ( -0.1239754375649672058, -0.9922852870422774751, 0.000000000000000000 ) ) ;
#10792=CIRCLE ( 'NONE', #23694, 70.00000000000001421 ) ;
#10793=LINE ( 'NONE', #3696, #64571 ) ;
#10794=CIRCLE ( 'NONE', #83564, 70.00000000000001421 ) ;
#10804=EDGE_LOOP ( 'NONE', ( #67134, #91478, #90398, #20320 ) ) ;
#10805=CARTESIAN_POINT ( 'NONE',  ( 30.84500111113854004, 63.18596212086494290, 59.99999999999999289 ) ) ;
#10807=ORIENTED_EDGE ( 'NONE', *, *, #38391, .F. ) ;
#10813=CARTESIAN_POINT ( 'NONE',  ( 43.35468487962021555, 120.5828561944265687, -10.00000000000000000 ) ) ;
#10815=ORIENTED_EDGE ( 'NONE', *, *, #56923, .T. ) ;
#10821=DIRECTION ( 'NONE',  ( -0.9874733399847778204, -0.1577859398657163181, 0.000000000000000000 ) ) ;
#10822=ORIENTED_EDGE ( 'NONE', *, *, #48500, .F. ) ;
#10826=CARTESIAN_POINT ( 'NONE',  ( 49.07456115661582174, 91.13648234292965356, 10.00000000000000000 ) ) ;
#10832=EDGE_CURVE ( 'NONE', #21633, #81790, #98376, .T. ) ;
#10833=DIRECTION ( 'NONE',  ( -0.000000000000000000, -0.000000000000000000, -1.000000000000000000 ) ) ;
#10835=VERTEX_POINT ( 'NONE', #13749 ) ;
#10843=ORIENTED_EDGE ( 'NONE', *, *, #17691, .T. ) ;
#10844=CIRCLE ( 'NONE', #57740, 0.1418229129684298040 ) ;
#10850=CARTESIAN_POINT ( 'NONE',  ( 25.98835327777827686, 41.64452202306098627, -10.00000000000000000 ) ) ;
#10851=EDGE_CURVE ( 'NONE', #34369, #74676, #35497, .T. ) ;
#10854=EDGE_LOOP ( 'NONE', ( #26739, #88446, #95814, #1454 ) ) ;
#10856=AXIS2_PLACEMENT_3D ( 'NONE', #59281, #90260, #20830 ) ;
#10859=VECTOR ( 'NONE', #20112, 1000.000000000000114 ) ;
#10868=ORIENTED_EDGE ( 'NONE', *, *, #66377, .T. ) ;
#10870=ORIENTED_EDGE ( 'NONE', *, *, #37336, .T. ) ;
#10876=EDGE_CURVE ( 'NONE', #78230, #64662, #38022, .T. ) ;
#10880=ORIENTED_EDGE ( 'NONE', *, *, #93051, .F. ) ;
#10882=EDGE_CURVE ( 'NONE', #96562, #91318, #68933, .T. ) ;
#10883=EDGE_CURVE ( 'NONE', #20265, #19444, #24349, .T. ) ;
#10897=CARTESIAN_POINT ( 'NONE',  ( -71.61465314115659453, 63.06504152958490295, 203.6502102582797420 ) ) ;
#10905=LINE ( 'NONE', #72727, #21490 ) ;
#10907=VERTEX_POINT ( 'NONE', #7642 ) ;
#10914=ORIENTED_EDGE ( 'NONE', *, *, #90879, .T. ) ;
#10940=AXIS2_PLACEMENT_3D ( 'NONE', #40598, #71536, #78634 ) ;
#10945=ORIENTED_EDGE ( 'NONE', *, *, #59166, .T. ) ;
#10946=ORIENTED_EDGE ( 'NONE', *, *, #17964, .T. ) ;
#10955=VECTOR ( 'NONE', #26355, 1000.000000000000114 ) ;
#10961=LINE ( 'NONE', #33238, #87412 ) ;
#10968=ORIENTED_EDGE ( 'NONE', *, *, #80428, .T. ) ;
#10971=CARTESIAN_POINT ( 'NONE',  ( 13.67211979723576931, 32.92651376809308772, -10.00000000000000000 ) ) ;
#10974=CARTESIAN_POINT ( 'NONE',  ( -71.61465314115659453, 63.06504152958490295, -40.00000000000000711 ) ) ;
#10982=CARTESIAN_POINT ( 'NONE',  ( 15.77038241084232517, 34.14663330942826747, 10.00000000000000000 ) ) ;
#10983=ORIENTED_EDGE ( 'NONE', *, *, #13269, .T. ) ;
#10989=CARTESIAN_POINT ( 'NONE',  ( -19.65312891409030271, 93.06504152958497400, 59.99999999999999289 ) ) ;
#10993=VECTOR ( 'NONE', #26656, 1000.000000000000000 ) ;
#10995=CARTESIAN_POINT ( 'NONE',  ( 42.76202708541288899, 64.24573752441608576, -10.00000000000000000 ) ) ;
#10997=CARTESIAN_POINT ( 'NONE',  ( -18.15312891409030627, 78.77562236714182120, 52.49999999999999289 ) ) ;
#10999=CIRCLE ( 'NONE', #38427, 70.00000000000001421 ) ;
#11001=DIRECTION ( 'NONE',  ( -0.6384778167143363437, 0.7696402260561061581, 0.000000000000000000 ) ) ;
#11003=DIRECTION ( 'NONE',  ( -0.2575544297740129385, 0.9662637919863205083, 0.000000000000000000 ) ) ;
#11015=LINE ( 'NONE', #42373, #81487 ) ;
#11018=FACE_OUTER_BOUND ( 'NONE', #49428, .T. ) ;
#11027=DIRECTION ( 'NONE',  ( -0.9946578707245747886, -0.1032265479692855564, 0.000000000000000000 ) ) ;
#11030=EDGE_CURVE ( 'NONE', #43292, #8402, #65223, .T. ) ;
#11042=DIRECTION ( 'NONE',  ( 0.000000000000000000, -0.000000000000000000, -1.000000000000000000 ) ) ;
#11055=DIRECTION ( 'NONE',  ( 1.000000000000000000, 0.000000000000000000, 0.000000000000000000 ) ) ;
#11056=VERTEX_POINT ( 'NONE', #28215 ) ;
#11057=CARTESIAN_POINT ( 'NONE',  ( 1.023347710557721113, 26.18841396516314646, -10.00000000000000000 ) ) ;
#11063=AXIS2_PLACEMENT_3D ( 'NONE', #80681, #74039, #58315 ) ;
#11064=EDGE_LOOP ( 'NONE', ( #22865, #36521, #70219, #25050 ) ) ;
#11068=CARTESIAN_POINT ( 'NONE',  ( -32.04500338604975695, 25.44370296803429810, -10.00000000000000000 ) ) ;
#11073=CARTESIAN_POINT ( 'NONE',  ( 40.82928596147627331, 60.38352576601455723, -10.00000000000000000 ) ) ;
#11090=VERTEX_POINT ( 'NONE', #57611 ) ;
#11094=FACE_OUTER_BOUND ( 'NONE', #21180, .T. ) ;
#11096=EDGE_CURVE ( 'NONE', #35869, #75897, #34808, .T. ) ;
#11100=EDGE_CURVE ( 'NONE', #84216, #83863, #42404, .T. ) ;
#11101=AXIS2_PLACEMENT_3D ( 'NONE', #42422, #57628, #35334 ) ;
#11105=ADVANCED_FACE ( 'NONE', ( #95688 ), #4940, .F. ) ;
#11107=EDGE_CURVE ( 'NONE', #75907, #20062, #8028, .T. ) ;
#11123=CARTESIAN_POINT ( 'NONE',  ( -19.65312891409030271, 93.06504152958497400, 177.5919119679930134 ) ) ;
#11126=CARTESIAN_POINT ( 'NONE',  ( -3.216670782107629911, 25.02209300385174373, 10.00000000000000000 ) ) ;
#11132=AXIS2_PLACEMENT_3D ( 'NONE', #66020, #10833, #4732 ) ;
#11136=LINE ( 'NONE', #51089, #90303 ) ;
#11144=VECTOR ( 'NONE', #5905, 999.9999999999998863 ) ;
#11147=DIRECTION ( 'NONE',  ( 0.000000000000000000, 0.000000000000000000, 1.000000000000000000 ) ) ;
#11154=EDGE_CURVE ( 'NONE', #90765, #41961, #66713, .T. ) ;
#11155=VECTOR ( 'NONE', #1281, 1000.000000000000114 ) ;
#11170=ORIENTED_EDGE ( 'NONE', *, *, #29935, .T. ) ;
#11171=CARTESIAN_POINT ( 'NONE',  ( -7.323307257743949528, 84.15769153094232990, 13.64793647583705294 ) ) ;
#11175=EDGE_LOOP ( 'NONE', ( #78678, #26737, #85639, #24474 ) ) ;
#11178=FACE_OUTER_BOUND ( 'NONE', #26047, .T. ) ;
#11181=CARTESIAN_POINT ( 'NONE',  ( -69.85371643402891095, 44.28081239092799848, -10.00000000000000000 ) ) ;
#11190=CARTESIAN_POINT ( 'NONE',  ( -19.65312891409030271, 93.06504152958497400, 203.6502102582797420 ) ) ;
#11198=CARTESIAN_POINT ( 'NONE',  ( 41.71240375114938814, 62.05720181600818108, 10.00000000000000000 ) ) ;
#11199=VECTOR ( 'NONE', #47948, 1000.000000000000000 ) ;
#11205=AXIS2_PLACEMENT_3D ( 'NONE', #87615, #72365, #11055 ) ;
#11209=ORIENTED_EDGE ( 'NONE', *, *, #82172, .T. ) ;
#11213=FACE_BOUND ( 'NONE', #49786, .T. ) ;
#11218=DIRECTION ( 'NONE',  ( 0.000000000000000000, 0.000000000000000000, 1.000000000000000000 ) ) ;
#11224=ORIENTED_EDGE ( 'NONE', *, *, #54772, .T. ) ;
#11228=EDGE_CURVE ( 'NONE', #92184, #79500, #20632, .T. ) ;
#11240=ORIENTED_EDGE ( 'NONE', *, *, #12101, .T. ) ;
#11242=CARTESIAN_POINT ( 'NONE',  ( 46.50192534792603283, 74.36443251879779837, 10.00000000000000000 ) ) ;
#11245=LINE ( 'NONE', #35005, #35285 ) ;
#11250=DIRECTION ( 'NONE',  ( -0.9303772761487891785, -0.3666034970181814012, 0.000000000000000000 ) ) ;
#11264=DIRECTION ( 'NONE',  ( 0.000000000000000000, 0.000000000000000000, 1.000000000000000000 ) ) ;
#11268=VERTEX_POINT ( 'NONE', #75840 ) ;
#11273=EDGE_CURVE ( 'NONE', #35906, #13323, #84945, .T. ) ;
#11275=VECTOR ( 'NONE', #38525, 1000.000000000000114 ) ;
#11278=DIRECTION ( 'NONE',  ( 0.7492053821868994712, 0.6623377501714527993, 0.000000000000000000 ) ) ;
#11289=CIRCLE ( 'NONE', #82482, 0.1418229129680828593 ) ;
#11296=EDGE_CURVE ( 'NONE', #48810, #80286, #67213, .T. ) ;
#11303=FACE_OUTER_BOUND ( 'NONE', #13525, .T. ) ;
#11309=VECTOR ( 'NONE', #90063, 1000.000000000000114 ) ;
#11314=CARTESIAN_POINT ( 'NONE',  ( 48.05312180239142350, 111.8345470171556428, 10.00000000000000000 ) ) ;
#11316=DIRECTION ( 'NONE',  ( 0.000000000000000000, 0.000000000000000000, 1.000000000000000000 ) ) ;
#11320=ORIENTED_EDGE ( 'NONE', *, *, #66082, .T. ) ;
#11321=ORIENTED_EDGE ( 'NONE', *, *, #30086, .T. ) ;
#11323=DIRECTION ( 'NONE',  ( 1.000000000000000000, 0.000000000000000000, 0.000000000000000000 ) ) ;
#11327=DIRECTION ( 'NONE',  ( -1.000000000000000000, 0.000000000000000000, 0.000000000000000000 ) ) ;
#11333=ORIENTED_EDGE ( 'NONE', *, *, #66938, .T. ) ;
#11336=DIRECTION ( 'NONE',  ( -1.000000000000000000, -9.785293164091215354E-14, 0.000000000000000000 ) ) ;
#11339=EDGE_CURVE ( 'NONE', #98279, #100024, #98644, .T. ) ;
#11342=VERTEX_POINT ( 'NONE', #91060 ) ;
#11345=LINE ( 'NONE', #19448, #76745 ) ;
#11356=VERTEX_POINT ( 'NONE', #39773 ) ;
#11375=VERTEX_POINT ( 'NONE', #7922 ) ;
#11379=CARTESIAN_POINT ( 'NONE',  ( -8.406493707509316238, 25.24382671950691304, -10.00000000000000000 ) ) ;
#11386=CARTESIAN_POINT ( 'NONE',  ( -4.170157060006060235, 26.08383846222962887, 10.00000000000000000 ) ) ;
#11397=CARTESIAN_POINT ( 'NONE',  ( -16.14350997085658435, 56.98620320469874656, 0.000000000000000000 ) ) ;
#11405=EDGE_CURVE ( 'NONE', #2950, #29361, #55482, .T. ) ;
#11409=LINE ( 'NONE', #49879, #19166 ) ;
#11410=VERTEX_POINT ( 'NONE', #31682 ) ;
#11429=EDGE_LOOP ( 'NONE', ( #87997, #31954, #55015, #25919 ) ) ;
#11435=CARTESIAN_POINT ( 'NONE',  ( -9.055497838557604595, 23.87190447404379157, -10.00000000000000000 ) ) ;
#11438=VECTOR ( 'NONE', #71915, 1000.000000000000000 ) ;
#11455=EDGE_CURVE ( 'NONE', #63771, #11090, #35570, .T. ) ;
#11464=ORIENTED_EDGE ( 'NONE', *, *, #5199, .F. ) ;
#11465=EDGE_CURVE ( 'NONE', #76337, #82333, #67898, .T. ) ;
#11474=CARTESIAN_POINT ( 'NONE',  ( 3.854092266844447501, 28.45370138451379560, -10.00000000000000000 ) ) ;
#11480=EDGE_CURVE ( 'NONE', #46907, #88625, #17505, .T. ) ;
#11498=DIRECTION ( 'NONE',  ( -0.000000000000000000, 0.000000000000000000, 1.000000000000000000 ) ) ;
#11506=DIRECTION ( 'NONE',  ( 1.000000000000000000, 0.000000000000000000, 0.000000000000000000 ) ) ;
#11536=ORIENTED_EDGE ( 'NONE', *, *, #43100, .F. ) ;
#11542=EDGE_CURVE ( 'NONE', #82653, #2846, #66104, .T. ) ;
#11550=ORIENTED_EDGE ( 'NONE', *, *, #51791, .T. ) ;
#11555=DIRECTION ( 'NONE',  ( 1.000000000000000000, 0.000000000000000000, 0.000000000000000000 ) ) ;
#11556=ORIENTED_EDGE ( 'NONE', *, *, #10728, .T. ) ;
#11558=VERTEX_POINT ( 'NONE', #12419 ) ;
#11568=EDGE_LOOP ( 'NONE', ( #35486, #53010, #99322, #26926 ) ) ;
#11569=VECTOR ( 'NONE', #39557, 1000.000000000000000 ) ;
#11582=EDGE_CURVE ( 'NONE', #85223, #20973, #65107, .T. ) ;
#11585=CARTESIAN_POINT ( 'NONE',  ( 3.854092266844447501, 28.45370138451379560, -10.00000000000000000 ) ) ;
#11598=ORIENTED_EDGE ( 'NONE', *, *, #31216, .T. ) ;
#11599=DIRECTION ( 'NONE',  ( -0.8951289669282589401, 0.4458072818673421422, 0.000000000000000000 ) ) ;
#11600=CARTESIAN_POINT ( 'NONE',  ( 49.07419501245632176, 91.40403951869188859, -10.00000000000000000 ) ) ;
#11601=ORIENTED_EDGE ( 'NONE', *, *, #80048, .T. ) ;
#11608=CARTESIAN_POINT ( 'NONE',  ( -56.16025090550425602, 33.03454289568183100, -10.00000000000000000 ) ) ;
#11624=DIRECTION ( 'NONE',  ( 0.000000000000000000, 0.000000000000000000, 1.000000000000000000 ) ) ;
#11641=LINE ( 'NONE', #66322, #79153 ) ;
#11655=EDGE_CURVE ( 'NONE', #68082, #84967, #51906, .T. ) ;
#11664=DIRECTION ( 'NONE',  ( 0.000000000000000000, 0.000000000000000000, 1.000000000000000000 ) ) ;
#11678=CARTESIAN_POINT ( 'NONE',  ( -44.55566051625979895, 47.72160670319654230, 59.99999999999999289 ) ) ;
#11679=CYLINDRICAL_SURFACE ( 'NONE', #24591, 45.00000000000000000 ) ;
#11683=PLANE ( 'NONE',  #23754 ) ;
#11685=VERTEX_POINT ( 'NONE', #29111 ) ;
#11689=AXIS2_PLACEMENT_3D ( 'NONE', #82818, #75190, #5765 ) ;
#11701=ORIENTED_EDGE ( 'NONE', *, *, #7264, .F. ) ;
#11713=FACE_OUTER_BOUND ( 'NONE', #15165, .T. ) ;
#11727=ORIENTED_EDGE ( 'NONE', *, *, #98097, .T. ) ;
#11732=FACE_OUTER_BOUND ( 'NONE', #17928, .T. ) ;
#11739=LINE ( 'NONE', #42603, #67264 ) ;
#11743=AXIS2_PLACEMENT_3D ( 'NONE', #44527, #83085, #61230 ) ;
#11757=VECTOR ( 'NONE', #65529, 1000.000000000000000 ) ;
#11780=EDGE_CURVE ( 'NONE', #71872, #5333, #92243, .T. ) ;
#11809=ORIENTED_EDGE ( 'NONE', *, *, #45398, .T. ) ;
#11814=DIRECTION ( 'NONE',  ( -0.2473641778533917646, -0.9689225787001330970, 0.000000000000000000 ) ) ;
#11816=ORIENTED_EDGE ( 'NONE', *, *, #31520, .F. ) ;
#11819=CIRCLE ( 'NONE', #68405, 70.00000000000001421 ) ;
#11828=VECTOR ( 'NONE', #46656, 1000.000000000000000 ) ;
#11831=VERTEX_POINT ( 'NONE', #84707 ) ;
#11832=CARTESIAN_POINT ( 'NONE',  ( 32.07560492619583670, 120.7590592525220075, 59.99999999999999289 ) ) ;
#11837=CARTESIAN_POINT ( 'NONE',  ( -0.06004842451780637025, 38.53370552223154988, 59.99999999999999289 ) ) ;
#11840=AXIS2_PLACEMENT_3D ( 'NONE', #82972, #84465, #44910 ) ;
#11845=CARTESIAN_POINT ( 'NONE',  ( 22.66956910419568061, 38.88013629349136835, -10.00000000000000000 ) ) ;
#11850=LINE ( 'NONE', #73640, #99872 ) ;
#11861=EDGE_CURVE ( 'NONE', #1989, #34033, #86225, .T. ) ;
#11869=LINE ( 'NONE', #88928, #23628 ) ;
#11870=ORIENTED_EDGE ( 'NONE', *, *, #35158, .T. ) ;
#11875=DIRECTION ( 'NONE',  ( 0.1473778574936323582, 0.9890802632347824863, 0.000000000000000000 ) ) ;
#11886=AXIS2_PLACEMENT_3D ( 'NONE', #16496, #30708, #85451 ) ;
#11900=VECTOR ( 'NONE', #9654, 1000.000000000000227 ) ;
#11917=ORIENTED_EDGE ( 'NONE', *, *, #63440, .T. ) ;
#11925=VERTEX_POINT ( 'NONE', #64366 ) ;
#11929=VERTEX_POINT ( 'NONE', #18779 ) ;
#11935=FACE_OUTER_BOUND ( 'NONE', #53012, .T. ) ;
#11938=ORIENTED_EDGE ( 'NONE', *, *, #53502, .F. ) ;
#11942=ORIENTED_EDGE ( 'NONE', *, *, #235, .F. ) ;
#11943=VERTEX_POINT ( 'NONE', #94802 ) ;
#11961=AXIS2_PLACEMENT_3D ( 'NONE', #8154, #55226, #70446 ) ;
#11962=EDGE_CURVE ( 'NONE', #94878, #97533, #57750, .T. ) ;
#11963=DIRECTION ( 'NONE',  ( -0.000000000000000000, -0.000000000000000000, -1.000000000000000000 ) ) ;
#11964=ORIENTED_EDGE ( 'NONE', *, *, #75812, .F. ) ;
#11976=ORIENTED_EDGE ( 'NONE', *, *, #53472, .T. ) ;
#11978=DIRECTION ( 'NONE',  ( -0.000000000000000000, -0.000000000000000000, 1.000000000000000000 ) ) ;
#11979=EDGE_CURVE ( 'NONE', #75787, #50887, #3212, .T. ) ;
#11992=CARTESIAN_POINT ( 'NONE',  ( -67.91103796225580425, 44.10201266000169795, -10.00000000000000000 ) ) ;
#11993=EDGE_CURVE ( 'NONE', #84833, #79042, #48166, .T. ) ;
#11995=FACE_OUTER_BOUND ( 'NONE', #69506, .T. ) ;
#11997=DIRECTION ( 'NONE',  ( 1.000000000000000000, -1.153838929164001651E-13, 0.000000000000000000 ) ) ;
#12012=EDGE_CURVE ( 'NONE', #39035, #87819, #56760, .T. ) ;
#12015=CARTESIAN_POINT ( 'NONE',  ( -42.23460334637721303, 26.80738527414552408, 10.00000000000000000 ) ) ;
#12016=CARTESIAN_POINT ( 'NONE',  ( 45.34926676561319425, 66.39822172987334170, -10.00000000000000000 ) ) ;
#12017=ADVANCED_FACE ( 'NONE', ( #64876 ), #95822, .T. ) ;
#12028=DIRECTION ( 'NONE',  ( 1.000000000000000000, 7.275925893525578569E-14, 0.000000000000000000 ) ) ;
#12034=PLANE ( 'NONE',  #82596 ) ;
#12041=ORIENTED_EDGE ( 'NONE', *, *, #74967, .T. ) ;
#12048=VECTOR ( 'NONE', #13447, 1000.000000000000000 ) ;
#12049=ORIENTED_EDGE ( 'NONE', *, *, #37813, .T. ) ;
#12056=CARTESIAN_POINT ( 'NONE',  ( 19.39999966495784989, 36.48715600906564305, -10.00000000000000000 ) ) ;
#12058=LINE ( 'NONE', #87629, #65917 ) ;
#12059=ORIENTED_EDGE ( 'NONE', *, *, #5644, .T. ) ;
#12060=ORIENTED_EDGE ( 'NONE', *, *, #13474, .T. ) ;
#12066=DIRECTION ( 'NONE',  ( -0.7080737730998298840, 0.7061384650677022812, 0.000000000000000000 ) ) ;
#12075=ORIENTED_EDGE ( 'NONE', *, *, #5755, .F. ) ;
#12084=DIRECTION ( 'NONE',  ( -0.2575544297740022803, 0.9662637919863232838, 0.000000000000000000 ) ) ;
#12093=DIRECTION ( 'NONE',  ( 1.000000000000000000, 0.000000000000000000, 0.000000000000000000 ) ) ;
#12094=CARTESIAN_POINT ( 'NONE',  ( -42.47074677134370546, 28.21475011077167849, -10.00000000000000000 ) ) ;
#12095=EDGE_LOOP ( 'NONE', ( #90099, #61533, #6200, #90460 ) ) ;
#12101=EDGE_CURVE ( 'NONE', #59362, #55035, #94132, .T. ) ;
#12104=VECTOR ( 'NONE', #49702, 1000.000000000000114 ) ;
#12118=LINE ( 'NONE', #51091, #93521 ) ;
#12125=ORIENTED_EDGE ( 'NONE', *, *, #48465, .T. ) ;
#12132=CIRCLE ( 'NONE', #33171, 49.99999999999999289 ) ;
#12139=DIRECTION ( 'NONE',  ( -0.9909246428798921258, -0.1344185706417024839, 0.000000000000000000 ) ) ;
#12140=DIRECTION ( 'NONE',  ( 1.000000000000000000, 0.000000000000000000, 0.000000000000000000 ) ) ;
#12144=FACE_OUTER_BOUND ( 'NONE', #29588, .T. ) ;
#12148=LINE ( 'NONE', #57227, #88759 ) ;
#12149=ORIENTED_EDGE ( 'NONE', *, *, #11582, .T. ) ;
#12154=PLANE ( 'NONE',  #79043 ) ;
#12158=CARTESIAN_POINT ( 'NONE',  ( -19.65312891409030271, 93.06504152958497400, -10.00000000000000888 ) ) ;
#12163=ORIENTED_EDGE ( 'NONE', *, *, #43755, .T. ) ;
#12167=CARTESIAN_POINT ( 'NONE',  ( 47.49582885874516336, 78.29235751436857527, -10.00000000000000000 ) ) ;
#12176=CARTESIAN_POINT ( 'NONE',  ( 34.25126403021256749, 69.88882648778609052, 59.99999999999999289 ) ) ;
#12178=EDGE_LOOP ( 'NONE', ( #74111, #71506, #64228, #32976 ) ) ;
#12180=DIRECTION ( 'NONE',  ( -0.5102188382608503492, 0.8600446134263898257, 0.000000000000000000 ) ) ;
#12181=FACE_OUTER_BOUND ( 'NONE', #13887, .T. ) ;
#12185=AXIS2_PLACEMENT_3D ( 'NONE', #14005, #6411, #21611 ) ;
#12189=ORIENTED_EDGE ( 'NONE', *, *, #80428, .F. ) ;
#12192=ORIENTED_EDGE ( 'NONE', *, *, #30086, .F. ) ;
#12194=FACE_BOUND ( 'NONE', #20291, .T. ) ;
#12197=ORIENTED_EDGE ( 'NONE', *, *, #39476, .T. ) ;
#12209=DIRECTION ( 'NONE',  ( 0.000000000000000000, -0.000000000000000000, 1.000000000000000000 ) ) ;
#12210=DIRECTION ( 'NONE',  ( 1.000000000000000000, 0.000000000000000000, 0.000000000000000000 ) ) ;
#12212=DIRECTION ( 'NONE',  ( -0.000000000000000000, 0.000000000000000000, -1.000000000000000000 ) ) ;
#12223=CARTESIAN_POINT ( 'NONE',  ( 49.07456115661582174, 91.13648234292965356, 10.00000000000000000 ) ) ;
#12229=DIRECTION ( 'NONE',  ( -0.000000000000000000, 0.000000000000000000, 1.000000000000000000 ) ) ;
#12231=CARTESIAN_POINT ( 'NONE',  ( -47.59865527897274973, 48.00312894580780210, 59.99999999999999289 ) ) ;
#12233=CARTESIAN_POINT ( 'NONE',  ( -66.55019942848203129, 42.78701949053055387, -10.00000000000000000 ) ) ;
#12239=VECTOR ( 'NONE', #57268, 1000.000000000000114 ) ;
#12246=VECTOR ( 'NONE', #25241, 1000.000000000000227 ) ;
#12247=DIRECTION ( 'NONE',  ( -1.000000000000000000, 0.000000000000000000, 0.000000000000000000 ) ) ;
#12249=EDGE_CURVE ( 'NONE', #78709, #62627, #21069, .T. ) ;
#12252=ORIENTED_EDGE ( 'NONE', *, *, #34281, .F. ) ;
#12268=CARTESIAN_POINT ( 'NONE',  ( 32.30839531297598910, 123.0650415295850593, -10.00000000000000888 ) ) ;
#12272=LINE ( 'NONE', #74074, #38489 ) ;
#12280=CARTESIAN_POINT ( 'NONE',  ( -19.65312891409030271, 93.06504152958497400, 10.00000000000000888 ) ) ;
#12287=FACE_OUTER_BOUND ( 'NONE', #61546, .T. ) ;
#12288=VECTOR ( 'NONE', #21447, 1000.000000000000000 ) ;
#12289=DIRECTION ( 'NONE',  ( 0.9819794923402651587, -0.1889875038809575580, 0.000000000000000000 ) ) ;
#12293=DIRECTION ( 'NONE',  ( 1.000000000000000000, 0.000000000000000000, 0.000000000000000000 ) ) ;
#12295=ORIENTED_EDGE ( 'NONE', *, *, #49742, .T. ) ;
#12298=CIRCLE ( 'NONE', #13948, 70.00000000000001421 ) ;
#12302=ORIENTED_EDGE ( 'NONE', *, *, #74187, .F. ) ;
#12304=DIRECTION ( 'NONE',  ( -0.7135562106085678868, 0.7005979833698787740, 0.000000000000000000 ) ) ;
#12312=VERTEX_POINT ( 'NONE', #82450 ) ;
#12316=ORIENTED_EDGE ( 'NONE', *, *, #97480, .T. ) ;
#12319=ORIENTED_EDGE ( 'NONE', *, *, #67961, .F. ) ;
#12323=DIRECTION ( 'NONE',  ( -0.000000000000000000, -0.000000000000000000, -1.000000000000000000 ) ) ;
#12327=CARTESIAN_POINT ( 'NONE',  ( -71.45866285464214229, 45.60329508610311677, -10.00000000000000000 ) ) ;
#12328=DIRECTION ( 'NONE',  ( 0.000000000000000000, -0.000000000000000000, -1.000000000000000000 ) ) ;
#12329=DIRECTION ( 'NONE',  ( -0.9172102815912979157, -0.3984034379159046013, 0.000000000000000000 ) ) ;
#12340=ORIENTED_EDGE ( 'NONE', *, *, #35836, .F. ) ;
#12342=DIRECTION ( 'NONE',  ( -0.000000000000000000, -0.000000000000000000, -1.000000000000000000 ) ) ;
#12343=DIRECTION ( 'NONE',  ( 0.8660254037844390407, 0.4999999999999992228, -0.000000000000000000 ) ) ;
#12345=EDGE_CURVE ( 'NONE', #47438, #82969, #95518, .T. ) ;
#12351=FACE_OUTER_BOUND ( 'NONE', #5807, .T. ) ;
#12355=EDGE_CURVE ( 'NONE', #71997, #32616, #8099, .T. ) ;
#12363=VECTOR ( 'NONE', #69757, 1000.000000000000000 ) ;
#12365=ORIENTED_EDGE ( 'NONE', *, *, #30617, .T. ) ;
#12366=AXIS2_PLACEMENT_3D ( 'NONE', #3495, #66762, #58648 ) ;
#12372=CARTESIAN_POINT ( 'NONE',  ( -19.65312891409030271, 93.06504152958497400, 10.00000000000000888 ) ) ;
#12382=VECTOR ( 'NONE', #27918, 1000.000000000000114 ) ;
#12393=CARTESIAN_POINT ( 'NONE',  ( -19.65312891409030271, 93.06504152958497400, -10.00000000000000888 ) ) ;
#12394=ORIENTED_EDGE ( 'NONE', *, *, #61621, .T. ) ;
#12405=EDGE_LOOP ( 'NONE', ( #95406, #7945, #89412, #68964 ) ) ;
#12411=CARTESIAN_POINT ( 'NONE',  ( 47.32807415326522715, 108.5480133836684900, -10.00000000000000000 ) ) ;
#12419=CARTESIAN_POINT ( 'NONE',  ( -74.22192597045216189, 49.22161114575668250, -10.00000000000000000 ) ) ;
#12424=DIRECTION ( 'NONE',  ( 0.000000000000000000, 0.000000000000000000, 1.000000000000000000 ) ) ;
#12428=VERTEX_POINT ( 'NONE', #38761 ) ;
#12434=CARTESIAN_POINT ( 'NONE',  ( -55.59287931351117606, 32.99562883703961091, 10.00000000000000000 ) ) ;
#12438=DIRECTION ( 'NONE',  ( -0.9778746070300391446, 0.2091919045418505763, 0.000000000000000000 ) ) ;
#12443=CIRCLE ( 'NONE', #65781, 0.1418229129680854683 ) ;
#12444=ORIENTED_EDGE ( 'NONE', *, *, #30036, .F. ) ;
#12446=ORIENTED_EDGE ( 'NONE', *, *, #12012, .F. ) ;
#12449=VERTEX_POINT ( 'NONE', #63568 ) ;
#12461=ORIENTED_EDGE ( 'NONE', *, *, #98481, .F. ) ;
#12464=ORIENTED_EDGE ( 'NONE', *, *, #55315, .T. ) ;
#12465=AXIS2_PLACEMENT_3D ( 'NONE', #81145, #48194, #9723 ) ;
#12467=CARTESIAN_POINT ( 'NONE',  ( -19.65312891409030271, 93.06504152958497400, 10.00000000000000888 ) ) ;
#12470=DIRECTION ( 'NONE',  ( 0.000000000000000000, 0.000000000000000000, 1.000000000000000000 ) ) ;
#12471=AXIS2_PLACEMENT_3D ( 'NONE', #73848, #58618, #28739 ) ;
#12472=B_SPLINE_CURVE_WITH_KNOTS ( 'NONE', 3,
 ( #84240, #69976, #14299, #99905, #29495, #68981, #54779, #21890, #29988, #38580, #91830, #6697, #77085, #92821, #91329, #78102, #45185, #22392, #46164, #37090, #30490, #22882, #54262, #37575, #100, #14789, #68483, #53768, #53288, #30984, #590, #67994, #60372, #52776, #7689, #76596, #84730, #38067, #15270, #61870, #85232, #15778, #46684 ),
 .UNSPECIFIED., .F., .F.,
 ( 4, 2, 2, 2, 2, 1, 2, 2, 2, 2, 2, 2, 2, 2, 2, 2, 2, 2, 2, 2, 2, 4 ),
 ( 0.02141244383927110029, 0.02208092004936386410, 0.02274939625945662791, 0.02408634867964215207, 0.02475482488973493669, 0.02542330109982772132, 0.02609177730992050595, 0.02676025352001328711, 0.02809720594019887718, 0.02876568215029168263, 0.02943415836038448807, 0.03077111078057008509, 0.03210806320075568210, 0.03277653941084848060, 0.03344501562094127911, 0.03478196804112686225, 0.03611892046131245232, 0.03745587288149804239, 0.03879282530168363247, 0.04012977772186922254, 0.04146673014205480567, 0.04280368256224039575 ),
 .UNSPECIFIED. ) ;
#12481=EDGE_CURVE ( 'NONE', #33383, #58141, #77793, .T. ) ;
#12486=DIRECTION ( 'NONE',  ( -0.000000000000000000, -0.000000000000000000, -1.000000000000000000 ) ) ;
#12492=DIRECTION ( 'NONE',  ( -0.9979398670145497308, -0.06415622980648832963, 0.000000000000000000 ) ) ;
#12498=DIRECTION ( 'NONE',  ( -0.9086904199442051855, 0.4174706225611858335, 0.000000000000000000 ) ) ;
#12505=VECTOR ( 'NONE', #57517, 1000.000000000000000 ) ;
#12510=PLANE ( 'NONE',  #52920 ) ;
#12522=LINE ( 'NONE', #36296, #96382 ) ;
#12523=EDGE_CURVE ( 'NONE', #55246, #25048, #764, .T. ) ;
#12526=EDGE_LOOP ( 'NONE', ( #95712, #7454, #98687, #6585 ) ) ;
#12528=AXIS2_PLACEMENT_3D ( 'NONE', #726, #78749, #31612 ) ;
#12533=DIRECTION ( 'NONE',  ( 0.5011331959107180323, 0.8653701635463924013, 0.000000000000000000 ) ) ;
#12535=CARTESIAN_POINT ( 'NONE',  ( -19.65312891409030271, 93.06504152958497400, 59.99999999999999289 ) ) ;
#12539=VECTOR ( 'NONE', #1673, 1000.000000000000114 ) ;
#12548=DIRECTION ( 'NONE',  ( -0.6141984594095433181, -0.7891516029629183082, 0.000000000000000000 ) ) ;
#12555=FACE_OUTER_BOUND ( 'NONE', #50155, .T. ) ;
#12559=ADVANCED_FACE ( 'NONE', ( #40751 ), #56957, .T. ) ;
#12562=ORIENTED_EDGE ( 'NONE', *, *, #15192, .T. ) ;
#12571=CARTESIAN_POINT ( 'NONE',  ( 48.95103868752454446, 97.61288834769685252, -10.00000000000000000 ) ) ;
#12572=CARTESIAN_POINT ( 'NONE',  ( 7.864685750751951865, 30.05722773587472929, -10.00000000000000000 ) ) ;
#12575=CARTESIAN_POINT ( 'NONE',  ( -19.65312891409030271, 93.06504152958497400, -40.00000000000000000 ) ) ;
#12580=VECTOR ( 'NONE', #48661, 999.9999999999998863 ) ;
#12581=ORIENTED_EDGE ( 'NONE', *, *, #89508, .T. ) ;
#12588=LINE ( 'NONE', #34374, #85662 ) ;
#12592=ADVANCED_FACE ( 'NONE', ( #77018 ), #44609, .F. ) ;
#12594=ORIENTED_EDGE ( 'NONE', *, *, #64591, .F. ) ;
#12596=ORIENTED_EDGE ( 'NONE', *, *, #66008, .F. ) ;
#12597=ADVANCED_FACE ( 'NONE', ( #21829 ), #75544, .F. ) ;
#12599=DIRECTION ( 'NONE',  ( -0.7911563084720502070, -0.6116140086401538056, 0.000000000000000000 ) ) ;
#12607=EDGE_CURVE ( 'NONE', #9589, #45905, #84006, .T. ) ;
#12617=VECTOR ( 'NONE', #49605, 1000.000000000000114 ) ;
#12620=CARTESIAN_POINT ( 'NONE',  ( 27.58098951138966726, 43.10352854649765675, -10.00000000000000000 ) ) ;
#12621=CARTESIAN_POINT ( 'NONE',  ( -54.25007008209492909, 32.21233689110872689, 177.5919119679930134 ) ) ;
#12624=CARTESIAN_POINT ( 'NONE',  ( -19.65312891409030271, 93.06504152958497400, 59.99999999999999289 ) ) ;
#12634=EDGE_LOOP ( 'NONE', ( #28333, #68118, #25117, #69331 ) ) ;
#12637=LINE ( 'NONE', #66809, #90446 ) ;
#12640=VECTOR ( 'NONE', #97804, 1000.000000000000000 ) ;
#12646=LINE ( 'NONE', #35917, #72396 ) ;
#12648=AXIS2_PLACEMENT_3D ( 'NONE', #8051, #942, #9038 ) ;
#12664=EDGE_CURVE ( 'NONE', #95472, #64892, #1545, .T. ) ;
#12678=FACE_OUTER_BOUND ( 'NONE', #48082, .T. ) ;
#12685=ORIENTED_EDGE ( 'NONE', *, *, #68758, .T. ) ;
#12704=FACE_BOUND ( 'NONE', #65637, .T. ) ;
#12705=DIRECTION ( 'NONE',  ( -0.9879014915521923124, 0.1550826972584425645, 0.000000000000000000 ) ) ;
#12713=EDGE_CURVE ( 'NONE', #34033, #69834, #32919, .T. ) ;
#12716=VECTOR ( 'NONE', #30004, 1000.000000000000114 ) ;
#12718=CARTESIAN_POINT ( 'NONE',  ( -77.58047734835669473, 56.02942318228900120, -10.00000000000000000 ) ) ;
#12720=CARTESIAN_POINT ( 'NONE',  ( -23.73952538801239598, 24.43184193311134678, 10.00000000000000000 ) ) ;
#12721=VECTOR ( 'NONE', #70966, 1000.000000000000227 ) ;
#12722=EDGE_CURVE ( 'NONE', #65850, #68464, #10638, .T. ) ;
#12723=DIRECTION ( 'NONE',  ( -1.000000000000000000, 0.000000000000000000, 0.000000000000000000 ) ) ;
#12727=ORIENTED_EDGE ( 'NONE', *, *, #90949, .T. ) ;
#12732=ORIENTED_EDGE ( 'NONE', *, *, #24408, .T. ) ;
#12735=CARTESIAN_POINT ( 'NONE',  ( -19.65312891409030271, 93.06504152958497400, 177.5919119679930134 ) ) ;
#12736=CARTESIAN_POINT ( 'NONE',  ( 43.63646518856938172, 66.22046553916848666, 10.00000000000000000 ) ) ;
#12739=ORIENTED_EDGE ( 'NONE', *, *, #56431, .T. ) ;
#12741=VECTOR ( 'NONE', #11218, 1000.000000000000000 ) ;
#12748=CARTESIAN_POINT ( 'NONE',  ( 48.73804053012794668, 107.9864336245683631, 10.00000000000000000 ) ) ;
#12785=ADVANCED_FACE ( 'NONE', ( #87205 ), #17738, .F. ) ;
#12807=EDGE_CURVE ( 'NONE', #28368, #70394, #11641, .T. ) ;
#12830=ORIENTED_EDGE ( 'NONE', *, *, #26890, .F. ) ;
#12831=PLANE ( 'NONE',  #83906 ) ;
#12834=ORIENTED_EDGE ( 'NONE', *, *, #70805, .T. ) ;
#12835=ADVANCED_FACE ( 'NONE', ( #42500 ), #89671, .F. ) ;
#12851=CARTESIAN_POINT ( 'NONE',  ( 48.81784752633561908, 86.82484054835779830, -10.00000000000000000 ) ) ;
#12852=ORIENTED_EDGE ( 'NONE', *, *, #83952, .F. ) ;
#12859=ORIENTED_EDGE ( 'NONE', *, *, #21601, .T. ) ;
#12873=ORIENTED_EDGE ( 'NONE', *, *, #36819, .F. ) ;
#12874=VECTOR ( 'NONE', #84175, 1000.000000000000114 ) ;
#12886=VERTEX_POINT ( 'NONE', #5028 ) ;
#12898=FACE_OUTER_BOUND ( 'NONE', #32146, .T. ) ;
#12904=CARTESIAN_POINT ( 'NONE',  ( -19.65312891409030271, 93.06504152958497400, -10.00000000000000888 ) ) ;
#12909=DIRECTION ( 'NONE',  ( 0.2194785493951409983, -0.9756173257765591300, 0.000000000000000000 ) ) ;
#12910=DIRECTION ( 'NONE',  ( -0.04056776950002415755, 0.9991767892008865948, 0.000000000000000000 ) ) ;
#12924=CARTESIAN_POINT ( 'NONE',  ( 40.34888600819125060, 126.6204015641749834, 10.00000000000000000 ) ) ;
#12930=EDGE_CURVE ( 'NONE', #4371, #8415, #58696, .T. ) ;
#12935=EDGE_CURVE ( 'NONE', #69469, #65627, #12637, .T. ) ;
#12939=AXIS2_PLACEMENT_3D ( 'NONE', #33763, #87526, #95092 ) ;
#12943=CARTESIAN_POINT ( 'NONE',  ( 7.864685750751951865, 30.05722773587472929, 10.00000000000000000 ) ) ;
#12944=VERTEX_POINT ( 'NONE', #90161 ) ;
#12952=VERTEX_POINT ( 'NONE', #20733 ) ;
#12954=EDGE_LOOP ( 'NONE', ( #76120, #6071, #12197, #27432 ) ) ;
#12955=CARTESIAN_POINT ( 'NONE',  ( 45.66470909604093720, 114.5311720768849995, -10.00000000000000000 ) ) ;
#12956=AXIS2_PLACEMENT_3D ( 'NONE', #25062, #77269, #40749 ) ;
#12969=ORIENTED_EDGE ( 'NONE', *, *, #93756, .F. ) ;
#12970=VECTOR ( 'NONE', #49657, 1000.000000000000227 ) ;
#12971=DIRECTION ( 'NONE',  ( 0.1860369090530955005, 0.9825427565607363078, 0.000000000000000000 ) ) ;
#12982=DIRECTION ( 'NONE',  ( 0.000000000000000000, 0.000000000000000000, 1.000000000000000000 ) ) ;
#12988=CARTESIAN_POINT ( 'NONE',  ( -8.378993335088974703, 41.25363085138964436, 59.99999999999999289 ) ) ;
#12990=CARTESIAN_POINT ( 'NONE',  ( -56.29836151245349640, 34.88994676555962826, -10.00000000000000000 ) ) ;
#12996=EDGE_LOOP ( 'NONE', ( #38849, #10868, #97075, #17240 ) ) ;
#13020=CARTESIAN_POINT ( 'NONE',  ( 47.32807415326522715, 108.5480133836684900, 10.00000000000000000 ) ) ;
#13021=VECTOR ( 'NONE', #2776, 1000.000000000000000 ) ;
#13031=PLANE ( 'NONE',  #55814 ) ;
#13039=LINE ( 'NONE', #65706, #34790 ) ;
#13041=EDGE_CURVE ( 'NONE', #69843, #68477, #75082, .T. ) ;
#13044=CARTESIAN_POINT ( 'NONE',  ( -25.04755574468711643, 23.27320705613571761, -10.00000000000000000 ) ) ;
#13046=DIRECTION ( 'NONE',  ( 0.000000000000000000, -0.000000000000000000, -1.000000000000000000 ) ) ;
#13051=ORIENTED_EDGE ( 'NONE', *, *, #47220, .T. ) ;
#13068=ORIENTED_EDGE ( 'NONE', *, *, #74460, .T. ) ;
#13073=CARTESIAN_POINT ( 'NONE',  ( 46.99867368304095550, 76.19044720721625197, -10.00000000000000000 ) ) ;
#13081=LINE ( 'NONE', #82996, #2679 ) ;
#13085=EDGE_LOOP ( 'NONE', ( #88154, #16129, #23924, #66897 ) ) ;
#13087=CARTESIAN_POINT ( 'NONE',  ( -29.34079512516344934, 35.93620001148155296, 59.99999999999999289 ) ) ;
#13100=CARTESIAN_POINT ( 'NONE',  ( 48.98007068238331385, 88.97864505566217019, 10.00000000000000000 ) ) ;
#13121=CARTESIAN_POINT ( 'NONE',  ( 19.39689925177878749, 34.96947112835012916, -10.00000000000000000 ) ) ;
#13124=PLANE ( 'NONE',  #33409 ) ;
#13126=DIRECTION ( 'NONE',  ( 0.000000000000000000, 0.000000000000000000, 1.000000000000000000 ) ) ;
#13150=VECTOR ( 'NONE', #32611, 999.9999999999998863 ) ;
#13156=ORIENTED_EDGE ( 'NONE', *, *, #12807, .T. ) ;
#13161=CARTESIAN_POINT ( 'NONE',  ( -19.65312891409030271, 93.06504152958497400, -10.00000000000000888 ) ) ;
#13162=DIRECTION ( 'NONE',  ( 0.000000000000000000, 0.000000000000000000, 1.000000000000000000 ) ) ;
#13163=EDGE_CURVE ( 'NONE', #51434, #24006, #2280, .T. ) ;
#13164=EDGE_LOOP ( 'NONE', ( #58063, #86998, #92589, #84661 ) ) ;
#13165=CARTESIAN_POINT ( 'NONE',  ( -71.61465314115659453, 63.06504152958490295, -45.00000000000001421 ) ) ;
#13181=ORIENTED_EDGE ( 'NONE', *, *, #82689, .F. ) ;
#13184=DIRECTION ( 'NONE',  ( 0.000000000000000000, 0.000000000000000000, 1.000000000000000000 ) ) ;
#13198=VERTEX_POINT ( 'NONE', #86420 ) ;
#13199=FACE_BOUND ( 'NONE', #1885, .T. ) ;
#13203=CARTESIAN_POINT ( 'NONE',  ( -19.65312891409030271, 93.06504152958497400, 59.99999999999999289 ) ) ;
#13221=ORIENTED_EDGE ( 'NONE', *, *, #3285, .F. ) ;
#13232=AXIS2_PLACEMENT_3D ( 'NONE', #22354, #77042, #37540 ) ;
#13235=CARTESIAN_POINT ( 'NONE',  ( 49.66226845319756222, 83.29899382260624918, 177.5919119679930134 ) ) ;
#13247=EDGE_CURVE ( 'NONE', #20907, #75140, #35653, .T. ) ;
#13263=PLANE ( 'NONE',  #54913 ) ;
#13269=EDGE_CURVE ( 'NONE', #93745, #709, #30037, .T. ) ;
#13272=DIRECTION ( 'NONE',  ( -1.000000000000000000, 0.000000000000000000, 0.000000000000000000 ) ) ;
#13278=DIRECTION ( 'NONE',  ( -0.000000000000000000, -0.000000000000000000, -1.000000000000000000 ) ) ;
#13289=ADVANCED_FACE ( 'NONE', ( #85283 ), #52835, .F. ) ;
#13294=EDGE_CURVE ( 'NONE', #70849, #57017, #83785, .T. ) ;
#13296=ADVANCED_FACE ( 'NONE', ( #77135 ), #18350, .T. ) ;
#13305=CYLINDRICAL_SURFACE ( 'NONE', #56734, 70.00000000000002842 ) ;
#13308=ORIENTED_EDGE ( 'NONE', *, *, #43064, .T. ) ;
#13314=ORIENTED_EDGE ( 'NONE', *, *, #16607, .F. ) ;
#13317=ORIENTED_EDGE ( 'NONE', *, *, #11861, .T. ) ;
#13321=DIRECTION ( 'NONE',  ( -0.4897629171537489778, 0.8718556560469457040, 0.000000000000000000 ) ) ;
#13323=VERTEX_POINT ( 'NONE', #39113 ) ;
#13324=ORIENTED_EDGE ( 'NONE', *, *, #73317, .F. ) ;
#13332=ORIENTED_EDGE ( 'NONE', *, *, #12930, .F. ) ;
#13335=AXIS2_PLACEMENT_3D ( 'NONE', #20269, #51143, #73473 ) ;
#13336=CARTESIAN_POINT ( 'NONE',  ( 9.561825351099750847, 42.17961057553871029, 59.99999999999999289 ) ) ;
#13364=ADVANCED_FACE ( 'NONE', ( #24441 ), #16832, .F. ) ;
#13369=FACE_OUTER_BOUND ( 'NONE', #58363, .T. ) ;
#13371=CARTESIAN_POINT ( 'NONE',  ( -73.83803415018344651, 50.74234351129840093, -10.00000000000000000 ) ) ;
#13373=ORIENTED_EDGE ( 'NONE', *, *, #55327, .T. ) ;
#13387=ORIENTED_EDGE ( 'NONE', *, *, #88072, .F. ) ;
#13397=DIRECTION ( 'NONE',  ( -0.000000000000000000, -0.000000000000000000, 1.000000000000000000 ) ) ;
#13400=EDGE_CURVE ( 'NONE', #24879, #34490, #5620, .T. ) ;
#13401=FACE_OUTER_BOUND ( 'NONE', #35716, .T. ) ;
#13411=CARTESIAN_POINT ( 'NONE',  ( -69.61464189717713680, 45.83092310410447112, 10.00000000000000000 ) ) ;
#13412=EDGE_CURVE ( 'NONE', #79361, #42173, #44599, .T. ) ;
#13428=ORIENTED_EDGE ( 'NONE', *, *, #87455, .F. ) ;
#13435=EDGE_LOOP ( 'NONE', ( #10822, #45067, #32364, #36708 ) ) ;
#13442=ORIENTED_EDGE ( 'NONE', *, *, #24101, .T. ) ;
#13445=LINE ( 'NONE', #83358, #48212 ) ;
#13447=DIRECTION ( 'NONE',  ( 0.000000000000000000, 0.000000000000000000, 1.000000000000000000 ) ) ;
#13448=DIRECTION ( 'NONE',  ( 1.000000000000000000, 0.000000000000000000, 0.000000000000000000 ) ) ;
#13459=VERTEX_POINT ( 'NONE', #45114 ) ;
#13460=LINE ( 'NONE', #5840, #5768 ) ;
#13466=CARTESIAN_POINT ( 'NONE',  ( -12.34951437337453228, 41.85136669140065635, 59.99999999999999289 ) ) ;
#13472=EDGE_LOOP ( 'NONE', ( #31596, #41401, #1945, #40723 ) ) ;
#13474=EDGE_CURVE ( 'NONE', #18285, #94538, #77008, .T. ) ;
#13482=ORIENTED_EDGE ( 'NONE', *, *, #65196, .F. ) ;
#13485=CARTESIAN_POINT ( 'NONE',  ( -61.58631828649576079, 53.07550491216805710, 59.99999999999999289 ) ) ;
#13486=AXIS2_PLACEMENT_3D ( 'NONE', #59322, #5647, #13272 ) ;
#13487=EDGE_CURVE ( 'NONE', #861, #17015, #53214, .T. ) ;
#13491=EDGE_CURVE ( 'NONE', #11268, #60486, #53219, .T. ) ;
#13495=VECTOR ( 'NONE', #36911, 1000.000000000000114 ) ;
#13497=DIRECTION ( 'NONE',  ( -0.000000000000000000, -0.000000000000000000, -1.000000000000000000 ) ) ;
#13498=DIRECTION ( 'NONE',  ( -0.8756465943326132706, -0.4829524219151362097, 0.000000000000000000 ) ) ;
#13510=CARTESIAN_POINT ( 'NONE',  ( -25.89332989531674301, 24.59406508915897760, 10.00000000000000000 ) ) ;
#13513=CARTESIAN_POINT ( 'NONE',  ( -61.60412911085354182, 37.02832515102500111, 177.5919119679930134 ) ) ;
#13521=CARTESIAN_POINT ( 'NONE',  ( -80.08603253397792798, 57.73992072201551906, 10.00000000000000000 ) ) ;
#13525=EDGE_LOOP ( 'NONE', ( #61489, #59531, #55894, #17653 ) ) ;
#13535=CARTESIAN_POINT ( 'NONE',  ( 1.023347710557721113, 26.18841396516314646, 10.00000000000000000 ) ) ;
#13540=ORIENTED_EDGE ( 'NONE', *, *, #93450, .F. ) ;
#13551=EDGE_CURVE ( 'NONE', #23610, #26627, #7111, .T. ) ;
#13555=CARTESIAN_POINT ( 'NONE',  ( -19.65312891409030271, 93.06504152958497400, 177.5919119679930134 ) ) ;
#13565=VECTOR ( 'NONE', #37179, 1000.000000000000000 ) ;
#13573=DIRECTION ( 'NONE',  ( 0.000000000000000000, 0.000000000000000000, 1.000000000000000000 ) ) ;
#13582=VERTEX_POINT ( 'NONE', #60790 ) ;
#13597=ADVANCED_FACE ( 'NONE', ( #37505 ), #98514, .F. ) ;
#13598=CARTESIAN_POINT ( 'NONE',  ( 49.93482446054089507, 85.48106202472366988, -10.00000000000000000 ) ) ;
#13599=CYLINDRICAL_SURFACE ( 'NONE', #3267, 70.00000000000002842 ) ;
#13602=CARTESIAN_POINT ( 'NONE',  ( -44.43135095815892299, 47.65333612089700921, 59.99999999999999289 ) ) ;
#13604=EDGE_CURVE ( 'NONE', #63278, #8092, #49977, .T. ) ;
#13607=DIRECTION ( 'NONE',  ( -0.000000000000000000, -0.000000000000000000, -1.000000000000000000 ) ) ;
#13612=CARTESIAN_POINT ( 'NONE',  ( 18.86034532297697908, 34.61239144260639478, 10.00000000000000000 ) ) ;
#13617=CARTESIAN_POINT ( 'NONE',  ( -66.52313368742112232, 58.99514187658198949, 59.99999999999999289 ) ) ;
#13620=AXIS2_PLACEMENT_3D ( 'NONE', #12016, #49017, #11027 ) ;
#13622=DIRECTION ( 'NONE',  ( -0.000000000000000000, 0.000000000000000000, 1.000000000000000000 ) ) ;
#13630=CARTESIAN_POINT ( 'NONE',  ( 46.80869107419874098, 110.6443039040113092, 10.00000000000000000 ) ) ;
#13636=CARTESIAN_POINT ( 'NONE',  ( -42.72532191160158987, 28.29708160126036987, -10.00000000000000000 ) ) ;
#13639=CARTESIAN_POINT ( 'NONE',  ( 36.73352089011212485, 76.83585917327397397, 59.99999999999999289 ) ) ;
#13643=ORIENTED_EDGE ( 'NONE', *, *, #66124, .T. ) ;
#13646=LINE ( 'NONE', #99748, #38390 ) ;
#13648=DIRECTION ( 'NONE',  ( -0.000000000000000000, -0.000000000000000000, 1.000000000000000000 ) ) ;
#13653=CARTESIAN_POINT ( 'NONE',  ( -11.40312891409031693, 78.77562236714182120, 59.99999999999999289 ) ) ;
#13655=DIRECTION ( 'NONE',  ( -0.1580495287025880657, -0.9874311856918890351, 0.000000000000000000 ) ) ;
#13663=ORIENTED_EDGE ( 'NONE', *, *, #61017, .F. ) ;
#13668=FACE_OUTER_BOUND ( 'NONE', #60144, .T. ) ;
#13673=CARTESIAN_POINT ( 'NONE',  ( 10.06845959268932411, 31.07446838803123157, 10.00000000000000000 ) ) ;
#13674=EDGE_CURVE ( 'NONE', #89979, #97433, #72632, .T. ) ;
#13679=LINE ( 'NONE', #36964, #54466 ) ;
#13685=LINE ( 'NONE', #82641, #38569 ) ;
#13688=DIRECTION ( 'NONE',  ( 1.000000000000000000, 0.000000000000000000, 0.000000000000000000 ) ) ;
#13692=ORIENTED_EDGE ( 'NONE', *, *, #12249, .T. ) ;
#13694=LINE ( 'NONE', #64791, #64158 ) ;
#13696=DIRECTION ( 'NONE',  ( 0.9778746070300412541, -0.2091919045418403900, 0.000000000000000000 ) ) ;
#13703=CARTESIAN_POINT ( 'NONE',  ( -19.65312891409030271, 93.06504152958497400, 177.5919119679930134 ) ) ;
#13710=FACE_OUTER_BOUND ( 'NONE', #10090, .T. ) ;
#13719=CYLINDRICAL_SURFACE ( 'NONE', #54618, 70.00000000000002842 ) ;
#13723=DIRECTION ( 'NONE',  ( 0.000000000000000000, 0.000000000000000000, 1.000000000000000000 ) ) ;
#13724=LINE ( 'NONE', #36515, #96883 ) ;
#13730=ORIENTED_EDGE ( 'NONE', *, *, #94145, .F. ) ;
#13738=DIRECTION ( 'NONE',  ( -0.3766285016932175989, 0.9263643838751153270, 0.000000000000000000 ) ) ;
#13739=PLANE ( 'NONE',  #15324 ) ;
#13743=AXIS2_PLACEMENT_3D ( 'NONE', #76487, #46046, #59761 ) ;
#13749=CARTESIAN_POINT ( 'NONE',  ( -62.38288563085208693, 61.66892052422337400, 59.99999999999999289 ) ) ;
#13752=VECTOR ( 'NONE', #66510, 1000.000000000000000 ) ;
#13762=EDGE_CURVE ( 'NONE', #63494, #36466, #771, .T. ) ;
#13764=ORIENTED_EDGE ( 'NONE', *, *, #77078, .F. ) ;
#13769=ORIENTED_EDGE ( 'NONE', *, *, #84524, .T. ) ;
#13772=LINE ( 'NONE', #23351, #44501 ) ;
#13783=CARTESIAN_POINT ( 'NONE',  ( -19.65312891409030271, 93.06504152958497400, 10.00000000000000888 ) ) ;
#13785=EDGE_CURVE ( 'NONE', #34934, #41570, #85426, .T. ) ;
#13786=CARTESIAN_POINT ( 'NONE',  ( -16.99542894172669349, 24.36904009834038476, 10.00000000000000000 ) ) ;
#13788=ORIENTED_EDGE ( 'NONE', *, *, #65951, .F. ) ;
#13791=ORIENTED_EDGE ( 'NONE', *, *, #83109, .F. ) ;
#13799=CARTESIAN_POINT ( 'NONE',  ( 47.84007798744509898, 106.1754093786579318, 10.00000000000000000 ) ) ;
#13805=DIRECTION ( 'NONE',  ( 1.000000000000000000, 0.000000000000000000, 0.000000000000000000 ) ) ;
#13812=CARTESIAN_POINT ( 'NONE',  ( -76.38857681351474582, 54.22815603855766398, -10.00000000000000000 ) ) ;
#13814=DIRECTION ( 'NONE',  ( -0.9762143704923794685, 0.2168075248790210796, 0.000000000000000000 ) ) ;
#13816=ORIENTED_EDGE ( 'NONE', *, *, #1880, .T. ) ;
#13823=AXIS2_PLACEMENT_3D ( 'NONE', #79538, #80534, #12093 ) ;
#13824=CARTESIAN_POINT ( 'NONE',  ( 31.52185460810256856, 85.49507869652470049, 59.99999999999999289 ) ) ;
#13826=ORIENTED_EDGE ( 'NONE', *, *, #8795, .T. ) ;
#13829=DIRECTION ( 'NONE',  ( -0.000000000000000000, -0.000000000000000000, 1.000000000000000000 ) ) ;
#13834=CARTESIAN_POINT ( 'NONE',  ( -19.65312891409030271, 93.06504152958497400, 177.5919119679930134 ) ) ;
#13840=DIRECTION ( 'NONE',  ( 0.6116140086401538056, -0.7911563084720502070, 0.000000000000000000 ) ) ;
#13853=ORIENTED_EDGE ( 'NONE', *, *, #51571, .T. ) ;
#13857=CIRCLE ( 'NONE', #49445, 0.1418229129680897982 ) ;
#13866=CARTESIAN_POINT ( 'NONE',  ( 38.65784837781280459, 56.65029301956750629, -10.00000000000000000 ) ) ;
#13870=VECTOR ( 'NONE', #55054, 1000.000000000000000 ) ;
#13885=CARTESIAN_POINT ( 'NONE',  ( -72.48190909937208914, 49.06123820388767598, 10.00000000000000000 ) ) ;
#13887=EDGE_LOOP ( 'NONE', ( #33896, #26230, #89016, #75010 ) ) ;
#13890=DIRECTION ( 'NONE',  ( -0.000000000000000000, 0.000000000000000000, 1.000000000000000000 ) ) ;
#13891=AXIS2_PLACEMENT_3D ( 'NONE', #89163, #19709, #18701 ) ;
#13899=PLANE ( 'NONE',  #50306 ) ;
#13907=EDGE_LOOP ( 'NONE', ( #25591, #83308, #23226, #22511 ) ) ;
#13913=DIRECTION ( 'NONE',  ( -0.000000000000000000, 0.000000000000000000, -1.000000000000000000 ) ) ;
#13923=EDGE_CURVE ( 'NONE', #83671, #53015, #70427, .T. ) ;
#13925=EDGE_CURVE ( 'NONE', #17814, #41047, #87208, .T. ) ;
#13931=CARTESIAN_POINT ( 'NONE',  ( -19.65312891409030271, 93.06504152958497400, 177.5919119679930134 ) ) ;
#13939=VECTOR ( 'NONE', #60164, 1000.000000000000000 ) ;
#13942=CARTESIAN_POINT ( 'NONE',  ( 46.99867368304095550, 76.19044720721625197, -10.00000000000000000 ) ) ;
#13943=ORIENTED_EDGE ( 'NONE', *, *, #14414, .F. ) ;
#13947=DIRECTION ( 'NONE',  ( -1.000000000000000000, 0.000000000000000000, 0.000000000000000000 ) ) ;
#13948=AXIS2_PLACEMENT_3D ( 'NONE', #74137, #81263, #13805 ) ;
#13949=PLANE ( 'NONE',  #20467 ) ;
#13952=ORIENTED_EDGE ( 'NONE', *, *, #20471, .F. ) ;
#13964=DIRECTION ( 'NONE',  ( -0.1887253692075926415, 0.9820299053580078263, 0.000000000000000000 ) ) ;
#13969=ADVANCED_FACE ( 'NONE', ( #80071 ), #32922, .F. ) ;
#13970=VECTOR ( 'NONE', #70278, 1000.000000000000114 ) ;
#13971=ORIENTED_EDGE ( 'NONE', *, *, #92441, .F. ) ;
#13972=PLANE ( 'NONE',  #30636 ) ;
#13994=DIRECTION ( 'NONE',  ( 1.000000000000000000, 0.000000000000000000, 0.000000000000000000 ) ) ;
#13996=EDGE_CURVE ( 'NONE', #35708, #5362, #25849, .T. ) ;
#14001=CARTESIAN_POINT ( 'NONE',  ( -27.77457187288641904, 24.79904599702367562, 10.00000000000000000 ) ) ;
#14005=CARTESIAN_POINT ( 'NONE',  ( 48.16808589598787904, 104.3116767361652535, -10.00000000000000000 ) ) ;
#14010=VERTEX_POINT ( 'NONE', #87708 ) ;
#14022=ORIENTED_EDGE ( 'NONE', *, *, #57800, .F. ) ;
#14024=CARTESIAN_POINT ( 'NONE',  ( -25.89332989531674301, 24.59406508915897760, 10.00000000000000000 ) ) ;
#14025=CARTESIAN_POINT ( 'NONE',  ( -19.65312891409030271, 93.06504152958497400, 177.5919119679930134 ) ) ;
#14026=ORIENTED_EDGE ( 'NONE', *, *, #87652, .T. ) ;
#14028=ORIENTED_EDGE ( 'NONE', *, *, #66044, .F. ) ;
#14035=CARTESIAN_POINT ( 'NONE',  ( -52.32156893544651410, 31.15564784356141814, -10.00000000000000000 ) ) ;
#14039=CARTESIAN_POINT ( 'NONE',  ( 36.25628400652970384, 53.06077264917335867, -10.00000000000000000 ) ) ;
#14042=AXIS2_PLACEMENT_3D ( 'NONE', #42443, #64778, #4461 ) ;
#14043=EDGE_CURVE ( 'NONE', #47254, #81234, #83057, .T. ) ;
#14044=VERTEX_POINT ( 'NONE', #67312 ) ;
#14047=LINE ( 'NONE', #4445, #15259 ) ;
#14058=VERTEX_POINT ( 'NONE', #69314 ) ;
#14070=VERTEX_POINT ( 'NONE', #85049 ) ;
#14071=EDGE_CURVE ( 'NONE', #57476, #50548, #92652, .T. ) ;
#14077=CIRCLE ( 'NONE', #69021, 0.1418229129680863287 ) ;
#14082=ORIENTED_EDGE ( 'NONE', *, *, #49998, .F. ) ;
#14086=CARTESIAN_POINT ( 'NONE',  ( 3.722289961109204626, 27.08330320443191752, 177.5919119679930134 ) ) ;
#14099=CARTESIAN_POINT ( 'NONE',  ( -19.65312891409030271, 93.06504152958497400, 177.5919119679930134 ) ) ;
#14105=CIRCLE ( 'NONE', #70722, 70.00000000000001421 ) ;
#14108=CARTESIAN_POINT ( 'NONE',  ( 50.33970617970974359, 92.06352491358971690, 177.5919119679930134 ) ) ;
#14112=ADVANCED_FACE ( 'NONE', ( #44504 ), #14623, .F. ) ;
#14114=AXIS2_PLACEMENT_3D ( 'NONE', #43121, #27467, #58337 ) ;
#14115=EDGE_CURVE ( 'NONE', #8334, #96434, #98746, .T. ) ;
#14125=DIRECTION ( 'NONE',  ( -0.6444573283588950208, 0.7646402761590023189, 0.000000000000000000 ) ) ;
#14129=CARTESIAN_POINT ( 'NONE',  ( -66.69146994933839778, 41.22495595238228105, 177.5919119679930134 ) ) ;
#14130=CARTESIAN_POINT ( 'NONE',  ( 11.80767242186427879, 30.53330575246453904, -10.00000000000000000 ) ) ;
#14131=CARTESIAN_POINT ( 'NONE',  ( 44.95821123098110661, 116.5722627105190270, -10.00000000000000000 ) ) ;
#14135=ORIENTED_EDGE ( 'NONE', *, *, #6838, .F. ) ;
#14137=ORIENTED_EDGE ( 'NONE', *, *, #66124, .F. ) ;
#14141=ORIENTED_EDGE ( 'NONE', *, *, #55410, .F. ) ;
#14146=CARTESIAN_POINT ( 'NONE',  ( -0.2492734796364602656, 27.10516647459198225, -10.00000000000000000 ) ) ;
#14149=ORIENTED_EDGE ( 'NONE', *, *, #90732, .T. ) ;
#14159=ORIENTED_EDGE ( 'NONE', *, *, #88749, .T. ) ;
#14168=CARTESIAN_POINT ( 'NONE',  ( -4.027391858960333693, 36.50819422017340088, 59.99999999999999289 ) ) ;
#14180=CARTESIAN_POINT ( 'NONE',  ( -19.79069005721430230, 93.09954762390393057, 59.99999999999999289 ) ) ;
#14183=ORIENTED_EDGE ( 'NONE', *, *, #18080, .T. ) ;
#14184=FACE_BOUND ( 'NONE', #24149, .T. ) ;
#14191=ORIENTED_EDGE ( 'NONE', *, *, #61393, .F. ) ;
#14192=AXIS2_PLACEMENT_3D ( 'NONE', #53938, #77780, #79317 ) ;
#14195=ORIENTED_EDGE ( 'NONE', *, *, #83693, .T. ) ;
#14201=DIRECTION ( 'NONE',  ( -0.000000000000000000, -0.000000000000000000, -1.000000000000000000 ) ) ;
#14209=ORIENTED_EDGE ( 'NONE', *, *, #76401, .T. ) ;
#14212=AXIS2_PLACEMENT_3D ( 'NONE', #87221, #63839, #39512 ) ;
#14216=CARTESIAN_POINT ( 'NONE',  ( -80.27490717900100492, 58.06504152958491005, 177.5919119679930134 ) ) ;
#14220=AXIS2_PLACEMENT_3D ( 'NONE', #10114, #63809, #48620 ) ;
#14222=AXIS2_PLACEMENT_3D ( 'NONE', #49042, #79976, #41419 ) ;
#14235=CIRCLE ( 'NONE', #20687, 70.00000000000001421 ) ;
#14249=DIRECTION ( 'NONE',  ( 0.7845058662179964504, 0.6201213960746324583, 0.000000000000000000 ) ) ;
#14250=AXIS2_PLACEMENT_3D ( 'NONE', #39295, #77329, #7936 ) ;
#14266=PLANE ( 'NONE',  #74472 ) ;
#14275=VERTEX_POINT ( 'NONE', #2949 ) ;
#14280=VECTOR ( 'NONE', #62560, 1000.000000000000000 ) ;
#14287=ADVANCED_FACE ( 'NONE', ( #10525 ), #4409, .T. ) ;
#14288=CIRCLE ( 'NONE', #4837, 70.00000000000001421 ) ;
#14290=AXIS2_PLACEMENT_3D ( 'NONE', #24390, #29986, #83734 ) ;
#14293=VECTOR ( 'NONE', #90853, 1000.000000000000000 ) ;
#14297=DIRECTION ( 'NONE',  ( 0.000000000000000000, -0.000000000000000000, 1.000000000000000000 ) ) ;
#14299=CARTESIAN_POINT ( 'NONE',  ( -18.14236540235112116, 78.33508314200840061, 13.72324207012383468 ) ) ;
#14300=DIRECTION ( 'NONE',  ( -0.000000000000000000, -0.000000000000000000, 1.000000000000000000 ) ) ;
#14302=VERTEX_POINT ( 'NONE', #3438 ) ;
#14303=ORIENTED_EDGE ( 'NONE', *, *, #33636, .T. ) ;
#14306=DIRECTION ( 'NONE',  ( -1.000000000000000000, 0.000000000000000000, 0.000000000000000000 ) ) ;
#14312=CIRCLE ( 'NONE', #73979, 70.00000000000001421 ) ;
#14314=CARTESIAN_POINT ( 'NONE',  ( -19.24216595772339744, 41.33483386289255890, 59.99999999999999289 ) ) ;
#14323=LINE ( 'NONE', #22418, #52825 ) ;
#14324=CARTESIAN_POINT ( 'NONE',  ( 35.10516808903320651, 74.11552124184515833, 59.99999999999999289 ) ) ;
#14328=VERTEX_POINT ( 'NONE', #27722 ) ;
#14331=VECTOR ( 'NONE', #95400, 1000.000000000000000 ) ;
#14335=CARTESIAN_POINT ( 'NONE',  ( -28.50628834134440126, 40.78531227041054308, 59.99999999999999289 ) ) ;
#14336=CARTESIAN_POINT ( 'NONE',  ( 11.61660434717087043, 51.85354971528389001, 59.99999999999999289 ) ) ;
#14342=DIRECTION ( 'NONE',  ( 0.3074612162317589825, -0.9515606131578205895, 0.000000000000000000 ) ) ;
#14343=ORIENTED_EDGE ( 'NONE', *, *, #80742, .T. ) ;
#14346=CARTESIAN_POINT ( 'NONE',  ( 32.07315653955450330, 47.77038272570916888, 10.00000000000000000 ) ) ;
#14349=EDGE_CURVE ( 'NONE', #38681, #75209, #91047, .T. ) ;
#14353=CIRCLE ( 'NONE', #45080, 70.00000000000001421 ) ;
#14355=EDGE_CURVE ( 'NONE', #62875, #97599, #53489, .T. ) ;
#14374=CIRCLE ( 'NONE', #71017, 70.00000000000001421 ) ;
#14387=ORIENTED_EDGE ( 'NONE', *, *, #90170, .F. ) ;
#14395=CARTESIAN_POINT ( 'NONE',  ( 33.28585168620431745, 96.06718347469407604, 59.99999999999999289 ) ) ;
#14405=LINE ( 'NONE', #39164, #89205 ) ;
#14408=ORIENTED_EDGE ( 'NONE', *, *, #88883, .T. ) ;
#14414=EDGE_CURVE ( 'NONE', #24764, #73348, #82472, .T. ) ;
#14417=CARTESIAN_POINT ( 'NONE',  ( 20.37106723994074997, 58.28585045587018953, 59.99999999999999289 ) ) ;
#14427=VERTEX_POINT ( 'NONE', #75327 ) ;
#14438=ORIENTED_EDGE ( 'NONE', *, *, #73646, .F. ) ;
#14450=CARTESIAN_POINT ( 'NONE',  ( -19.65312891409030271, 93.06504152958497400, 59.99999999999999289 ) ) ;
#14453=AXIS2_PLACEMENT_3D ( 'NONE', #65168, #4884, #95632 ) ;
#14457=PLANE ( 'NONE',  #4664 ) ;
#14463=LINE ( 'NONE', #69142, #37060 ) ;
#14471=DIRECTION ( 'NONE',  ( 0.000000000000000000, -0.000000000000000000, 1.000000000000000000 ) ) ;
#14495=EDGE_CURVE ( 'NONE', #25441, #49704, #24092, .T. ) ;
#14496=CARTESIAN_POINT ( 'NONE',  ( 50.53943819540625526, 89.99351993437284136, -10.00000000000000000 ) ) ;
#14512=VECTOR ( 'NONE', #82434, 1000.000000000000000 ) ;
#14516=ADVANCED_FACE ( 'NONE', ( #17497 ), #93022, .F. ) ;
#14523=CIRCLE ( 'NONE', #45238, 70.00000000000001421 ) ;
#14530=DIRECTION ( 'NONE',  ( -0.000000000000000000, -0.000000000000000000, -1.000000000000000000 ) ) ;
#14542=EDGE_CURVE ( 'NONE', #29044, #14044, #25086, .T. ) ;
#14543=EDGE_CURVE ( 'NONE', #76666, #16524, #39763, .T. ) ;
#14544=AXIS2_PLACEMENT_3D ( 'NONE', #31, #8622, #9121 ) ;
#14546=ORIENTED_EDGE ( 'NONE', *, *, #72666, .F. ) ;
#14549=EDGE_LOOP ( 'NONE', ( #67521, #20126, #38689, #42561 ) ) ;
#14562=EDGE_LOOP ( 'NONE', ( #63093, #55643, #95199, #41335 ) ) ;
#14573=CARTESIAN_POINT ( 'NONE',  ( -69.42640704509901184, 61.99316646242160544, 59.99999999999999289 ) ) ;
#14581=LINE ( 'NONE', #77379, #2538 ) ;
#14594=CARTESIAN_POINT ( 'NONE',  ( -27.12601731895737700, 23.20384585402105770, -10.00000000000000000 ) ) ;
#14595=VECTOR ( 'NONE', #42476, 1000.000000000000114 ) ;
#14603=LINE ( 'NONE', #60171, #70848 ) ;
#14609=EDGE_CURVE ( 'NONE', #20973, #31576, #40276, .T. ) ;
#14623=PLANE ( 'NONE',  #81497 ) ;
#14627=DIRECTION ( 'NONE',  ( -0.5000000000000013323, 0.8660254037844380415, 0.000000000000000000 ) ) ;
#14629=DIRECTION ( 'NONE',  ( -0.000000000000000000, 0.000000000000000000, -1.000000000000000000 ) ) ;
#14634=EDGE_CURVE ( 'NONE', #33594, #82113, #58478, .T. ) ;
#14636=ORIENTED_EDGE ( 'NONE', *, *, #57037, .T. ) ;
#14638=ORIENTED_EDGE ( 'NONE', *, *, #25046, .F. ) ;
#14644=CARTESIAN_POINT ( 'NONE',  ( 32.00866654959714452, 120.8840912179599343, 59.99999999999999289 ) ) ;
#14647=LINE ( 'NONE', #29843, #80587 ) ;
#14650=VERTEX_POINT ( 'NONE', #90941 ) ;
#14660=VERTEX_POINT ( 'NONE', #22483 ) ;
#14678=FACE_BOUND ( 'NONE', #17660, .T. ) ;
#14685=DIRECTION ( 'NONE',  ( 1.000000000000000000, 0.000000000000000000, 0.000000000000000000 ) ) ;
#14686=ORIENTED_EDGE ( 'NONE', *, *, #74528, .F. ) ;
#14702=ORIENTED_EDGE ( 'NONE', *, *, #81736, .T. ) ;
#14717=CARTESIAN_POINT ( 'NONE',  ( 31.12960416526798468, 44.88710030135631257, 177.5919119679930134 ) ) ;
#14718=CARTESIAN_POINT ( 'NONE',  ( -14.06329310883398875, 23.28858607597029007, 10.00000000000000000 ) ) ;
#14720=CARTESIAN_POINT ( 'NONE',  ( 32.24342178309110096, 47.97677246190463052, -10.00000000000000000 ) ) ;
#14722=AXIS2_PLACEMENT_3D ( 'NONE', #26999, #81236, #90331 ) ;
#14725=EDGE_LOOP ( 'NONE', ( #93582, #68270, #68472, #91946 ) ) ;
#14742=EDGE_CURVE ( 'NONE', #3124, #99043, #62572, .T. ) ;
#14748=DIRECTION ( 'NONE',  ( 1.000000000000000000, 0.000000000000000000, 0.000000000000000000 ) ) ;
#14759=CARTESIAN_POINT ( 'NONE',  ( 37.10733492148454360, 81.41235766493377923, 59.99999999999999289 ) ) ;
#14767=CARTESIAN_POINT ( 'NONE',  ( 15.54467260552930341, 34.00295985972734059, -10.00000000000000000 ) ) ;
#14770=EDGE_LOOP ( 'NONE', ( #80188, #26634, #83374, #76057 ) ) ;
#14771=DIRECTION ( 'NONE',  ( 0.000000000000000000, -0.000000000000000000, -1.000000000000000000 ) ) ;
#14772=CARTESIAN_POINT ( 'NONE',  ( -19.65312891409030271, 93.06504152958497400, 177.5919119679930134 ) ) ;
#14781=EDGE_CURVE ( 'NONE', #54956, #38929, #86353, .T. ) ;
#14782=ORIENTED_EDGE ( 'NONE', *, *, #77995, .F. ) ;
#14784=CARTESIAN_POINT ( 'NONE',  ( -32.37721085874458282, 42.92243475195172664, 59.99999999999999289 ) ) ;
#14789=CARTESIAN_POINT ( 'NONE',  ( -10.97633901967424919, 72.03548929155091685, 14.69827683239626381 ) ) ;
#14790=CARTESIAN_POINT ( 'NONE',  ( -54.45295541630240166, 33.76759809053437067, -10.00000000000000000 ) ) ;
#14794=ORIENTED_EDGE ( 'NONE', *, *, #60944, .F. ) ;
#14806=CARTESIAN_POINT ( 'NONE',  ( 49.04287251715432205, 95.72274150194785136, -10.00000000000000000 ) ) ;
#14823=CARTESIAN_POINT ( 'NONE',  ( 50.53943819540625526, 89.99351993437284136, 10.00000000000000000 ) ) ;
#14827=DIRECTION ( 'NONE',  ( 1.000000000000000000, -7.930164461608259453E-16, 0.000000000000000000 ) ) ;
#14837=ADVANCED_FACE ( 'NONE', ( #85445 ), #93020, .F. ) ;
#14841=LINE ( 'NONE', #76650, #38568 ) ;
#14866=FACE_OUTER_BOUND ( 'NONE', #30971, .T. ) ;
#14868=VERTEX_POINT ( 'NONE', #95042 ) ;
#14878=CARTESIAN_POINT ( 'NONE',  ( -73.81593683174931186, 48.72104262922892559, -10.00000000000000000 ) ) ;
#14883=DIRECTION ( 'NONE',  ( -0.000000000000000000, -0.000000000000000000, -1.000000000000000000 ) ) ;
#14890=CYLINDRICAL_SURFACE ( 'NONE', #34525, 70.00000000000002842 ) ;
#14894=EDGE_CURVE ( 'NONE', #1725, #97001, #65093, .T. ) ;
#14902=VERTEX_POINT ( 'NONE', #80854 ) ;
#14904=ORIENTED_EDGE ( 'NONE', *, *, #11465, .T. ) ;
#14908=ORIENTED_EDGE ( 'NONE', *, *, #6783, .F. ) ;
#14918=PLANE ( 'NONE',  #84039 ) ;
#14922=DIRECTION ( 'NONE',  ( -0.8263106059122556912, -0.5632146860273805622, 0.000000000000000000 ) ) ;
#14930=CARTESIAN_POINT ( 'NONE',  ( -40.42249077443059235, 27.53003111760058630, -10.00000000000000000 ) ) ;
#14934=DIRECTION ( 'NONE',  ( 0.000000000000000000, -0.000000000000000000, -1.000000000000000000 ) ) ;
#14943=ADVANCED_FACE ( 'NONE', ( #87966 ), #96046, .F. ) ;
#14948=DIRECTION ( 'NONE',  ( 1.000000000000000000, 0.000000000000000000, 0.000000000000000000 ) ) ;
#14955=EDGE_CURVE ( 'NONE', #38181, #24509, #4286, .T. ) ;
#14960=CARTESIAN_POINT ( 'NONE',  ( -22.20871200244593879, 23.11170711957622004, 10.00000000000000000 ) ) ;
#14967=DIRECTION ( 'NONE',  ( -0.000000000000000000, 0.000000000000000000, -1.000000000000000000 ) ) ;
#14969=CARTESIAN_POINT ( 'NONE',  ( 43.53192288983094471, 62.93782412512172186, -10.00000000000000000 ) ) ;
#14973=DIRECTION ( 'NONE',  ( 0.4527707594502572985, 0.8916269620120498285, 0.000000000000000000 ) ) ;
#14977=DIRECTION ( 'NONE',  ( -1.000000000000000000, 0.000000000000000000, 0.000000000000000000 ) ) ;
#14979=LINE ( 'NONE', #91529, #58171 ) ;
#14986=CARTESIAN_POINT ( 'NONE',  ( -38.35373792487678202, 26.90998726756845727, -10.00000000000000000 ) ) ;
#14987=ORIENTED_EDGE ( 'NONE', *, *, #30883, .F. ) ;
#14992=DIRECTION ( 'NONE',  ( 0.000000000000000000, 0.000000000000000000, 1.000000000000000000 ) ) ;
#14996=CARTESIAN_POINT ( 'NONE',  ( -34.42581292930597670, 25.91608375674935161, -10.00000000000000000 ) ) ;
#14998=VERTEX_POINT ( 'NONE', #95560 ) ;
#15006=CARTESIAN_POINT ( 'NONE',  ( 48.77433535142598231, 99.76555324011610537, -10.00000000000000000 ) ) ;
#15014=DIRECTION ( 'NONE',  ( 0.000000000000000000, 0.000000000000000000, 1.000000000000000000 ) ) ;
#15015=ORIENTED_EDGE ( 'NONE', *, *, #98097, .F. ) ;
#15017=ORIENTED_EDGE ( 'NONE', *, *, #11480, .T. ) ;
#15018=ORIENTED_EDGE ( 'NONE', *, *, #9448, .F. ) ;
#15020=CARTESIAN_POINT ( 'NONE',  ( -41.62359735524142934, 26.60228115600143184, 10.00000000000000000 ) ) ;
#15046=ORIENTED_EDGE ( 'NONE', *, *, #7153, .T. ) ;
#15048=ORIENTED_EDGE ( 'NONE', *, *, #90256, .F. ) ;
#15050=DIRECTION ( 'NONE',  ( -0.8660254037844399289, -0.4999999999999976130, 0.000000000000000000 ) ) ;
#15060=ORIENTED_EDGE ( 'NONE', *, *, #9254, .T. ) ;
#15064=EDGE_CURVE ( 'NONE', #1376, #77230, #88973, .T. ) ;
#15068=DIRECTION ( 'NONE',  ( 0.000000000000000000, 0.000000000000000000, 1.000000000000000000 ) ) ;
#15069=FACE_OUTER_BOUND ( 'NONE', #66109, .T. ) ;
#15075=DIRECTION ( 'NONE',  ( -0.4527707594502665689, -0.8916269620120450545, 0.000000000000000000 ) ) ;
#15078=DIRECTION ( 'NONE',  ( -0.000000000000000000, -0.000000000000000000, 1.000000000000000000 ) ) ;
#15079=EDGE_CURVE ( 'NONE', #78966, #84837, #28582, .T. ) ;
#15092=CARTESIAN_POINT ( 'NONE',  ( 49.28760614098965220, 105.1966139777580338, -10.00000000000000000 ) ) ;
#15110=ORIENTED_EDGE ( 'NONE', *, *, #20664, .F. ) ;
#15125=DIRECTION ( 'NONE',  ( -0.2270762630343793331, 0.9738769792773321887, 0.000000000000000000 ) ) ;
#15127=ORIENTED_EDGE ( 'NONE', *, *, #39516, .T. ) ;
#15129=FACE_OUTER_BOUND ( 'NONE', #80493, .T. ) ;
#15131=DIRECTION ( 'NONE',  ( 1.000000000000000000, 0.000000000000000000, 0.000000000000000000 ) ) ;
#15132=CARTESIAN_POINT ( 'NONE',  ( 24.08514838022782811, 55.05848426107617399, 59.99999999999999289 ) ) ;
#15139=EDGE_CURVE ( 'NONE', #94007, #97001, #89929, .T. ) ;
#15145=DIRECTION ( 'NONE',  ( 0.000000000000000000, 0.000000000000000000, 1.000000000000000000 ) ) ;
#15148=ORIENTED_EDGE ( 'NONE', *, *, #95793, .F. ) ;
#15152=FACE_BOUND ( 'NONE', #70336, .T. ) ;
#15159=DIRECTION ( 'NONE',  ( -0.9607486656258008573, -0.2774202615135435979, 0.000000000000000000 ) ) ;
#15162=ORIENTED_EDGE ( 'NONE', *, *, #99895, .F. ) ;
#15165=EDGE_LOOP ( 'NONE', ( #95589, #17480, #98037, #15341 ) ) ;
#15167=LINE ( 'NONE', #76979, #36853 ) ;
#15169=LINE ( 'NONE', #494, #60658 ) ;
#15170=CARTESIAN_POINT ( 'NONE',  ( 34.97213163436671124, 51.32435524152969464, 10.00000000000000000 ) ) ;
#15187=ORIENTED_EDGE ( 'NONE', *, *, #99295, .T. ) ;
#15188=AXIS2_PLACEMENT_3D ( 'NONE', #100020, #67603, #68598 ) ;
#15192=EDGE_CURVE ( 'NONE', #66165, #15491, #47454, .T. ) ;
#15197=EDGE_CURVE ( 'NONE', #71865, #23641, #42599, .T. ) ;
#15201=DIRECTION ( 'NONE',  ( 0.000000000000000000, -0.000000000000000000, -1.000000000000000000 ) ) ;
#15218=LINE ( 'NONE', #46113, #11275 ) ;
#15239=DIRECTION ( 'NONE',  ( 0.1548189829846108034, -0.9879428538673736826, 0.000000000000000000 ) ) ;
#15241=CARTESIAN_POINT ( 'NONE',  ( 41.25821923120311396, 128.0827283385945918, 10.00000000000000000 ) ) ;
#15248=CIRCLE ( 'NONE', #52436, 0.1418229129681591871 ) ;
#15250=CARTESIAN_POINT ( 'NONE',  ( -19.65312891409030271, 93.06504152958497400, 10.00000000000000888 ) ) ;
#15256=LINE ( 'NONE', #61367, #88860 ) ;
#15257=ORIENTED_EDGE ( 'NONE', *, *, #94219, .T. ) ;
#15259=VECTOR ( 'NONE', #44923, 1000.000000000000341 ) ;
#15260=EDGE_CURVE ( 'NONE', #45441, #99285, #83545, .T. ) ;
#15265=ORIENTED_EDGE ( 'NONE', *, *, #69517, .T. ) ;
#15268=ORIENTED_EDGE ( 'NONE', *, *, #11780, .F. ) ;
#15270=CARTESIAN_POINT ( 'NONE',  ( -4.991637333140347188, 76.62020665819028409, 14.32149113796480577 ) ) ;
#15272=DIRECTION ( 'NONE',  ( -0.7061384650677094976, -0.7080737730998225565, 0.000000000000000000 ) ) ;
#15286=DIRECTION ( 'NONE',  ( -0.5369817302126890235, 0.8435938723211464652, 0.000000000000000000 ) ) ;
#15315=DIRECTION ( 'NONE',  ( 0.000000000000000000, 0.000000000000000000, -1.000000000000000000 ) ) ;
#15316=DIRECTION ( 'NONE',  ( 1.000000000000000000, 0.000000000000000000, 0.000000000000000000 ) ) ;
#15317=CARTESIAN_POINT ( 'NONE',  ( -24.55113401881919089, 60.19361660390018898, -10.00000000000000000 ) ) ;
#15324=AXIS2_PLACEMENT_3D ( 'NONE', #915, #90796, #414 ) ;
#15329=ADVANCED_FACE ( 'NONE', ( #45973 ), #7490, .F. ) ;
#15339=LINE ( 'NONE', #30565, #81286 ) ;
#15341=ORIENTED_EDGE ( 'NONE', *, *, #49055, .F. ) ;
#15354=CARTESIAN_POINT ( 'NONE',  ( 0.000000000000000000, 0.000000000000000000, 0.000000000000000000 ) ) ;
#15370=DIRECTION ( 'NONE',  ( -0.8660254037844390407, -0.4999999999999992228, 0.000000000000000000 ) ) ;
#15376=FACE_OUTER_BOUND ( 'NONE', #94847, .T. ) ;
#15379=LINE ( 'NONE', #62476, #73923 ) ;
#15392=AXIS2_PLACEMENT_3D ( 'NONE', #26519, #73130, #89842 ) ;
#15393=ORIENTED_EDGE ( 'NONE', *, *, #96548, .T. ) ;
#15396=ORIENTED_EDGE ( 'NONE', *, *, #19961, .F. ) ;
#15418=ORIENTED_EDGE ( 'NONE', *, *, #93104, .T. ) ;
#15420=CARTESIAN_POINT ( 'NONE',  ( -6.887318171848119341, 24.23892674679880699, -10.00000000000000000 ) ) ;
#15421=PLANE ( 'NONE',  #38633 ) ;
#15430=CIRCLE ( 'NONE', #41333, 70.00000000000001421 ) ;
#15432=EDGE_LOOP ( 'NONE', ( #21065, #21405, #16540, #80527 ) ) ;
#15433=ORIENTED_EDGE ( 'NONE', *, *, #79059, .F. ) ;
#15434=CARTESIAN_POINT ( 'NONE',  ( 32.30839531297598910, 123.0650415295850593, -25.00000000000000000 ) ) ;
#15438=CARTESIAN_POINT ( 'NONE',  ( -71.36129514276956343, 45.88172302328153052, -10.00000000000000000 ) ) ;
#15447=ADVANCED_FACE ( 'NONE', ( #94635 ), #78928, .F. ) ;
#15452=VECTOR ( 'NONE', #76098, 1000.000000000000000 ) ;
#15461=VERTEX_POINT ( 'NONE', #42378 ) ;
#15462=CIRCLE ( 'NONE', #72132, 70.00000000000001421 ) ;
#15470=DIRECTION ( 'NONE',  ( 0.9963824715083259287, -0.08498217737243619896, 0.000000000000000000 ) ) ;
#15478=DIRECTION ( 'NONE',  ( -0.6602847420308685100, -0.7510153523339117010, 0.000000000000000000 ) ) ;
#15484=CARTESIAN_POINT ( 'NONE',  ( 30.45139999638899653, 75.71324894449729470, 59.99999999999999289 ) ) ;
#15491=VERTEX_POINT ( 'NONE', #18105 ) ;
#15500=CARTESIAN_POINT ( 'NONE',  ( 9.807469842037885854, 42.32143348850679132, 59.99999999999999289 ) ) ;
#15504=DIRECTION ( 'NONE',  ( -1.000000000000000000, 0.000000000000000000, 0.000000000000000000 ) ) ;
#15510=AXIS2_PLACEMENT_3D ( 'NONE', #97926, #27029, #28501 ) ;
#15511=ORIENTED_EDGE ( 'NONE', *, *, #72839, .F. ) ;
#15512=EDGE_LOOP ( 'NONE', ( #1210, #71858, #53994, #14135 ) ) ;
#15518=CARTESIAN_POINT ( 'NONE',  ( -19.65312891409030271, 93.06504152958497400, 177.5919119679930134 ) ) ;
#15529=CIRCLE ( 'NONE', #78631, 0.1418229129680828593 ) ;
#15552=VERTEX_POINT ( 'NONE', #2929 ) ;
#15557=CARTESIAN_POINT ( 'NONE',  ( 40.70814378237798081, 60.14496435084704018, -10.00000000000000000 ) ) ;
#15563=DIRECTION ( 'NONE',  ( 0.000000000000000000, -0.000000000000000000, 1.000000000000000000 ) ) ;
#15571=EDGE_CURVE ( 'NONE', #37717, #90330, #26505, .T. ) ;
#15573=DIRECTION ( 'NONE',  ( 1.000000000000000000, 0.000000000000000000, 0.000000000000000000 ) ) ;
#15574=VECTOR ( 'NONE', #8222, 1000.000000000000000 ) ;
#15577=DIRECTION ( 'NONE',  ( -0.000000000000000000, -0.000000000000000000, -1.000000000000000000 ) ) ;
#15581=AXIS2_PLACEMENT_3D ( 'NONE', #74879, #13573, #53539 ) ;
#15582=LINE ( 'NONE', #78418, #80326 ) ;
#15586=ADVANCED_FACE ( 'NONE', ( #72830 ), #3902, .F. ) ;
#15588=CARTESIAN_POINT ( 'NONE',  ( 48.43557798863805886, 76.81918075477977936, -10.00000000000000000 ) ) ;
#15592=CARTESIAN_POINT ( 'NONE',  ( -19.65312891409030271, 93.06504152958497400, -10.00000000000000888 ) ) ;
#15601=VECTOR ( 'NONE', #91592, 1000.000000000000227 ) ;
#15603=LINE ( 'NONE', #40403, #84602 ) ;
#15614=ORIENTED_EDGE ( 'NONE', *, *, #60944, .T. ) ;
#15620=ORIENTED_EDGE ( 'NONE', *, *, #34946, .F. ) ;
#15621=CARTESIAN_POINT ( 'NONE',  ( -19.51228460464733416, 93.04840965836413602, 59.99999999999999289 ) ) ;
#15624=ORIENTED_EDGE ( 'NONE', *, *, #91376, .T. ) ;
#15631=ORIENTED_EDGE ( 'NONE', *, *, #23766, .T. ) ;
#15639=DIRECTION ( 'NONE',  ( 1.000000000000000000, 0.000000000000000000, 0.000000000000000000 ) ) ;
#15651=CARTESIAN_POINT ( 'NONE',  ( -8.406493707509316238, 25.24382671950691304, 10.00000000000000000 ) ) ;
#15652=AXIS2_PLACEMENT_3D ( 'NONE', #79935, #88551, #96632 ) ;
#15664=CARTESIAN_POINT ( 'NONE',  ( -67.91103796225580425, 44.10201266000169795, -10.00000000000000000 ) ) ;
#15669=ORIENTED_EDGE ( 'NONE', *, *, #67651, .F. ) ;
#15671=LINE ( 'NONE', #84140, #80296 ) ;
#15672=ORIENTED_EDGE ( 'NONE', *, *, #72839, .T. ) ;
#15681=VECTOR ( 'NONE', #64904, 1000.000000000000114 ) ;
#15684=DIRECTION ( 'NONE',  ( 0.9981280818701453450, 0.06115825522547521653, 0.000000000000000000 ) ) ;
#15691=PLANE ( 'NONE',  #98066 ) ;
#15702=EDGE_CURVE ( 'NONE', #45792, #59362, #48888, .T. ) ;
#15705=DIRECTION ( 'NONE',  ( -0.000000000000000000, -0.000000000000000000, 1.000000000000000000 ) ) ;
#15712=DIRECTION ( 'NONE',  ( -1.000000000000000000, 0.000000000000000000, 0.000000000000000000 ) ) ;
#15721=VECTOR ( 'NONE', #27752, 1000.000000000000000 ) ;
#15726=ADVANCED_FACE ( 'NONE', ( #80321 ), #41767, .F. ) ;
#15727=VECTOR ( 'NONE', #87673, 1000.000000000000000 ) ;
#15742=AXIS2_PLACEMENT_3D ( 'NONE', #33356, #62233, #95207 ) ;
#15749=VERTEX_POINT ( 'NONE', #19510 ) ;
#15750=CARTESIAN_POINT ( 'NONE',  ( 23.64814127513161068, 118.0650415295850308, 40.00000000000000000 ) ) ;
#15757=VECTOR ( 'NONE', #94283, 1000.000000000000114 ) ;
#15760=ORIENTED_EDGE ( 'NONE', *, *, #81804, .T. ) ;
#15762=DIRECTION ( 'NONE',  ( 0.2398044646550112069, 0.9708212084269294273, 0.000000000000000000 ) ) ;
#15767=ADVANCED_FACE ( 'NONE', ( #80837 ), #50368, .T. ) ;
#15768=EDGE_CURVE ( 'NONE', #90969, #70646, #34669, .T. ) ;
#15769=VERTEX_POINT ( 'NONE', #73684 ) ;
#15777=VERTEX_POINT ( 'NONE', #64079 ) ;
#15778=CARTESIAN_POINT ( 'NONE',  ( -4.653128914090328472, 78.33390353417378549, 13.90751606465751777 ) ) ;
#15780=DIRECTION ( 'NONE',  ( 1.000000000000000000, 0.000000000000000000, 0.000000000000000000 ) ) ;
#15781=LINE ( 'NONE', #7692, #62456 ) ;
#15783=VERTEX_POINT ( 'NONE', #35669 ) ;
#15784=DIRECTION ( 'NONE',  ( -0.9347244501068304734, -0.3553733281669903543, 0.000000000000000000 ) ) ;
#15785=PLANE ( 'NONE',  #84954 ) ;
#15787=VECTOR ( 'NONE', #4892, 1000.000000000000000 ) ;
#15800=AXIS2_PLACEMENT_3D ( 'NONE', #13161, #28846, #44014 ) ;
#15806=PLANE ( 'NONE',  #66774 ) ;
#15828=CARTESIAN_POINT ( 'NONE',  ( -19.65312891409030271, 93.06504152958497400, 60.00000000000000000 ) ) ;
#15836=ADVANCED_FACE ( 'NONE', ( #12898 ), #82329, .F. ) ;
#15841=CARTESIAN_POINT ( 'NONE',  ( 45.88188149789386472, 72.29567966924399514, 10.00000000000000000 ) ) ;
#15842=FACE_OUTER_BOUND ( 'NONE', #59445, .T. ) ;
#15864=VERTEX_POINT ( 'NONE', #99479 ) ;
#15865=DIRECTION ( 'NONE',  ( 0.000000000000000000, 0.000000000000000000, 1.000000000000000000 ) ) ;
#15880=EDGE_LOOP ( 'NONE', ( #43705, #10807, #51572, #57771 ) ) ;
#15882=CARTESIAN_POINT ( 'NONE',  ( 21.15788363470973366, 37.74176219324819215, 10.00000000000000000 ) ) ;
#15887=ORIENTED_EDGE ( 'NONE', *, *, #67637, .F. ) ;
#15888=CARTESIAN_POINT ( 'NONE',  ( -19.65312891409030271, 93.06504152958497400, 177.5919119679930134 ) ) ;
#15891=EDGE_CURVE ( 'NONE', #43419, #38467, #57710, .T. ) ;
#15895=ORIENTED_EDGE ( 'NONE', *, *, #26890, .T. ) ;
#15901=ORIENTED_EDGE ( 'NONE', *, *, #100085, .F. ) ;
#15907=DIRECTION ( 'NONE',  ( -0.000000000000000000, 0.000000000000000000, -1.000000000000000000 ) ) ;
#15908=VERTEX_POINT ( 'NONE', #23690 ) ;
#15910=VECTOR ( 'NONE', #13655, 1000.000000000000000 ) ;
#15917=FACE_OUTER_BOUND ( 'NONE', #63871, .T. ) ;
#15923=ORIENTED_EDGE ( 'NONE', *, *, #54019, .F. ) ;
#15925=DIRECTION ( 'NONE',  ( -1.000000000000000000, -9.785293164091933533E-14, 0.000000000000000000 ) ) ;
#15929=EDGE_CURVE ( 'NONE', #17145, #22043, #45760, .T. ) ;
#15932=EDGE_LOOP ( 'NONE', ( #7580, #9185, #65774, #51167 ) ) ;
#15936=EDGE_CURVE ( 'NONE', #69110, #23277, #77427, .T. ) ;
#15940=CIRCLE ( 'NONE', #11205, 11.89249999999999652 ) ;
#15943=VECTOR ( 'NONE', #26428, 1000.000000000000000 ) ;
#15948=ORIENTED_EDGE ( 'NONE', *, *, #84676, .T. ) ;
#15949=AXIS2_PLACEMENT_3D ( 'NONE', #9932, #31206, #62597 ) ;
#15950=VERTEX_POINT ( 'NONE', #45985 ) ;
#15964=VECTOR ( 'NONE', #46095, 1000.000000000000000 ) ;
#15978=PLANE ( 'NONE',  #90085 ) ;
#15987=DIRECTION ( 'NONE',  ( -1.000000000000000000, 0.000000000000000000, 0.000000000000000000 ) ) ;
#15996=CARTESIAN_POINT ( 'NONE',  ( 30.80155721116056355, 46.36891074996812989, -10.00000000000000000 ) ) ;
#16005=DIRECTION ( 'NONE',  ( -0.4805540241036398430, -0.8769651246872924855, 0.000000000000000000 ) ) ;
#16007=EDGE_CURVE ( 'NONE', #24573, #29268, #63209, .T. ) ;
#16022=VECTOR ( 'NONE', #43217, 1000.000000000000000 ) ;
#16029=VERTEX_POINT ( 'NONE', #85043 ) ;
#16031=VECTOR ( 'NONE', #65607, 999.9999999999998863 ) ;
#16034=PLANE ( 'NONE',  #84801 ) ;
#16040=DIRECTION ( 'NONE',  ( -1.000000000000000000, 0.000000000000000000, 0.000000000000000000 ) ) ;
#16048=EDGE_LOOP ( 'NONE', ( #69460, #32230, #25895, #72622 ) ) ;
#16052=CARTESIAN_POINT ( 'NONE',  ( -12.68721568607400485, 24.67147432707382748, -10.00000000000000000 ) ) ;
#16059=VERTEX_POINT ( 'NONE', #53598 ) ;
#16062=ORIENTED_EDGE ( 'NONE', *, *, #13762, .F. ) ;
#16076=CARTESIAN_POINT ( 'NONE',  ( 2.814886498931689296, 38.86145383009443321, 59.99999999999999289 ) ) ;
#16087=VECTOR ( 'NONE', #26217, 1000.000000000000000 ) ;
#16098=EDGE_CURVE ( 'NONE', #10423, #17015, #9530, .T. ) ;
#16103=VECTOR ( 'NONE', #61095, 1000.000000000000000 ) ;
#16105=ADVANCED_FACE ( 'NONE', ( #71834 ), #41903, .F. ) ;
#16107=DIRECTION ( 'NONE',  ( -1.000000000000000000, 0.000000000000000000, 0.000000000000000000 ) ) ;
#16109=DIRECTION ( 'NONE',  ( 1.000000000000000000, 4.999968693044007408E-13, 0.000000000000000000 ) ) ;
#16113=CARTESIAN_POINT ( 'NONE',  ( 44.44706364856356373, 64.93738052781137071, 177.5919119679930134 ) ) ;
#16114=AXIS2_PLACEMENT_3D ( 'NONE', #12535, #97164, #27730 ) ;
#16123=FACE_OUTER_BOUND ( 'NONE', #76108, .T. ) ;
#16129=ORIENTED_EDGE ( 'NONE', *, *, #10322, .F. ) ;
#16132=ORIENTED_EDGE ( 'NONE', *, *, #69593, .T. ) ;
#16141=FACE_OUTER_BOUND ( 'NONE', #37914, .T. ) ;
#16142=ORIENTED_EDGE ( 'NONE', *, *, #43882, .F. ) ;
#16158=PLANE ( 'NONE',  #70696 ) ;
#16161=AXIS2_PLACEMENT_3D ( 'NONE', #55278, #78114, #76607 ) ;
#16181=ADVANCED_FACE ( 'NONE', ( #95670 ), #64209, .F. ) ;
#16183=ORIENTED_EDGE ( 'NONE', *, *, #64204, .T. ) ;
#16187=EDGE_CURVE ( 'NONE', #8050, #58060, #56088, .T. ) ;
#16191=CYLINDRICAL_SURFACE ( 'NONE', #4061, 70.00000000000002842 ) ;
#16193=ORIENTED_EDGE ( 'NONE', *, *, #67692, .T. ) ;
#16195=DIRECTION ( 'NONE',  ( -0.000000000000000000, 0.000000000000000000, 1.000000000000000000 ) ) ;
#16196=CARTESIAN_POINT ( 'NONE',  ( 47.05668214639808866, 76.45164061169337799, -10.00000000000000000 ) ) ;
#16198=FACE_OUTER_BOUND ( 'NONE', #37089, .T. ) ;
#16203=CARTESIAN_POINT ( 'NONE',  ( 15.54467260552930341, 34.00295985972733348, -10.00000000000000000 ) ) ;
#16207=EDGE_LOOP ( 'NONE', ( #18482, #15048, #95457, #65736 ) ) ;
#16214=EDGE_CURVE ( 'NONE', #57637, #89739, #3434, .T. ) ;
#16225=AXIS2_PLACEMENT_3D ( 'NONE', #88089, #71847, #95174 ) ;
#16228=CARTESIAN_POINT ( 'NONE',  ( -19.65312891409030271, 93.06504152958497400, -10.00000000000000888 ) ) ;
#16259=EDGE_LOOP ( 'NONE', ( #63860, #39585, #4981, #58759 ) ) ;
#16264=ORIENTED_EDGE ( 'NONE', *, *, #35895, .T. ) ;
#16278=CARTESIAN_POINT ( 'NONE',  ( -19.65312891409030271, 93.06504152958497400, -10.00000000000000888 ) ) ;
#16283=DIRECTION ( 'NONE',  ( -0.8615733660689046669, -0.5076330711061851630, 0.000000000000000000 ) ) ;
#16284=EDGE_CURVE ( 'NONE', #78948, #41197, #46889, .T. ) ;
#16287=DIRECTION ( 'NONE',  ( -1.000000000000000000, 0.000000000000000000, 0.000000000000000000 ) ) ;
#16296=ORIENTED_EDGE ( 'NONE', *, *, #94321, .T. ) ;
#16300=CARTESIAN_POINT ( 'NONE',  ( 49.07456115661582174, 91.13648234292965356, -10.00000000000000000 ) ) ;
#16319=CIRCLE ( 'NONE', #35703, 70.00000000000001421 ) ;
#16336=DIRECTION ( 'NONE',  ( -0.2502735827033041316, -0.9681751565707789053, 0.000000000000000000 ) ) ;
#16337=DIRECTION ( 'NONE',  ( -1.000000000000000000, 0.000000000000000000, 0.000000000000000000 ) ) ;
#16338=DIRECTION ( 'NONE',  ( -0.9377374661009826307, -0.3473448497826164827, 0.000000000000000000 ) ) ;
#16342=ADVANCED_FACE ( 'NONE', ( #96532 ), #18008, .F. ) ;
#16346=EDGE_CURVE ( 'NONE', #58893, #32206, #10905, .T. ) ;
#16352=CARTESIAN_POINT ( 'NONE',  ( -70.89022602266993545, 47.22876919346843749, -10.00000000000000000 ) ) ;
#16355=DIRECTION ( 'NONE',  ( 0.000000000000000000, 0.000000000000000000, 1.000000000000000000 ) ) ;
#16359=FACE_OUTER_BOUND ( 'NONE', #94069, .T. ) ;
#16361=ORIENTED_EDGE ( 'NONE', *, *, #70034, .F. ) ;
#16369=DIRECTION ( 'NONE',  ( 0.000000000000000000, 0.000000000000000000, 1.000000000000000000 ) ) ;
#16375=LINE ( 'NONE', #25475, #64927 ) ;
#16382=DIRECTION ( 'NONE',  ( 0.000000000000000000, -0.000000000000000000, 1.000000000000000000 ) ) ;
#16383=CARTESIAN_POINT ( 'NONE',  ( -19.65312891409030271, 93.06504152958497400, -10.00000000000000888 ) ) ;
#16386=CIRCLE ( 'NONE', #47186, 0.1418229129681557177 ) ;
#16388=ORIENTED_EDGE ( 'NONE', *, *, #95050, .T. ) ;
#16402=CARTESIAN_POINT ( 'NONE',  ( -38.61298035630893111, 26.97617139035147460, -10.00000000000000000 ) ) ;
#16406=ORIENTED_EDGE ( 'NONE', *, *, #51647, .F. ) ;
#16411=VERTEX_POINT ( 'NONE', #40270 ) ;
#16413=CARTESIAN_POINT ( 'NONE',  ( 49.66226845319755512, 83.29899382260626339, -10.00000000000000000 ) ) ;
#16415=CARTESIAN_POINT ( 'NONE',  ( -19.63800298229563523, 92.92402754151969191, 59.99999999999999289 ) ) ;
#16431=ADVANCED_FACE ( 'NONE', ( #50383 ), #95036, .F. ) ;
#16437=DIRECTION ( 'NONE',  ( 0.7646402761589956576, 0.6444573283589029034, 0.000000000000000000 ) ) ;
#16442=CARTESIAN_POINT ( 'NONE',  ( 50.37091257173480585, 98.81520120758277415, 10.00000000000000000 ) ) ;
#16445=DIRECTION ( 'NONE',  ( 0.1887253692075823441, -0.9820299053580097137, 0.000000000000000000 ) ) ;
#16460=ORIENTED_EDGE ( 'NONE', *, *, #7400, .T. ) ;
#16462=EDGE_CURVE ( 'NONE', #58717, #8050, #69993, .T. ) ;
#16471=EDGE_CURVE ( 'NONE', #80971, #74122, #20000, .T. ) ;
#16478=VERTEX_POINT ( 'NONE', #25336 ) ;
#16479=CARTESIAN_POINT ( 'NONE',  ( -14.67426454553563708, 35.33509950918588061, 59.99999999999999289 ) ) ;
#16485=LINE ( 'NONE', #94526, #29005 ) ;
#16490=DIRECTION ( 'NONE',  ( 1.000000000000000000, -1.189524669241238790E-13, 0.000000000000000000 ) ) ;
#16496=CARTESIAN_POINT ( 'NONE',  ( -19.65312891409030271, 93.06504152958497400, 10.00000000000000888 ) ) ;
#16498=ORIENTED_EDGE ( 'NONE', *, *, #35836, .T. ) ;
#16504=LINE ( 'NONE', #802, #27403 ) ;
#16511=CARTESIAN_POINT ( 'NONE',  ( -44.49648453423614569, 28.96346851210257967, -10.00000000000000000 ) ) ;
#16513=ORIENTED_EDGE ( 'NONE', *, *, #20961, .T. ) ;
#16521=ORIENTED_EDGE ( 'NONE', *, *, #7043, .T. ) ;
#16524=VERTEX_POINT ( 'NONE', #22476 ) ;
#16526=ORIENTED_EDGE ( 'NONE', *, *, #46324, .F. ) ;
#16533=LINE ( 'NONE', #70737, #39944 ) ;
#16537=EDGE_CURVE ( 'NONE', #22359, #33337, #16637, .T. ) ;
#16540=ORIENTED_EDGE ( 'NONE', *, *, #67351, .F. ) ;
#16561=DIRECTION ( 'NONE',  ( 1.000000000000000000, 0.000000000000000000, 0.000000000000000000 ) ) ;
#16573=DIRECTION ( 'NONE',  ( 0.000000000000000000, 0.000000000000000000, 1.000000000000000000 ) ) ;
#16580=ADVANCED_FACE ( 'NONE', ( #14866 ), #40526, .T. ) ;
#16586=LINE ( 'NONE', #71308, #5869 ) ;
#16592=LINE ( 'NONE', #18102, #100140 ) ;
#16607=EDGE_CURVE ( 'NONE', #6688, #78977, #76679, .T. ) ;
#16627=ORIENTED_EDGE ( 'NONE', *, *, #11154, .T. ) ;
#16633=ORIENTED_EDGE ( 'NONE', *, *, #42572, .F. ) ;
#16637=CIRCLE ( 'NONE', #26336, 70.00000000000001421 ) ;
#16643=VECTOR ( 'NONE', #16382, 1000.000000000000000 ) ;
#16648=ORIENTED_EDGE ( 'NONE', *, *, #58669, .T. ) ;
#16658=VECTOR ( 'NONE', #93679, 1000.000000000000000 ) ;
#16661=ORIENTED_EDGE ( 'NONE', *, *, #9635, .F. ) ;
#16666=ORIENTED_EDGE ( 'NONE', *, *, #23575, .F. ) ;
#16667=VERTEX_POINT ( 'NONE', #32934 ) ;
#16671=CARTESIAN_POINT ( 'NONE',  ( -19.65312891409030271, 93.06504152958497400, 59.99999999999999289 ) ) ;
#16672=CARTESIAN_POINT ( 'NONE',  ( -48.10310308390612022, 75.88598450110713145, -10.00000000000000000 ) ) ;
#16681=EDGE_CURVE ( 'NONE', #40696, #81604, #23658, .T. ) ;
#16690=ORIENTED_EDGE ( 'NONE', *, *, #81302, .T. ) ;
#16695=CARTESIAN_POINT ( 'NONE',  ( -11.40312891409031693, 78.77562236714182120, 59.99999999999999289 ) ) ;
#16699=CARTESIAN_POINT ( 'NONE',  ( 49.91331508509971115, 100.8438505198844553, -10.00000000000000000 ) ) ;
#16707=VECTOR ( 'NONE', #66705, 999.9999999999998863 ) ;
#16720=ORIENTED_EDGE ( 'NONE', *, *, #12481, .F. ) ;
#16727=EDGE_CURVE ( 'NONE', #49424, #26012, #11819, .T. ) ;
#16728=CARTESIAN_POINT ( 'NONE',  ( -11.40312891409031693, 78.77562236714182120, 59.99999999999999289 ) ) ;
#16736=CARTESIAN_POINT ( 'NONE',  ( -35.89898968889473707, 24.97633462685642414, 177.5919119679930134 ) ) ;
#16742=LINE ( 'NONE', #35816, #79567 ) ;
#16749=LINE ( 'NONE', #71968, #64998 ) ;
#16754=VERTEX_POINT ( 'NONE', #31269 ) ;
#16757=ORIENTED_EDGE ( 'NONE', *, *, #42541, .T. ) ;
#16766=VERTEX_POINT ( 'NONE', #93102 ) ;
#16774=AXIS2_PLACEMENT_3D ( 'NONE', #66345, #58723, #89698 ) ;
#16775=VERTEX_POINT ( 'NONE', #58791 ) ;
#16776=DIRECTION ( 'NONE',  ( 1.000000000000000000, 1.070572202317114942E-14, 0.000000000000000000 ) ) ;
#16793=LINE ( 'NONE', #77618, #70382 ) ;
#16795=ORIENTED_EDGE ( 'NONE', *, *, #97129, .F. ) ;
#16799=ADVANCED_FACE ( 'NONE', ( #48987 ), #24671, .T. ) ;
#16808=ORIENTED_EDGE ( 'NONE', *, *, #88403, .T. ) ;
#16824=CARTESIAN_POINT ( 'NONE',  ( -19.65312891409030271, 93.06504152958497400, -25.00000000000000000 ) ) ;
#16827=ORIENTED_EDGE ( 'NONE', *, *, #60630, .F. ) ;
#16832=PLANE ( 'NONE',  #67763 ) ;
#16840=DIRECTION ( 'NONE',  ( 0.3002896333693371722, 0.9538480676139722281, 0.000000000000000000 ) ) ;
#16864=ADVANCED_FACE ( 'NONE', ( #87558 ), #71296, .T. ) ;
#16867=AXIS2_PLACEMENT_3D ( 'NONE', #93693, #24256, #55133 ) ;
#16877=EDGE_CURVE ( 'NONE', #88681, #33594, #1888, .T. ) ;
#16878=DIRECTION ( 'NONE',  ( -0.000000000000000000, 0.000000000000000000, -1.000000000000000000 ) ) ;
#16884=ORIENTED_EDGE ( 'NONE', *, *, #66791, .T. ) ;
#16892=CARTESIAN_POINT ( 'NONE',  ( 11.80767242186427879, 30.53330575246453904, 10.00000000000000000 ) ) ;
#16895=DIRECTION ( 'NONE',  ( -0.001635407438350354676, -0.9999986627203610867, 0.000000000000000000 ) ) ;
#16900=EDGE_CURVE ( 'NONE', #31576, #64281, #48485, .T. ) ;
#16902=VERTEX_POINT ( 'NONE', #79426 ) ;
#16907=ORIENTED_EDGE ( 'NONE', *, *, #97400, .T. ) ;
#16922=ADVANCED_FACE ( 'NONE', ( #20093 ), #50467, .F. ) ;
#16923=CARTESIAN_POINT ( 'NONE',  ( 35.03822396736671152, 49.37458582131907292, 10.00000000000000000 ) ) ;
#16926=CARTESIAN_POINT ( 'NONE',  ( 48.61286661847091040, 84.94359857078811160, -10.00000000000000000 ) ) ;
#16931=CARTESIAN_POINT ( 'NONE',  ( 3.076650163567010932, 38.97070005862290287, 59.99999999999999289 ) ) ;
#16945=VERTEX_POINT ( 'NONE', #66668 ) ;
#16956=VECTOR ( 'NONE', #22223, 1000.000000000000114 ) ;
#16964=EDGE_CURVE ( 'NONE', #61138, #62301, #30228, .T. ) ;
#16967=CARTESIAN_POINT ( 'NONE',  ( -19.42194755839791753, 24.31068691715150010, -10.00000000000000000 ) ) ;
#16972=LINE ( 'NONE', #9387, #70836 ) ;
#16977=DIRECTION ( 'NONE',  ( 1.000000000000000000, 0.000000000000000000, 0.000000000000000000 ) ) ;
#16985=DIRECTION ( 'NONE',  ( -0.7510153523339117010, 0.6602847420308685100, 0.000000000000000000 ) ) ;
#16990=ADVANCED_FACE ( 'NONE', ( #6374 ), #68156, .F. ) ;
#17003=EDGE_LOOP ( 'NONE', ( #92932, #10575, #50033, #51049 ) ) ;
#17007=ORIENTED_EDGE ( 'NONE', *, *, #90170, .T. ) ;
#17009=CARTESIAN_POINT ( 'NONE',  ( 44.95821123098110661, 116.5722627105190270, 10.00000000000000000 ) ) ;
#17012=CARTESIAN_POINT ( 'NONE',  ( -30.18034446749236821, 25.12100238203590763, 10.00000000000000000 ) ) ;
#17015=VERTEX_POINT ( 'NONE', #22059 ) ;
#17022=CARTESIAN_POINT ( 'NONE',  ( 30.62489312496363425, 46.16797101519271962, -10.00000000000000000 ) ) ;
#17025=VERTEX_POINT ( 'NONE', #29178 ) ;
#17026=ADVANCED_FACE ( 'NONE', ( #45833 ), #44357, .F. ) ;
#17035=EDGE_CURVE ( 'NONE', #10907, #93808, #91011, .T. ) ;
#17041=DIRECTION ( 'NONE',  ( 0.000000000000000000, 0.000000000000000000, 1.000000000000000000 ) ) ;
#17042=EDGE_LOOP ( 'NONE', ( #5584, #87496, #31677, #60742 ) ) ;
#17053=ORIENTED_EDGE ( 'NONE', *, *, #72853, .T. ) ;
#17057=DIRECTION ( 'NONE',  ( -1.000000000000000000, 0.000000000000000000, 0.000000000000000000 ) ) ;
#17065=ORIENTED_EDGE ( 'NONE', *, *, #40547, .T. ) ;
#17069=CARTESIAN_POINT ( 'NONE',  ( -19.65312891409030271, 93.06504152958497400, 25.00000000000000000 ) ) ;
#17087=CARTESIAN_POINT ( 'NONE',  ( 23.64814127513158937, 118.0650415295850451, 45.00000000000000711 ) ) ;
#17096=DIRECTION ( 'NONE',  ( 0.000000000000000000, 0.000000000000000000, 1.000000000000000000 ) ) ;
#17098=EDGE_CURVE ( 'NONE', #86003, #28497, #99804, .T. ) ;
#17104=AXIS2_PLACEMENT_3D ( 'NONE', #52671, #13696, #37963 ) ;
#17116=AXIS2_PLACEMENT_3D ( 'NONE', #69864, #17166, #77986 ) ;
#17117=EDGE_CURVE ( 'NONE', #50533, #60486, #75289, .T. ) ;
#17118=CARTESIAN_POINT ( 'NONE',  ( 34.97213163436671124, 51.32435524152969464, -10.00000000000000000 ) ) ;
#17126=ORIENTED_EDGE ( 'NONE', *, *, #30617, .F. ) ;
#17129=DIRECTION ( 'NONE',  ( -0.03304531753666253152, -0.9994538543569188027, 0.000000000000000000 ) ) ;
#17131=CARTESIAN_POINT ( 'NONE',  ( -19.65312891409030271, 93.06504152958497400, 40.00000000000000000 ) ) ;
#17138=AXIS2_PLACEMENT_3D ( 'NONE', #72811, #49469, #41870 ) ;
#17145=VERTEX_POINT ( 'NONE', #6857 ) ;
#17149=LINE ( 'NONE', #57640, #86421 ) ;
#17158=EDGE_LOOP ( 'NONE', ( #63515, #71640, #57523, #39147 ) ) ;
#17166=DIRECTION ( 'NONE',  ( -0.7713848165480218233, 0.6363689690731114679, 0.000000000000000000 ) ) ;
#17175=VERTEX_POINT ( 'NONE', #13485 ) ;
#17176=DIRECTION ( 'NONE',  ( -0.000000000000000000, -0.000000000000000000, -1.000000000000000000 ) ) ;
#17177=VECTOR ( 'NONE', #27134, 1000.000000000000000 ) ;
#17180=VERTEX_POINT ( 'NONE', #69148 ) ;
#17181=CIRCLE ( 'NONE', #12366, 0.1418229129681522482 ) ;
#17208=CARTESIAN_POINT ( 'NONE',  ( -61.61048871844075592, 38.59675092633816007, -10.00000000000000000 ) ) ;
#17225=FACE_OUTER_BOUND ( 'NONE', #25623, .T. ) ;
#17238=FACE_OUTER_BOUND ( 'NONE', #23216, .T. ) ;
#17240=ORIENTED_EDGE ( 'NONE', *, *, #68513, .T. ) ;
#17241=DIRECTION ( 'NONE',  ( -0.07193265315672570104, 0.9974094913373514615, 0.000000000000000000 ) ) ;
#17243=CARTESIAN_POINT ( 'NONE',  ( -52.33464467766007289, 32.58262665401804270, 10.00000000000000000 ) ) ;
#17252=VECTOR ( 'NONE', #56012, 1000.000000000000114 ) ;
#17255=CARTESIAN_POINT ( 'NONE',  ( 42.55121439978241682, 60.39930420098813357, -10.00000000000000000 ) ) ;
#17264=ORIENTED_EDGE ( 'NONE', *, *, #52200, .F. ) ;
#17269=EDGE_LOOP ( 'NONE', ( #18273, #11209 ) ) ;
#17280=ORIENTED_EDGE ( 'NONE', *, *, #25840, .F. ) ;
#17290=ORIENTED_EDGE ( 'NONE', *, *, #33756, .F. ) ;
#17294=DIRECTION ( 'NONE',  ( 1.000000000000000000, 0.000000000000000000, 0.000000000000000000 ) ) ;
#17295=VERTEX_POINT ( 'NONE', #5742 ) ;
#17307=CARTESIAN_POINT ( 'NONE',  ( -19.65312891409030271, 93.06504152958497400, 10.00000000000000888 ) ) ;
#17326=VECTOR ( 'NONE', #29054, 999.9999999999998863 ) ;
#17327=VECTOR ( 'NONE', #74378, 1000.000000000000114 ) ;
#17334=CARTESIAN_POINT ( 'NONE',  ( -19.65312891409030271, 93.06504152958497400, 177.5919119679930134 ) ) ;
#17345=CIRCLE ( 'NONE', #10940, 70.00000000000001421 ) ;
#17359=VECTOR ( 'NONE', #81336, 1000.000000000000000 ) ;
#17379=CARTESIAN_POINT ( 'NONE',  ( -78.10577900106846982, 54.55156729251706338, 177.5919119679930134 ) ) ;
#17388=DIRECTION ( 'NONE',  ( 0.06115825522547173321, -0.9981280818701455670, 0.000000000000000000 ) ) ;
#17393=ORIENTED_EDGE ( 'NONE', *, *, #5131, .F. ) ;
#17396=VECTOR ( 'NONE', #73758, 999.9999999999998863 ) ;
#17398=ORIENTED_EDGE ( 'NONE', *, *, #44947, .T. ) ;
#17401=CIRCLE ( 'NONE', #25508, 70.00000000000001421 ) ;
#17405=EDGE_LOOP ( 'NONE', ( #86185, #64093, #21545, #78148 ) ) ;
#17407=PLANE ( 'NONE',  #33685 ) ;
#17409=ORIENTED_EDGE ( 'NONE', *, *, #36134, .F. ) ;
#17411=VERTEX_POINT ( 'NONE', #70528 ) ;
#17413=VERTEX_POINT ( 'NONE', #86295 ) ;
#17421=ORIENTED_EDGE ( 'NONE', *, *, #70534, .F. ) ;
#17432=DIRECTION ( 'NONE',  ( 0.000000000000000000, 0.000000000000000000, 1.000000000000000000 ) ) ;
#17434=DIRECTION ( 'NONE',  ( 1.000000000000000000, 0.000000000000000000, 0.000000000000000000 ) ) ;
#17440=CARTESIAN_POINT ( 'NONE',  ( -19.65312891409030271, 93.06504152958497400, 177.5919119679930134 ) ) ;
#17443=DIRECTION ( 'NONE',  ( 0.000000000000000000, 0.000000000000000000, 1.000000000000000000 ) ) ;
#17448=CARTESIAN_POINT ( 'NONE',  ( 26.60956029314639082, 56.97371141178327747, 59.99999999999999289 ) ) ;
#17454=ORIENTED_EDGE ( 'NONE', *, *, #41816, .T. ) ;
#17459=CARTESIAN_POINT ( 'NONE',  ( -57.88150100324660485, 35.92665207732902388, 10.00000000000000000 ) ) ;
#17464=CYLINDRICAL_SURFACE ( 'NONE', #28555, 70.00000000000002842 ) ;
#17465=VERTEX_POINT ( 'NONE', #40618 ) ;
#17470=AXIS2_PLACEMENT_3D ( 'NONE', #45629, #52247, #97386 ) ;
#17475=EDGE_CURVE ( 'NONE', #39911, #41051, #63436, .T. ) ;
#17480=ORIENTED_EDGE ( 'NONE', *, *, #89306, .F. ) ;
#17486=EDGE_CURVE ( 'NONE', #42311, #5196, #39608, .T. ) ;
#17488=AXIS2_PLACEMENT_3D ( 'NONE', #69480, #583, #47668 ) ;
#17497=FACE_OUTER_BOUND ( 'NONE', #67890, .T. ) ;
#17499=CARTESIAN_POINT ( 'NONE',  ( -33.66737166714137430, 24.21715323669988607, 10.00000000000000000 ) ) ;
#17504=DIRECTION ( 'NONE',  ( -0.000000000000000000, 0.000000000000000000, -1.000000000000000000 ) ) ;
#17505=LINE ( 'NONE', #40784, #80908 ) ;
#17507=VECTOR ( 'NONE', #77136, 1000.000000000000000 ) ;
#17508=ORIENTED_EDGE ( 'NONE', *, *, #28836, .F. ) ;
#17514=DIRECTION ( 'NONE',  ( -0.4805540241036398430, -0.8769651246872924855, 0.000000000000000000 ) ) ;
#17516=ORIENTED_EDGE ( 'NONE', *, *, #88072, .T. ) ;
#17528=VERTEX_POINT ( 'NONE', #93882 ) ;
#17535=DIRECTION ( 'NONE',  ( -0.000000000000000000, -0.000000000000000000, -1.000000000000000000 ) ) ;
#17539=CARTESIAN_POINT ( 'NONE',  ( -19.65312891409030271, 93.06504152958497400, 177.5919119679930134 ) ) ;
#17545=AXIS2_PLACEMENT_3D ( 'NONE', #34973, #90230, #36971 ) ;
#17548=VECTOR ( 'NONE', #28512, 1000.000000000000000 ) ;
#17553=EDGE_CURVE ( 'NONE', #18450, #48481, #55802, .T. ) ;
#17557=DIRECTION ( 'NONE',  ( -0.3177184104407523302, 0.9481851146622169990, 0.000000000000000000 ) ) ;
#17563=LINE ( 'NONE', #95114, #83610 ) ;
#17566=EDGE_CURVE ( 'NONE', #61138, #5695, #31028, .T. ) ;
#17567=CARTESIAN_POINT ( 'NONE',  ( 26.37028381016232004, 40.32183835407518302, -10.00000000000000000 ) ) ;
#17584=DIRECTION ( 'NONE',  ( 0.4829524219151267173, -0.8756465943326184886, 0.000000000000000000 ) ) ;
#17605=EDGE_CURVE ( 'NONE', #80767, #91193, #57817, .T. ) ;
#17608=VECTOR ( 'NONE', #94989, 1000.000000000000000 ) ;
#17617=VECTOR ( 'NONE', #39211, 1000.000000000000000 ) ;
#17621=DIRECTION ( 'NONE',  ( -0.000000000000000000, -0.000000000000000000, -1.000000000000000000 ) ) ;
#17634=CIRCLE ( 'NONE', #1442, 70.00000000000001421 ) ;
#17640=ORIENTED_EDGE ( 'NONE', *, *, #1316, .F. ) ;
#17642=ORIENTED_EDGE ( 'NONE', *, *, #5236, .F. ) ;
#17649=DIRECTION ( 'NONE',  ( 0.1172721027424030449, 0.9930998207221544138, 0.000000000000000000 ) ) ;
#17652=VECTOR ( 'NONE', #32429, 1000.000000000000000 ) ;
#17653=ORIENTED_EDGE ( 'NONE', *, *, #60759, .T. ) ;
#17657=CARTESIAN_POINT ( 'NONE',  ( -70.92467617367975663, 45.40763453331954480, -10.00000000000000000 ) ) ;
#17659=FACE_OUTER_BOUND ( 'NONE', #47957, .T. ) ;
#17660=EDGE_LOOP ( 'NONE', ( #28896, #78326, #37607, #9563 ) ) ;
#17665=FACE_OUTER_BOUND ( 'NONE', #48262, .T. ) ;
#17671=CARTESIAN_POINT ( 'NONE',  ( -30.95603806669010538, 23.98360954755322183, 10.00000000000000000 ) ) ;
#17673=ORIENTED_EDGE ( 'NONE', *, *, #90442, .T. ) ;
#17678=ORIENTED_EDGE ( 'NONE', *, *, #76938, .F. ) ;
#17679=ORIENTED_EDGE ( 'NONE', *, *, #96554, .F. ) ;
#17691=EDGE_CURVE ( 'NONE', #28238, #87428, #2700, .T. ) ;
#17692=VECTOR ( 'NONE', #93192, 1000.000000000000000 ) ;
#17698=AXIS2_PLACEMENT_3D ( 'NONE', #83262, #13829, #35131 ) ;
#17711=VECTOR ( 'NONE', #93034, 1000.000000000000000 ) ;
#17715=LINE ( 'NONE', #27310, #6236 ) ;
#17717=CARTESIAN_POINT ( 'NONE',  ( -19.65312891409030271, 93.06504152958497400, 10.00000000000000888 ) ) ;
#17718=VERTEX_POINT ( 'NONE', #31899 ) ;
#17732=EDGE_CURVE ( 'NONE', #76706, #60917, #40496, .T. ) ;
#17738=PLANE ( 'NONE',  #33800 ) ;
#17743=CARTESIAN_POINT ( 'NONE',  ( 12.00096474099108690, 32.03863464977599307, 10.00000000000000000 ) ) ;
#17748=CARTESIAN_POINT ( 'NONE',  ( 38.20673285489099413, 96.19101212341352891, 59.99999999999999289 ) ) ;
#17759=CARTESIAN_POINT ( 'NONE',  ( -13.78482047291978141, 85.09546807867688756, 14.96147123686172620 ) ) ;
#17777=VERTEX_POINT ( 'NONE', #64313 ) ;
#17782=EDGE_LOOP ( 'NONE', ( #11942, #89729, #3600, #93416 ) ) ;
#17786=CARTESIAN_POINT ( 'NONE',  ( -19.65312891409030271, 93.06504152958497400, 177.5919119679930134 ) ) ;
#17789=DIRECTION ( 'NONE',  ( 0.000000000000000000, -0.000000000000000000, -1.000000000000000000 ) ) ;
#17797=VERTEX_POINT ( 'NONE', #82560 ) ;
#17799=ORIENTED_EDGE ( 'NONE', *, *, #70034, .T. ) ;
#17813=CARTESIAN_POINT ( 'NONE',  ( 30.80155721116056355, 46.36891074996812989, 10.00000000000000000 ) ) ;
#17814=VERTEX_POINT ( 'NONE', #37386 ) ;
#17819=ADVANCED_FACE ( 'NONE', ( #99214 ), #13124, .F. ) ;
#17821=CARTESIAN_POINT ( 'NONE',  ( 44.18794977381974576, 118.5901545549086791, 10.00000000000000000 ) ) ;
#17827=ORIENTED_EDGE ( 'NONE', *, *, #33051, .T. ) ;
#17846=DIRECTION ( 'NONE',  ( -0.7082622432767160525, -0.7059494278973771353, 0.000000000000000000 ) ) ;
#17852=LINE ( 'NONE', #33034, #56329 ) ;
#17853=CARTESIAN_POINT ( 'NONE',  ( 6.117390533544194930, 29.33055864014943026, -10.00000000000000000 ) ) ;
#17854=CARTESIAN_POINT ( 'NONE',  ( -23.73952538801239598, 24.43184193311134678, -10.00000000000000000 ) ) ;
#17877=LINE ( 'NONE', #80711, #27461 ) ;
#17878=ORIENTED_EDGE ( 'NONE', *, *, #83156, .T. ) ;
#17902=ORIENTED_EDGE ( 'NONE', *, *, #45812, .F. ) ;
#17923=DIRECTION ( 'NONE',  ( -0.8718556560469457040, -0.4897629171537489778, 0.000000000000000000 ) ) ;
#17928=EDGE_LOOP ( 'NONE', ( #43552, #53171, #76975, #69088 ) ) ;
#17932=DIRECTION ( 'NONE',  ( 0.000000000000000000, 0.000000000000000000, 1.000000000000000000 ) ) ;
#17944=PLANE ( 'NONE',  #38289 ) ;
#17949=ORIENTED_EDGE ( 'NONE', *, *, #50941, .T. ) ;
#17960=ORIENTED_EDGE ( 'NONE', *, *, #54651, .T. ) ;
#17964=EDGE_CURVE ( 'NONE', #61794, #89238, #10792, .T. ) ;
#17976=ORIENTED_EDGE ( 'NONE', *, *, #27551, .F. ) ;
#18002=CARTESIAN_POINT ( 'NONE',  ( -52.15214130626392830, 100.0173953888347569, -10.00000000000000000 ) ) ;
#18008=PLANE ( 'NONE',  #78119 ) ;
#18010=VERTEX_POINT ( 'NONE', #87064 ) ;
#18013=ADVANCED_FACE ( 'NONE', ( #88061 ), #71314, .F. ) ;
#18017=EDGE_LOOP ( 'NONE', ( #58025, #73842, #84091, #20892 ) ) ;
#18030=ORIENTED_EDGE ( 'NONE', *, *, #45339, .T. ) ;
#18032=ADVANCED_FACE ( 'NONE', ( #87577 ), #50856, .F. ) ;
#18042=EDGE_LOOP ( 'NONE', ( #93951, #30610, #89105, #89340 ) ) ;
#18045=ORIENTED_EDGE ( 'NONE', *, *, #86847, .T. ) ;
#18050=VERTEX_POINT ( 'NONE', #74191 ) ;
#18055=FACE_OUTER_BOUND ( 'NONE', #26431, .T. ) ;
#18057=CARTESIAN_POINT ( 'NONE',  ( 48.53010236944518851, 101.9116055364396090, -10.00000000000000000 ) ) ;
#18060=CARTESIAN_POINT ( 'NONE',  ( 42.32809528168264990, 126.1521775423068163, -10.00000000000000000 ) ) ;
#18063=ORIENTED_EDGE ( 'NONE', *, *, #88355, .T. ) ;
#18070=FACE_OUTER_BOUND ( 'NONE', #68635, .T. ) ;
#18075=VERTEX_POINT ( 'NONE', #6253 ) ;
#18078=ORIENTED_EDGE ( 'NONE', *, *, #32798, .T. ) ;
#18079=CARTESIAN_POINT ( 'NONE',  ( -19.65312891409030271, 93.06504152958497400, 59.99999999999999289 ) ) ;
#18080=EDGE_CURVE ( 'NONE', #17465, #42705, #52846, .T. ) ;
#18090=CARTESIAN_POINT ( 'NONE',  ( -19.65312891409030271, 93.06504152958497400, 177.5919119679930134 ) ) ;
#18097=DIRECTION ( 'NONE',  ( -0.000000000000000000, -0.000000000000000000, -1.000000000000000000 ) ) ;
#18102=CARTESIAN_POINT ( 'NONE',  ( 44.35815684012577265, 67.96982248125696913, -10.00000000000000000 ) ) ;
#18105=CARTESIAN_POINT ( 'NONE',  ( -56.14442822474984496, 33.32908021129815523, -10.00000000000000000 ) ) ;
#18111=DIRECTION ( 'NONE',  ( 0.000000000000000000, 0.000000000000000000, -1.000000000000000000 ) ) ;
#18114=PLANE ( 'NONE',  #13620 ) ;
#18115=DIRECTION ( 'NONE',  ( 0.000000000000000000, 0.000000000000000000, 1.000000000000000000 ) ) ;
#18118=DIRECTION ( 'NONE',  ( -0.000000000000000000, 0.000000000000000000, -1.000000000000000000 ) ) ;
#18123=EDGE_LOOP ( 'NONE', ( #74128, #30834, #99, #77737 ) ) ;
#18126=CARTESIAN_POINT ( 'NONE',  ( 32.07315653955450330, 47.77038272570916888, 10.00000000000000000 ) ) ;
#18142=PLANE ( 'NONE',  #14222 ) ;
#18146=DIRECTION ( 'NONE',  ( -1.000000000000000000, 0.000000000000000000, 0.000000000000000000 ) ) ;
#18155=CARTESIAN_POINT ( 'NONE',  ( 5.783292089056025098, 27.85010085989870277, 10.00000000000000000 ) ) ;
#18158=DIRECTION ( 'NONE',  ( 0.4737039832092511671, 0.8806841296921895657, 0.000000000000000000 ) ) ;
#18159=ORIENTED_EDGE ( 'NONE', *, *, #31086, .T. ) ;
#18170=FACE_OUTER_BOUND ( 'NONE', #54256, .T. ) ;
#18175=ORIENTED_EDGE ( 'NONE', *, *, #9958, .T. ) ;
#18187=CARTESIAN_POINT ( 'NONE',  ( 47.84007798744510609, 106.1754093786579318, -10.00000000000000000 ) ) ;
#18190=ORIENTED_EDGE ( 'NONE', *, *, #64591, .T. ) ;
#18196=EDGE_CURVE ( 'NONE', #5695, #15552, #63943, .T. ) ;
#18199=LINE ( 'NONE', #46193, #15574 ) ;
#18200=CARTESIAN_POINT ( 'NONE',  ( 48.32408078245681793, 82.80331927372955647, 10.00000000000000000 ) ) ;
#18202=ORIENTED_EDGE ( 'NONE', *, *, #31534, .F. ) ;
#18210=CARTESIAN_POINT ( 'NONE',  ( -32.04500338604974985, 25.44370296803430520, -10.00000000000000000 ) ) ;
#18224=DIRECTION ( 'NONE',  ( 0.9041295198386993803, -0.4272584830711297910, 0.000000000000000000 ) ) ;
#18227=PLANE ( 'NONE',  #59428 ) ;
#18230=CARTESIAN_POINT ( 'NONE',  ( 28.58622839714300667, 60.96364432824390178, 59.99999999999999289 ) ) ;
#18235=VERTEX_POINT ( 'NONE', #79675 ) ;
#18239=CARTESIAN_POINT ( 'NONE',  ( -50.66096862766640641, 31.69950886434491721, 10.00000000000000000 ) ) ;
#18241=AXIS2_PLACEMENT_3D ( 'NONE', #6264, #98982, #83304 ) ;
#18251=AXIS2_PLACEMENT_3D ( 'NONE', #75093, #53262, #5672 ) ;
#18258=ORIENTED_EDGE ( 'NONE', *, *, #8184, .F. ) ;
#18259=CARTESIAN_POINT ( 'NONE',  ( -17.94336299062649687, 80.50122156528269102, 14.21411446845087845 ) ) ;
#18264=AXIS2_PLACEMENT_3D ( 'NONE', #86394, #93475, #24027 ) ;
#18273=ORIENTED_EDGE ( 'NONE', *, *, #65194, .T. ) ;
#18278=ADVANCED_FACE ( 'NONE', ( #49237 ), #57811, .F. ) ;
#18279=ORIENTED_EDGE ( 'NONE', *, *, #69198, .F. ) ;
#18283=DIRECTION ( 'NONE',  ( -0.9616534368410322164, 0.2742675106749447034, 0.000000000000000000 ) ) ;
#18285=VERTEX_POINT ( 'NONE', #58312 ) ;
#18288=FACE_OUTER_BOUND ( 'NONE', #87604, .T. ) ;
#18298=EDGE_LOOP ( 'NONE', ( #13816, #71034, #56541, #23016 ) ) ;
#18306=FACE_OUTER_BOUND ( 'NONE', #92820, .T. ) ;
#18318=EDGE_CURVE ( 'NONE', #30892, #80971, #66420, .T. ) ;
#18321=AXIS2_PLACEMENT_3D ( 'NONE', #18090, #87045, #77896 ) ;
#18324=CARTESIAN_POINT ( 'NONE',  ( 47.46694519036043403, 73.19305994210745325, -10.00000000000000000 ) ) ;
#18332=AXIS2_PLACEMENT_3D ( 'NONE', #68929, #14249, #23327 ) ;
#18338=VERTEX_POINT ( 'NONE', #46588 ) ;
#18350=CYLINDRICAL_SURFACE ( 'NONE', #32162, 70.00000000000002842 ) ;
#18354=CARTESIAN_POINT ( 'NONE',  ( -19.65312891409030271, 93.06504152958497400, 59.99999999999999289 ) ) ;
#18384=EDGE_CURVE ( 'NONE', #20413, #31364, #17715, .T. ) ;
#18387=PLANE ( 'NONE',  #23432 ) ;
#18407=ORIENTED_EDGE ( 'NONE', *, *, #41038, .F. ) ;
#18409=LINE ( 'NONE', #24490, #48653 ) ;
#18417=CARTESIAN_POINT ( 'NONE',  ( -69.94229046795800286, 43.99946344738946635, -10.00000000000000000 ) ) ;
#18418=VECTOR ( 'NONE', #45737, 1000.000000000000000 ) ;
#18425=EDGE_LOOP ( 'NONE', ( #80775, #67987, #23268, #215 ) ) ;
#18433=ORIENTED_EDGE ( 'NONE', *, *, #97697, .T. ) ;
#18440=DIRECTION ( 'NONE',  ( 0.09547062131715944311, -0.9954322480537364237, 0.000000000000000000 ) ) ;
#18442=ORIENTED_EDGE ( 'NONE', *, *, #40958, .T. ) ;
#18443=CARTESIAN_POINT ( 'NONE',  ( 2.064617007569730767, 27.83817977871671800, -10.00000000000000000 ) ) ;
#18448=CARTESIAN_POINT ( 'NONE',  ( -6.542761065016642341, 25.57183462804972507, -10.00000000000000000 ) ) ;
#18449=ORIENTED_EDGE ( 'NONE', *, *, #98607, .T. ) ;
#18450=VERTEX_POINT ( 'NONE', #12620 ) ;
#18452=DIRECTION ( 'NONE',  ( -1.000000000000000000, 0.000000000000000000, 0.000000000000000000 ) ) ;
#18453=EDGE_CURVE ( 'NONE', #99040, #10180, #51083, .T. ) ;
#18458=ORIENTED_EDGE ( 'NONE', *, *, #91483, .T. ) ;
#18467=ADVANCED_FACE ( 'NONE', ( #29307 ), #5501, .T. ) ;
#18482=ORIENTED_EDGE ( 'NONE', *, *, #42572, .T. ) ;
#18496=ORIENTED_EDGE ( 'NONE', *, *, #50746, .F. ) ;
#18502=PLANE ( 'NONE',  #88090 ) ;
#18506=DIRECTION ( 'NONE',  ( -0.009162850352631533510, 0.9999580202055560196, 0.000000000000000000 ) ) ;
#18513=EDGE_LOOP ( 'NONE', ( #50881, #88884, #79159, #61985 ) ) ;
#18514=PLANE ( 'NONE',  #10137 ) ;
#18516=CARTESIAN_POINT ( 'NONE',  ( -6.542761065016642341, 25.57183462804972862, -10.00000000000000000 ) ) ;
#18524=EDGE_LOOP ( 'NONE', ( #92919, #46439, #31998, #7565 ) ) ;
#18531=EDGE_CURVE ( 'NONE', #23843, #61231, #89176, .T. ) ;
#18535=DIRECTION ( 'NONE',  ( -0.6778389383370750920, -0.7352104281592222179, 0.000000000000000000 ) ) ;
#18547=CIRCLE ( 'NONE', #10440, 70.00000000000001421 ) ;
#18549=DIRECTION ( 'NONE',  ( 0.3666034970181715757, -0.9303772761487930643, 0.000000000000000000 ) ) ;
#18550=DIRECTION ( 'NONE',  ( 0.000000000000000000, 0.000000000000000000, 1.000000000000000000 ) ) ;
#18551=VERTEX_POINT ( 'NONE', #81538 ) ;
#18567=ORIENTED_EDGE ( 'NONE', *, *, #76295, .T. ) ;
#18570=DIRECTION ( 'NONE',  ( -0.000000000000000000, -0.000000000000000000, -1.000000000000000000 ) ) ;
#18573=DIRECTION ( 'NONE',  ( 0.000000000000000000, 0.000000000000000000, 1.000000000000000000 ) ) ;
#18574=LINE ( 'NONE', #67014, #93316 ) ;
#18580=CARTESIAN_POINT ( 'NONE',  ( -19.65312891409030271, 93.06504152958497400, -10.00000000000000888 ) ) ;
#18581=ORIENTED_EDGE ( 'NONE', *, *, #57106, .T. ) ;
#18589=CARTESIAN_POINT ( 'NONE',  ( 21.71530570849275321, 51.45382605859413161, 59.99999999999999289 ) ) ;
#18605=ADVANCED_FACE ( 'NONE', ( #84532 ), #60665, .F. ) ;
#18606=DIRECTION ( 'NONE',  ( 0.000000000000000000, 0.000000000000000000, 1.000000000000000000 ) ) ;
#18610=DIRECTION ( 'NONE',  ( -0.000000000000000000, -0.000000000000000000, 1.000000000000000000 ) ) ;
#18616=AXIS2_PLACEMENT_3D ( 'NONE', #71152, #41211, #72150 ) ;
#18636=LINE ( 'NONE', #40895, #42528 ) ;
#18639=DIRECTION ( 'NONE',  ( -0.09547062131716983757, 0.9954322480537355355, 0.000000000000000000 ) ) ;
#18645=ORIENTED_EDGE ( 'NONE', *, *, #70020, .F. ) ;
#18647=EDGE_LOOP ( 'NONE', ( #1262, #41630, #45607, #27258 ) ) ;
#18659=ORIENTED_EDGE ( 'NONE', *, *, #45660, .T. ) ;
#18660=VECTOR ( 'NONE', #44808, 1000.000000000000114 ) ;
#18663=CARTESIAN_POINT ( 'NONE',  ( 1.813001633210440611, 27.74720351945397923, -10.00000000000000000 ) ) ;
#18665=ORIENTED_EDGE ( 'NONE', *, *, #41239, .T. ) ;
#18675=PLANE ( 'NONE',  #19239 ) ;
#18691=PLANE ( 'NONE',  #2601 ) ;
#18692=EDGE_LOOP ( 'NONE', ( #83355, #20493, #55172, #21889 ) ) ;
#18693=AXIS2_PLACEMENT_3D ( 'NONE', #93533, #23574, #16490 ) ;
#18701=DIRECTION ( 'NONE',  ( -0.9628097264997621529, 0.2701803667135219689, 0.000000000000000000 ) ) ;
#18702=ORIENTED_EDGE ( 'NONE', *, *, #82884, .F. ) ;
#18709=EDGE_CURVE ( 'NONE', #18235, #88859, #71307, .T. ) ;
#18710=CYLINDRICAL_SURFACE ( 'NONE', #74492, 70.00000000000002842 ) ;
#18718=DIRECTION ( 'NONE',  ( 0.000000000000000000, 0.000000000000000000, 1.000000000000000000 ) ) ;
#18722=LINE ( 'NONE', #58684, #12617 ) ;
#18728=AXIS2_PLACEMENT_3D ( 'NONE', #22173, #22680, #53559 ) ;
#18738=CARTESIAN_POINT ( 'NONE',  ( 40.48539884740146277, 126.3902902409112556, -10.00000000000000000 ) ) ;
#18742=DIRECTION ( 'NONE',  ( -0.6855440362341557181, 0.7280311630581363103, 0.000000000000000000 ) ) ;
#18743=VECTOR ( 'NONE', #72174, 1000.000000000000227 ) ;
#18748=EDGE_CURVE ( 'NONE', #36466, #81234, #73793, .T. ) ;
#18774=DIRECTION ( 'NONE',  ( 0.09248003802711829424, -0.9957145386939485476, 0.000000000000000000 ) ) ;
#18779=CARTESIAN_POINT ( 'NONE',  ( 45.56181175559624563, 118.5014625327306135, -10.00000000000000000 ) ) ;
#18786=ORIENTED_EDGE ( 'NONE', *, *, #80555, .T. ) ;
#18793=CARTESIAN_POINT ( 'NONE',  ( -19.65312891409030271, 93.06504152958497400, 10.00000000000000888 ) ) ;
#18794=VECTOR ( 'NONE', #68755, 1000.000000000000000 ) ;
#18798=FACE_BOUND ( 'NONE', #35585, .T. ) ;
#18806=EDGE_LOOP ( 'NONE', ( #4302, #93503, #69008, #60102 ) ) ;
#18813=CARTESIAN_POINT ( 'NONE',  ( -19.65312891409030271, 93.06504152958497400, -10.00000000000000888 ) ) ;
#18816=ADVANCED_FACE ( 'NONE', ( #90533 ), #21103, .T. ) ;
#18818=CARTESIAN_POINT ( 'NONE',  ( -19.74273382965125379, 93.17497195189844206, 59.99999999999999289 ) ) ;
#18826=DIRECTION ( 'NONE',  ( -0.2473641778533917646, -0.9689225787001330970, 0.000000000000000000 ) ) ;
#18830=CIRCLE ( 'NONE', #52707, 0.1418229129681522482 ) ;
#18838=FACE_OUTER_BOUND ( 'NONE', #79974, .T. ) ;
#18842=ADVANCED_FACE ( 'NONE', ( #34775 ), #30167, .T. ) ;
#18859=ORIENTED_EDGE ( 'NONE', *, *, #39874, .F. ) ;
#18863=VECTOR ( 'NONE', #20204, 1000.000000000000000 ) ;
#18867=CARTESIAN_POINT ( 'NONE',  ( -72.30469571560091424, 48.86078274006646183, -10.00000000000000000 ) ) ;
#18877=DIRECTION ( 'NONE',  ( 0.000000000000000000, 0.000000000000000000, 1.000000000000000000 ) ) ;
#18879=EDGE_CURVE ( 'NONE', #16411, #8947, #87321, .T. ) ;
#18883=DIRECTION ( 'NONE',  ( 1.000000000000000000, 0.000000000000000000, 0.000000000000000000 ) ) ;
#18902=VECTOR ( 'NONE', #70627, 1000.000000000000114 ) ;
#18907=LINE ( 'NONE', #80744, #63509 ) ;
#18914=VERTEX_POINT ( 'NONE', #95401 ) ;
#18918=ORIENTED_EDGE ( 'NONE', *, *, #39476, .F. ) ;
#18929=DIRECTION ( 'NONE',  ( 0.000000000000000000, 0.000000000000000000, 1.000000000000000000 ) ) ;
#18934=CARTESIAN_POINT ( 'NONE',  ( 34.81516168915607068, 51.10768172523390973, -10.00000000000000000 ) ) ;
#18937=ORIENTED_EDGE ( 'NONE', *, *, #85972, .T. ) ;
#18946=ORIENTED_EDGE ( 'NONE', *, *, #43385, .T. ) ;
#18949=AXIS2_PLACEMENT_3D ( 'NONE', #1621, #32507, #33506 ) ;
#18952=ORIENTED_EDGE ( 'NONE', *, *, #5997, .T. ) ;
#18953=AXIS2_PLACEMENT_3D ( 'NONE', #40053, #33480, #3114 ) ;
#18958=PLANE ( 'NONE',  #36023 ) ;
#18963=LINE ( 'NONE', #3756, #81807 ) ;
#18964=CIRCLE ( 'NONE', #75557, 70.00000000000001421 ) ;
#18978=ORIENTED_EDGE ( 'NONE', *, *, #66938, .F. ) ;
#19005=ORIENTED_EDGE ( 'NONE', *, *, #68461, .T. ) ;
#19019=EDGE_LOOP ( 'NONE', ( #44398, #59248, #74250, #59499 ) ) ;
#19022=VECTOR ( 'NONE', #30182, 999.9999999999998863 ) ;
#19023=DIRECTION ( 'NONE',  ( -0.3077152132536331575, -0.9514785060800222682, 0.000000000000000000 ) ) ;
#19029=EDGE_CURVE ( 'NONE', #87101, #32335, #67925, .T. ) ;
#19037=ORIENTED_EDGE ( 'NONE', *, *, #67320, .F. ) ;
#19041=ORIENTED_EDGE ( 'NONE', *, *, #38510, .F. ) ;
#19051=AXIS2_PLACEMENT_3D ( 'NONE', #1473, #78991, #9576 ) ;
#19058=ORIENTED_EDGE ( 'NONE', *, *, #98274, .T. ) ;
#19061=ORIENTED_EDGE ( 'NONE', *, *, #42251, .T. ) ;
#19062=CIRCLE ( 'NONE', #43319, 0.1418229129680845801 ) ;
#19068=ADVANCED_FACE ( 'NONE', ( #28417 ), #59297, .F. ) ;
#19069=DIRECTION ( 'NONE',  ( -0.8868092729070087277, -0.4621356007560363244, 0.000000000000000000 ) ) ;
#19075=ORIENTED_EDGE ( 'NONE', *, *, #23167, .T. ) ;
#19089=ORIENTED_EDGE ( 'NONE', *, *, #73337, .F. ) ;
#19090=AXIS2_PLACEMENT_3D ( 'NONE', #92523, #14973, #77807 ) ;
#19092=DIRECTION ( 'NONE',  ( -0.000000000000000000, -0.000000000000000000, -1.000000000000000000 ) ) ;
#19105=CARTESIAN_POINT ( 'NONE',  ( -59.65739779450132829, 37.15562860896454112, -10.00000000000000000 ) ) ;
#19108=AXIS2_PLACEMENT_3D ( 'NONE', #6513, #29803, #36394 ) ;
#19118=VECTOR ( 'NONE', #23978, 1000.000000000000000 ) ;
#19136=CARTESIAN_POINT ( 'NONE',  ( 42.16454434324482747, 125.9067112960471349, -10.00000000000000000 ) ) ;
#19141=DIRECTION ( 'NONE',  ( -0.9292718480896806632, -0.3693965786901518555, 0.000000000000000000 ) ) ;
#19143=ORIENTED_EDGE ( 'NONE', *, *, #62394, .T. ) ;
#19151=LINE ( 'NONE', #17118, #7276 ) ;
#19152=DIRECTION ( 'NONE',  ( -0.8653701635463872943, 0.5011331959107268030, 0.000000000000000000 ) ) ;
#19156=ORIENTED_EDGE ( 'NONE', *, *, #15079, .F. ) ;
#19157=AXIS2_PLACEMENT_3D ( 'NONE', #90802, #9666, #62319 ) ;
#19166=VECTOR ( 'NONE', #19513, 1000.000000000000000 ) ;
#19171=CIRCLE ( 'NONE', #46594, 0.1418229129680828593 ) ;
#19182=VECTOR ( 'NONE', #30493, 1000.000000000000114 ) ;
#19187=DIRECTION ( 'NONE',  ( 0.8495546651763555834, 0.5275005885087621360, 0.000000000000000000 ) ) ;
#19195=FACE_OUTER_BOUND ( 'NONE', #9294, .T. ) ;
#19197=EDGE_LOOP ( 'NONE', ( #29621, #27145, #92956, #16808 ) ) ;
#19199=VERTEX_POINT ( 'NONE', #29921 ) ;
#19204=CARTESIAN_POINT ( 'NONE',  ( -52.66218383418999593, 96.92811335557053098, -10.00000000000000000 ) ) ;
#19206=ORIENTED_EDGE ( 'NONE', *, *, #85123, .F. ) ;
#19207=VECTOR ( 'NONE', #10052, 1000.000000000000000 ) ;
#19208=ORIENTED_EDGE ( 'NONE', *, *, #97598, .F. ) ;
#19209=CARTESIAN_POINT ( 'NONE',  ( 48.95103868752454446, 97.61288834769685252, -10.00000000000000000 ) ) ;
#19210=ORIENTED_EDGE ( 'NONE', *, *, #33379, .T. ) ;
#19217=CARTESIAN_POINT ( 'NONE',  ( -52.70992191624042533, 89.63437584143055403, -10.00000000000000000 ) ) ;
#19224=LINE ( 'NONE', #44470, #57668 ) ;
#19225=EDGE_CURVE ( 'NONE', #10682, #87650, #67417, .T. ) ;
#19227=FACE_OUTER_BOUND ( 'NONE', #9613, .T. ) ;
#19232=EDGE_CURVE ( 'NONE', #87618, #96856, #63056, .T. ) ;
#19236=DIRECTION ( 'NONE',  ( -1.000000000000000000, 0.000000000000000000, 0.000000000000000000 ) ) ;
#19237=EDGE_CURVE ( 'NONE', #11090, #68611, #69419, .T. ) ;
#19239=AXIS2_PLACEMENT_3D ( 'NONE', #86622, #72388, #1479 ) ;
#19253=CARTESIAN_POINT ( 'NONE',  ( 8.569540968619184795, 75.51505761670109962, -10.00000000000000000 ) ) ;
#19254=ORIENTED_EDGE ( 'NONE', *, *, #9448, .T. ) ;
#19270=PLANE ( 'NONE',  #41360 ) ;
#19276=CARTESIAN_POINT ( 'NONE',  ( -17.81655838990255702, 80.92514050927856317, 14.32002587595537690 ) ) ;
#19282=CARTESIAN_POINT ( 'NONE',  ( 1.813001633210440611, 27.74720351945397923, 10.00000000000000000 ) ) ;
#19288=ORIENTED_EDGE ( 'NONE', *, *, #3295, .F. ) ;
#19298=EDGE_CURVE ( 'NONE', #26627, #22737, #19418, .T. ) ;
#19299=ORIENTED_EDGE ( 'NONE', *, *, #69056, .T. ) ;
#19300=ORIENTED_EDGE ( 'NONE', *, *, #81415, .T. ) ;
#19302=LINE ( 'NONE', #50169, #20072 ) ;
#19310=EDGE_CURVE ( 'NONE', #42311, #2950, #1023, .T. ) ;
#19313=AXIS2_PLACEMENT_3D ( 'NONE', #56588, #40870, #95654 ) ;
#19316=VECTOR ( 'NONE', #96987, 1000.000000000000000 ) ;
#19330=FACE_OUTER_BOUND ( 'NONE', #71415, .T. ) ;
#19331=DIRECTION ( 'NONE',  ( -0.7511915808658203852, -0.6600842437418951159, 0.000000000000000000 ) ) ;
#19333=ORIENTED_EDGE ( 'NONE', *, *, #9088, .F. ) ;
#19339=AXIS2_PLACEMENT_3D ( 'NONE', #24960, #7262, #99991 ) ;
#19343=ORIENTED_EDGE ( 'NONE', *, *, #14894, .F. ) ;
#19346=VERTEX_POINT ( 'NONE', #46097 ) ;
#19348=DIRECTION ( 'NONE',  ( 1.000000000000000000, 0.000000000000000000, 0.000000000000000000 ) ) ;
#19349=EDGE_CURVE ( 'NONE', #44888, #90330, #38504, .T. ) ;
#19356=CARTESIAN_POINT ( 'NONE',  ( -19.72534873751503781, 92.94298401958562295, 59.99999999999999289 ) ) ;
#19357=DIRECTION ( 'NONE',  ( 0.000000000000000000, 0.000000000000000000, 1.000000000000000000 ) ) ;
#19359=DIRECTION ( 'NONE',  ( -0.6681572590663519273, 0.7440200784635719877, 0.000000000000000000 ) ) ;
#19361=PLANE ( 'NONE',  #90270 ) ;
#19363=EDGE_CURVE ( 'NONE', #87907, #29268, #40406, .T. ) ;
#19368=DIRECTION ( 'NONE',  ( 0.000000000000000000, 0.000000000000000000, 1.000000000000000000 ) ) ;
#19375=AXIS2_PLACEMENT_3D ( 'NONE', #35685, #82342, #12910 ) ;
#19392=DIRECTION ( 'NONE',  ( -0.000000000000000000, -0.000000000000000000, -1.000000000000000000 ) ) ;
#19404=LINE ( 'NONE', #48789, #36811 ) ;
#19405=DIRECTION ( 'NONE',  ( -0.1889875038809575303, -0.9819794923402652698, 0.000000000000000000 ) ) ;
#19410=VECTOR ( 'NONE', #13046, 1000.000000000000000 ) ;
#19412=EDGE_CURVE ( 'NONE', #17718, #10180, #76032, .T. ) ;
#19418=CIRCLE ( 'NONE', #80913, 70.00000000000001421 ) ;
#19425=ORIENTED_EDGE ( 'NONE', *, *, #13674, .T. ) ;
#19426=EDGE_LOOP ( 'NONE', ( #31467, #52292, #78455, #10945 ) ) ;
#19433=EDGE_LOOP ( 'NONE', ( #45664, #943, #35326, #12163 ) ) ;
#19434=EDGE_CURVE ( 'NONE', #52564, #97421, #53356, .T. ) ;
#19439=CARTESIAN_POINT ( 'NONE',  ( 46.99867368304095550, 76.19044720721625197, 10.00000000000000000 ) ) ;
#19444=VERTEX_POINT ( 'NONE', #71434 ) ;
#19448=CARTESIAN_POINT ( 'NONE',  ( -64.74139798177010618, 41.16849083240310847, 10.00000000000000000 ) ) ;
#19449=ORIENTED_EDGE ( 'NONE', *, *, #2779, .F. ) ;
#19454=PLANE ( 'NONE',  #57608 ) ;
#19455=DIRECTION ( 'NONE',  ( -0.04056776950002415755, 0.9991767892008865948, 0.000000000000000000 ) ) ;
#19456=VECTOR ( 'NONE', #2361, 1000.000000000000000 ) ;
#19463=LINE ( 'NONE', #37106, #51522 ) ;
#19465=VERTEX_POINT ( 'NONE', #22819 ) ;
#19468=EDGE_CURVE ( 'NONE', #57311, #45676, #32909, .T. ) ;
#19471=DIRECTION ( 'NONE',  ( 0.000000000000000000, 0.000000000000000000, 1.000000000000000000 ) ) ;
#19474=AXIS2_PLACEMENT_3D ( 'NONE', #69901, #23800, #70407 ) ;
#19475=EDGE_LOOP ( 'NONE', ( #85063, #75899, #15887, #69758 ) ) ;
#19477=EDGE_CURVE ( 'NONE', #12886, #63646, #73922, .T. ) ;
#19484=DIRECTION ( 'NONE',  ( 0.000000000000000000, 0.000000000000000000, 1.000000000000000000 ) ) ;
#19492=ADVANCED_FACE ( 'NONE', ( #4015 ), #34415, .T. ) ;
#19498=PLANE ( 'NONE',  #94851 ) ;
#19510=CARTESIAN_POINT ( 'NONE',  ( 29.12701137275935892, 44.61184105132205957, -10.00000000000000000 ) ) ;
#19513=DIRECTION ( 'NONE',  ( -0.000000000000000000, 0.000000000000000000, -1.000000000000000000 ) ) ;
#19521=LINE ( 'NONE', #56973, #46779 ) ;
#19524=CARTESIAN_POINT ( 'NONE',  ( 48.61286661847091040, 84.94359857078811160, -10.00000000000000000 ) ) ;
#19538=AXIS2_PLACEMENT_3D ( 'NONE', #1517, #56179, #87173 ) ;
#19548=EDGE_CURVE ( 'NONE', #76128, #61758, #93838, .T. ) ;
#19549=CARTESIAN_POINT ( 'NONE',  ( 32.86530875704925592, 117.5470576720593954, 59.99999999999999289 ) ) ;
#19551=PLANE ( 'NONE',  #22097 ) ;
#19557=ORIENTED_EDGE ( 'NONE', *, *, #25246, .F. ) ;
#19561=ADVANCED_FACE ( 'NONE', ( #5021 ), #82060, .F. ) ;
#19564=VERTEX_POINT ( 'NONE', #6006 ) ;
#19565=DIRECTION ( 'NONE',  ( -0.6118251767726359258, -0.7909930170786165782, 0.000000000000000000 ) ) ;
#19589=EDGE_LOOP ( 'NONE', ( #7530, #32174, #48828, #98998 ) ) ;
#19595=ADVANCED_FACE ( 'NONE', ( #51610 ), #21221, .F. ) ;
#19610=DIRECTION ( 'NONE',  ( -0.9879428538673719062, -0.1548189829846212673, 0.000000000000000000 ) ) ;
#19614=DIRECTION ( 'NONE',  ( -0.000000000000000000, -0.000000000000000000, -1.000000000000000000 ) ) ;
#19640=ORIENTED_EDGE ( 'NONE', *, *, #89508, .F. ) ;
#19645=ORIENTED_EDGE ( 'NONE', *, *, #47301, .F. ) ;
#19660=EDGE_CURVE ( 'NONE', #60043, #45522, #47852, .T. ) ;
#19665=CARTESIAN_POINT ( 'NONE',  ( -4.731736819106164837, 24.67387208536690224, 10.00000000000000000 ) ) ;
#19667=DIRECTION ( 'NONE',  ( 0.000000000000000000, 0.000000000000000000, 1.000000000000000000 ) ) ;
#19690=ORIENTED_EDGE ( 'NONE', *, *, #83453, .T. ) ;
#19693=CARTESIAN_POINT ( 'NONE',  ( -49.40214497367342972, 107.8811501326408546, -10.00000000000000000 ) ) ;
#19700=EDGE_CURVE ( 'NONE', #71493, #65030, #2418, .T. ) ;
#19705=CARTESIAN_POINT ( 'NONE',  ( -43.67044039880972406, 70.09354223814025886, -10.00000000000000000 ) ) ;
#19709=DIRECTION ( 'NONE',  ( 0.2701803667135219689, 0.9628097264997621529, 0.000000000000000000 ) ) ;
#19716=DIRECTION ( 'NONE',  ( 0.000000000000000000, 0.000000000000000000, 1.000000000000000000 ) ) ;
#19717=CARTESIAN_POINT ( 'NONE',  ( 49.42830306794132866, 81.76213237698443947, -10.00000000000000000 ) ) ;
#19723=CARTESIAN_POINT ( 'NONE',  ( -40.14225747417106760, 26.13077817479420872, 177.5919119679930134 ) ) ;
#19725=LINE ( 'NONE', #3528, #91594 ) ;
#19733=DIRECTION ( 'NONE',  ( -0.6384778167143362326, 0.7696402260561061581, 0.000000000000000000 ) ) ;
#19738=LINE ( 'NONE', #61067, #66290 ) ;
#19741=DIRECTION ( 'NONE',  ( -0.9515606131578174809, -0.3074612162317687525, 0.000000000000000000 ) ) ;
#19749=CARTESIAN_POINT ( 'NONE',  ( 46.22371820283662203, 112.7232458147606451, -10.00000000000000000 ) ) ;
#19752=DIRECTION ( 'NONE',  ( 0.000000000000000000, 0.000000000000000000, 1.000000000000000000 ) ) ;
#19753=DIRECTION ( 'NONE',  ( 0.2471055264905481497, -0.9689885751534065284, 0.000000000000000000 ) ) ;
#19761=CARTESIAN_POINT ( 'NONE',  ( -10.95801343888480339, 85.52545552628633629, 14.52632409138724512 ) ) ;
#19773=VERTEX_POINT ( 'NONE', #98618 ) ;
#19777=FACE_OUTER_BOUND ( 'NONE', #99183, .T. ) ;
#19789=EDGE_CURVE ( 'NONE', #28368, #62719, #83426, .T. ) ;
#19794=ADVANCED_FACE ( 'NONE', ( #44871 ), #12510, .F. ) ;
#19802=FACE_BOUND ( 'NONE', #2842, .T. ) ;
#19803=CARTESIAN_POINT ( 'NONE',  ( -72.48190909937208914, 49.06123820388767598, 10.00000000000000000 ) ) ;
#19805=DIRECTION ( 'NONE',  ( -0.9963824715083250405, 0.08498217737244646852, 0.000000000000000000 ) ) ;
#19811=CARTESIAN_POINT ( 'NONE',  ( -35.89898968889472997, 24.97633462685643124, -10.00000000000000000 ) ) ;
#19813=EDGE_LOOP ( 'NONE', ( #9298, #93431, #40820, #18946 ) ) ;
#19818=DIRECTION ( 'NONE',  ( -0.000000000000000000, 0.000000000000000000, -1.000000000000000000 ) ) ;
#19819=DIRECTION ( 'NONE',  ( -0.2877784213863714968, 0.9576970189910627429, 0.000000000000000000 ) ) ;
#19830=CARTESIAN_POINT ( 'NONE',  ( -61.61048871844075592, 38.59675092633816007, -10.00000000000000000 ) ) ;
#19831=EDGE_LOOP ( 'NONE', ( #60997, #94246, #3259, #953 ) ) ;
#19834=DIRECTION ( 'NONE',  ( -0.5888918169447047157, 0.8082118706970125022, 0.000000000000000000 ) ) ;
#19842=EDGE_CURVE ( 'NONE', #99166, #99285, #85288, .T. ) ;
#19843=VECTOR ( 'NONE', #81592, 1000.000000000000000 ) ;
#19857=CIRCLE ( 'NONE', #76480, 70.00000000000001421 ) ;
#19869=LINE ( 'NONE', #81201, #83367 ) ;
#19872=DIRECTION ( 'NONE',  ( -0.9994626398093611197, -0.03277852384265240310, 0.000000000000000000 ) ) ;
#19884=CARTESIAN_POINT ( 'NONE',  ( -58.02784037451009880, 34.21088073648085981, 10.00000000000000000 ) ) ;
#19886=DIRECTION ( 'NONE',  ( -1.000000000000000000, 0.000000000000000000, 0.000000000000000000 ) ) ;
#19897=ORIENTED_EDGE ( 'NONE', *, *, #43172, .T. ) ;
#19904=DIRECTION ( 'NONE',  ( -1.000000000000000000, 0.000000000000000000, 0.000000000000000000 ) ) ;
#19910=ORIENTED_EDGE ( 'NONE', *, *, #24676, .T. ) ;
#19912=EDGE_CURVE ( 'NONE', #37567, #56511, #89550, .T. ) ;
#19916=ORIENTED_EDGE ( 'NONE', *, *, #8510, .T. ) ;
#19919=DIRECTION ( 'NONE',  ( 0.000000000000000000, 0.000000000000000000, 1.000000000000000000 ) ) ;
#19923=AXIS2_PLACEMENT_3D ( 'NONE', #64467, #23953, #32568 ) ;
#19926=ORIENTED_EDGE ( 'NONE', *, *, #29524, .T. ) ;
#19927=FACE_OUTER_BOUND ( 'NONE', #72898, .T. ) ;
#19932=FACE_OUTER_BOUND ( 'NONE', #9355, .T. ) ;
#19936=VECTOR ( 'NONE', #76688, 1000.000000000000000 ) ;
#19937=ORIENTED_EDGE ( 'NONE', *, *, #48568, .F. ) ;
#19942=ORIENTED_EDGE ( 'NONE', *, *, #65876, .F. ) ;
#19961=EDGE_CURVE ( 'NONE', #11356, #1030, #20606, .T. ) ;
#19975=ORIENTED_EDGE ( 'NONE', *, *, #78320, .F. ) ;
#19986=FACE_OUTER_BOUND ( 'NONE', #81169, .T. ) ;
#19993=VECTOR ( 'NONE', #48402, 1000.000000000000000 ) ;
#20000=LINE ( 'NONE', #53369, #83000 ) ;
#20002=ORIENTED_EDGE ( 'NONE', *, *, #30122, .F. ) ;
#20005=CARTESIAN_POINT ( 'NONE',  ( -19.65312891409030271, 93.06504152958497400, -10.00000000000000000 ) ) ;
#20017=DIRECTION ( 'NONE',  ( -0.7893155279419928894, -0.6139877827364751406, 0.000000000000000000 ) ) ;
#20029=EDGE_LOOP ( 'NONE', ( #70379, #39291, #92892, #27288 ) ) ;
#20038=CARTESIAN_POINT ( 'NONE',  ( 41.51553799054923388, 59.02985107750645000, 177.5919119679930134 ) ) ;
#20040=EDGE_CURVE ( 'NONE', #86862, #11831, #67561, .T. ) ;
#20048=LINE ( 'NONE', #50920, #99402 ) ;
#20050=ORIENTED_EDGE ( 'NONE', *, *, #96381, .T. ) ;
#20051=DIRECTION ( 'NONE',  ( -0.9956898167541090583, 0.09274582908232931189, 0.000000000000000000 ) ) ;
#20054=DIRECTION ( 'NONE',  ( -0.9942962326340534229, -0.1066536533351210708, 0.000000000000000000 ) ) ;
#20062=VERTEX_POINT ( 'NONE', #35671 ) ;
#20063=CARTESIAN_POINT ( 'NONE',  ( -34.16292631813981728, 25.86630820016799248, -10.00000000000000000 ) ) ;
#20071=DIRECTION ( 'NONE',  ( -1.000000000000000000, 0.000000000000000000, 0.000000000000000000 ) ) ;
#20072=VECTOR ( 'NONE', #42548, 1000.000000000000000 ) ;
#20075=ORIENTED_EDGE ( 'NONE', *, *, #28774, .T. ) ;
#20078=AXIS2_PLACEMENT_3D ( 'NONE', #65197, #72325, #34298 ) ;
#20081=AXIS2_PLACEMENT_3D ( 'NONE', #15006, #76345, #61106 ) ;
#20082=DIRECTION ( 'NONE',  ( 0.9755587037855241173, -0.2197389712097240766, 0.000000000000000000 ) ) ;
#20088=ADVANCED_FACE ( 'NONE', ( #19986 ), #59443, .F. ) ;
#20092=ORIENTED_EDGE ( 'NONE', *, *, #8174, .F. ) ;
#20093=FACE_OUTER_BOUND ( 'NONE', #34608, .T. ) ;
#20099=CARTESIAN_POINT ( 'NONE',  ( 22.72264919896475988, 37.02287747747012503, -10.00000000000000000 ) ) ;
#20108=DIRECTION ( 'NONE',  ( 1.000000000000000000, 0.000000000000000000, 0.000000000000000000 ) ) ;
#20112=DIRECTION ( 'NONE',  ( -0.001635407438350354676, -0.9999986627203610867, 0.000000000000000000 ) ) ;
#20115=DIRECTION ( 'NONE',  ( 0.000000000000000000, 0.000000000000000000, 1.000000000000000000 ) ) ;
#20122=FACE_OUTER_BOUND ( 'NONE', #78708, .T. ) ;
#20126=ORIENTED_EDGE ( 'NONE', *, *, #34864, .T. ) ;
#20128=LINE ( 'NONE', #42884, #16707 ) ;
#20131=ADVANCED_FACE ( 'NONE', ( #16359 ), #38135, .F. ) ;
#20140=EDGE_CURVE ( 'NONE', #74959, #31723, #15339, .T. ) ;
#20158=EDGE_CURVE ( 'NONE', #54381, #24764, #63953, .T. ) ;
#20163=ORIENTED_EDGE ( 'NONE', *, *, #55878, .T. ) ;
#20178=LINE ( 'NONE', #64265, #38211 ) ;
#20181=ORIENTED_EDGE ( 'NONE', *, *, #40293, .T. ) ;
#20188=VERTEX_POINT ( 'NONE', #64462 ) ;
#20191=DIRECTION ( 'NONE',  ( 0.000000000000000000, 0.000000000000000000, 1.000000000000000000 ) ) ;
#20198=CARTESIAN_POINT ( 'NONE',  ( 33.63407072503001416, 49.62913085183823370, 10.00000000000000000 ) ) ;
#20204=DIRECTION ( 'NONE',  ( 0.000000000000000000, 0.000000000000000000, 1.000000000000000000 ) ) ;
#20222=DIRECTION ( 'NONE',  ( -0.9302793824855987159, 0.3668518372888613377, 0.000000000000000000 ) ) ;
#20225=DIRECTION ( 'NONE',  ( -0.4272584830711297910, -0.9041295198386993803, 0.000000000000000000 ) ) ;
#20231=CARTESIAN_POINT ( 'NONE',  ( -19.54038299334472484, 93.15107696413387828, 59.99999999999999289 ) ) ;
#20248=ADVANCED_FACE ( 'NONE', ( #58342 ), #29328, .F. ) ;
#20252=VERTEX_POINT ( 'NONE', #60194 ) ;
#20254=DIRECTION ( 'NONE',  ( -0.2197389712097240488, -0.9755587037855242283, 0.000000000000000000 ) ) ;
#20259=EDGE_CURVE ( 'NONE', #11090, #23644, #37897, .T. ) ;
#20260=CARTESIAN_POINT ( 'NONE',  ( 32.23239235789582580, 67.26876094202697232, 59.99999999999999289 ) ) ;
#20263=DIRECTION ( 'NONE',  ( -0.8917477921037054722, -0.4525327339300069251, 0.000000000000000000 ) ) ;
#20265=VERTEX_POINT ( 'NONE', #74069 ) ;
#20267=FACE_OUTER_BOUND ( 'NONE', #42225, .T. ) ;
#20269=CARTESIAN_POINT ( 'NONE',  ( -19.65312891409030271, 93.06504152958497400, 59.99999999999999289 ) ) ;
#20270=ADVANCED_FACE ( 'NONE', ( #68805 ), #91154, .F. ) ;
#20271=ORIENTED_EDGE ( 'NONE', *, *, #85808, .F. ) ;
#20275=CIRCLE ( 'NONE', #8902, 0.1418229129683812317 ) ;
#20290=ORIENTED_EDGE ( 'NONE', *, *, #30736, .F. ) ;
#20291=EDGE_LOOP ( 'NONE', ( #64518, #63078, #31375, #43416 ) ) ;
#20292=FACE_BOUND ( 'NONE', #67722, .T. ) ;
#20295=ORIENTED_EDGE ( 'NONE', *, *, #52129, .T. ) ;
#20296=DIRECTION ( 'NONE',  ( 0.08498217737244646852, 0.9963824715083250405, 0.000000000000000000 ) ) ;
#20300=VERTEX_POINT ( 'NONE', #68310 ) ;
#20308=DIRECTION ( 'NONE',  ( -0.000000000000000000, -0.000000000000000000, -1.000000000000000000 ) ) ;
#20311=DIRECTION ( 'NONE',  ( -1.000000000000000000, 0.000000000000000000, 0.000000000000000000 ) ) ;
#20314=CIRCLE ( 'NONE', #52599, 0.1418229129681522482 ) ;
#20320=ORIENTED_EDGE ( 'NONE', *, *, #64941, .F. ) ;
#20323=CARTESIAN_POINT ( 'NONE',  ( 30.49745206674571563, 75.84738672984741470, 59.99999999999999289 ) ) ;
#20325=VECTOR ( 'NONE', #37852, 1000.000000000000114 ) ;
#20328=CARTESIAN_POINT ( 'NONE',  ( -12.68721568607400485, 24.67147432707382748, 10.00000000000000000 ) ) ;
#20332=CARTESIAN_POINT ( 'NONE',  ( 26.18314342202569023, 41.82794442100486521, -10.00000000000000000 ) ) ;
#20333=CARTESIAN_POINT ( 'NONE',  ( 48.58805178314243278, 84.67719436603331928, -10.00000000000000000 ) ) ;
#20351=PRODUCT_DEFINITION_FORMATION_WITH_SPECIFIED_SOURCE ( 'ANY', '', #65334, .NOT_KNOWN. ) ;
#20352=FACE_OUTER_BOUND ( 'NONE', #38170, .T. ) ;
#20375=DIRECTION ( 'NONE',  ( 0.3371987438498061929, -0.9414334852479556703, 0.000000000000000000 ) ) ;
#20385=VECTOR ( 'NONE', #91129, 1000.000000000000114 ) ;
#20386=CARTESIAN_POINT ( 'NONE',  ( 46.88368875251780565, 110.3874725885333135, -10.00000000000000000 ) ) ;
#20387=ORIENTED_EDGE ( 'NONE', *, *, #989, .F. ) ;
#20392=CARTESIAN_POINT ( 'NONE',  ( 42.55442611339157111, 60.96799964870729127, 177.5919119679930134 ) ) ;
#20396=AXIS2_PLACEMENT_3D ( 'NONE', #36719, #60013, #4338 ) ;
#20399=ORIENTED_EDGE ( 'NONE', *, *, #77995, .T. ) ;
#20409=LINE ( 'NONE', #82742, #44269 ) ;
#20413=VERTEX_POINT ( 'NONE', #56153 ) ;
#20420=EDGE_LOOP ( 'NONE', ( #74488, #2543, #38087, #32961 ) ) ;
#20422=AXIS2_PLACEMENT_3D ( 'NONE', #73545, #11264, #12247 ) ;
#20439=LINE ( 'NONE', #48964, #57965 ) ;
#20448=EDGE_LOOP ( 'NONE', ( #46011, #62241, #71129, #64012 ) ) ;
#20455=CARTESIAN_POINT ( 'NONE',  ( -1.087500518889665591, 25.57194971796827332, -10.00000000000000000 ) ) ;
#20460=LINE ( 'NONE', #44717, #77002 ) ;
#20462=VERTEX_POINT ( 'NONE', #39947 ) ;
#20467=AXIS2_PLACEMENT_3D ( 'NONE', #14450, #44831, #75764 ) ;
#20471=EDGE_CURVE ( 'NONE', #98305, #28495, #72106, .T. ) ;
#20473=CARTESIAN_POINT ( 'NONE',  ( 45.86253193465722688, 68.41350641406140198, 10.00000000000000000 ) ) ;
#20475=ORIENTED_EDGE ( 'NONE', *, *, #63363, .F. ) ;
#20483=VECTOR ( 'NONE', #15159, 1000.000000000000114 ) ;
#20490=CARTESIAN_POINT ( 'NONE',  ( -32.30932376655839988, 25.48519649537502119, 10.00000000000000000 ) ) ;
#20493=ORIENTED_EDGE ( 'NONE', *, *, #7079, .F. ) ;
#20494=AXIS2_PLACEMENT_3D ( 'NONE', #68580, #99505, #55361 ) ;
#20496=CARTESIAN_POINT ( 'NONE',  ( 46.74097198175142154, 116.0488203434314727, 10.00000000000000000 ) ) ;
#20504=ORIENTED_EDGE ( 'NONE', *, *, #1513, .F. ) ;
#20507=CARTESIAN_POINT ( 'NONE',  ( -10.54235908185773418, 24.92402704602492847, 10.00000000000000000 ) ) ;
#20525=DIRECTION ( 'NONE',  ( 0.3374500364938339270, 0.9413434404457866611, 0.000000000000000000 ) ) ;
#20526=ORIENTED_EDGE ( 'NONE', *, *, #64042, .T. ) ;
#20530=AXIS2_PLACEMENT_3D ( 'NONE', #63399, #64401, #17294 ) ;
#20532=CARTESIAN_POINT ( 'NONE',  ( -19.65312891409030271, 93.06504152958497400, 10.00000000000000888 ) ) ;
#20533=ORIENTED_EDGE ( 'NONE', *, *, #71364, .T. ) ;
#20536=AXIS2_PLACEMENT_3D ( 'NONE', #75993, #36454, #6570 ) ;
#20539=ORIENTED_EDGE ( 'NONE', *, *, #76944, .T. ) ;
#20541=AXIS2_PLACEMENT_3D ( 'NONE', #72146, #26042, #87899 ) ;
#20542=VERTEX_POINT ( 'NONE', #24767 ) ;
#20545=ADVANCED_FACE ( 'NONE', ( #47564 ), #63773, .F. ) ;
#20547=CYLINDRICAL_SURFACE ( 'NONE', #96304, 70.00000000000002842 ) ;
#20551=LINE ( 'NONE', #29630, #47911 ) ;
#20585=DIRECTION ( 'NONE',  ( -0.000000000000000000, 0.000000000000000000, 1.000000000000000000 ) ) ;
#20587=ADVANCED_FACE ( 'NONE', ( #78492 ), #8581, .T. ) ;
#20597=EDGE_CURVE ( 'NONE', #49571, #16524, #1981, .T. ) ;
#20598=VECTOR ( 'NONE', #76783, 1000.000000000000000 ) ;
#20600=VECTOR ( 'NONE', #67429, 1000.000000000000000 ) ;
#20606=LINE ( 'NONE', #51993, #10859 ) ;
#20614=LINE ( 'NONE', #84433, #59508 ) ;
#20626=DIRECTION ( 'NONE',  ( 0.2194785493951409983, -0.9756173257765590190, 0.000000000000000000 ) ) ;
#20627=VERTEX_POINT ( 'NONE', #31366 ) ;
#20632=LINE ( 'NONE', #5427, #51713 ) ;
#20641=ORIENTED_EDGE ( 'NONE', *, *, #32982, .T. ) ;
#20642=DIRECTION ( 'NONE',  ( -1.000000000000000000, -4.892646582057456999E-14, 0.000000000000000000 ) ) ;
#20643=ORIENTED_EDGE ( 'NONE', *, *, #45660, .F. ) ;
#20651=ADVANCED_FACE ( 'NONE', ( #79007 ), #73755, .F. ) ;
#20656=CARTESIAN_POINT ( 'NONE',  ( 34.81516168915606357, 51.10768172523390973, -10.00000000000000000 ) ) ;
#20660=CARTESIAN_POINT ( 'NONE',  ( 48.92549481379852949, 97.87922363803308201, -10.00000000000000000 ) ) ;
#20664=EDGE_CURVE ( 'NONE', #35809, #73457, #28140, .T. ) ;
#20673=ORIENTED_EDGE ( 'NONE', *, *, #98080, .F. ) ;
#20687=AXIS2_PLACEMENT_3D ( 'NONE', #16383, #24483, #31073 ) ;
#20694=ORIENTED_EDGE ( 'NONE', *, *, #76938, .T. ) ;
#20695=VECTOR ( 'NONE', #40812, 1000.000000000000000 ) ;
#20698=EDGE_CURVE ( 'NONE', #33736, #56406, #13460, .T. ) ;
#20708=VECTOR ( 'NONE', #75319, 1000.000000000000000 ) ;
#20713=LINE ( 'NONE', #12621, #46257 ) ;
#20718=ADVANCED_FACE ( 'NONE', ( #92466 ), #23013, .F. ) ;
#20725=DIRECTION ( 'NONE',  ( -0.7893155279419930004, -0.6139877827364750296, 0.000000000000000000 ) ) ;
#20733=CARTESIAN_POINT ( 'NONE',  ( -4.653128914090325807, 78.77562236714182120, 52.49999999999999289 ) ) ;
#20736=AXIS2_PLACEMENT_3D ( 'NONE', #43849, #59031, #43350 ) ;
#20743=VECTOR ( 'NONE', #69107, 1000.000000000000000 ) ;
#20748=DIRECTION ( 'NONE',  ( 0.000000000000000000, 0.000000000000000000, -1.000000000000000000 ) ) ;
#20749=VECTOR ( 'NONE', #67061, 1000.000000000000114 ) ;
#20752=DIRECTION ( 'NONE',  ( -0.2803049773603352723, 0.9599109957006545235, 0.000000000000000000 ) ) ;
#20754=VERTEX_POINT ( 'NONE', #93969 ) ;
#20758=DIRECTION ( 'NONE',  ( 0.9755587037855241173, -0.2197389712097240211, 0.000000000000000000 ) ) ;
#20761=VECTOR ( 'NONE', #85224, 1000.000000000000000 ) ;
#20762=LINE ( 'NONE', #84092, #86411 ) ;
#20773=CARTESIAN_POINT ( 'NONE',  ( 15.54467260552930341, 34.00295985972733348, 10.00000000000000000 ) ) ;
#20783=ORIENTED_EDGE ( 'NONE', *, *, #27888, .F. ) ;
#20790=ORIENTED_EDGE ( 'NONE', *, *, #78516, .T. ) ;
#20794=ORIENTED_EDGE ( 'NONE', *, *, #54147, .T. ) ;
#20799=CARTESIAN_POINT ( 'NONE',  ( 0.4022032943177059061, 45.37891224861880346, 59.99999999999999289 ) ) ;
#20808=LINE ( 'NONE', #354, #75513 ) ;
#20812=AXIS2_PLACEMENT_3D ( 'NONE', #76993, #98833, #45103 ) ;
#20813=ORIENTED_EDGE ( 'NONE', *, *, #22839, .T. ) ;
#20820=LINE ( 'NONE', #45090, #37961 ) ;
#20822=CARTESIAN_POINT ( 'NONE',  ( 46.80963145949299076, 71.09457308843315104, 177.5919119679930134 ) ) ;
#20823=AXIS2_PLACEMENT_3D ( 'NONE', #93938, #32081, #71114 ) ;
#20825=ORIENTED_EDGE ( 'NONE', *, *, #28811, .F. ) ;
#20830=DIRECTION ( 'NONE',  ( 1.000000000000000000, 0.000000000000000000, 0.000000000000000000 ) ) ;
#20831=CYLINDRICAL_SURFACE ( 'NONE', #79359, 70.00000000000002842 ) ;
#20834=CIRCLE ( 'NONE', #54785, 70.00000000000001421 ) ;
#20842=EDGE_CURVE ( 'NONE', #66829, #67877, #51827, .T. ) ;
#20873=DIRECTION ( 'NONE',  ( 0.1783728972749306640, 0.9839629614562466209, 0.000000000000000000 ) ) ;
#20877=EDGE_CURVE ( 'NONE', #81790, #81845, #36602, .T. ) ;
#20881=VECTOR ( 'NONE', #30683, 1000.000000000000000 ) ;
#20892=ORIENTED_EDGE ( 'NONE', *, *, #90616, .T. ) ;
#20893=VECTOR ( 'NONE', #79537, 1000.000000000000000 ) ;
#20894=CARTESIAN_POINT ( 'NONE',  ( 47.92671612011951510, 80.40884667711614497, -10.00000000000000000 ) ) ;
#20897=DIRECTION ( 'NONE',  ( -0.7510153523339186954, 0.6602847420308604054, 0.000000000000000000 ) ) ;
#20898=ORIENTED_EDGE ( 'NONE', *, *, #21888, .F. ) ;
#20904=ORIENTED_EDGE ( 'NONE', *, *, #98009, .F. ) ;
#20907=VERTEX_POINT ( 'NONE', #98934 ) ;
#20917=EDGE_CURVE ( 'NONE', #65735, #81256, #50319, .T. ) ;
#20928=ORIENTED_EDGE ( 'NONE', *, *, #70020, .T. ) ;
#20929=EDGE_CURVE ( 'NONE', #15783, #54743, #89385, .T. ) ;
#20933=EDGE_CURVE ( 'NONE', #72951, #45184, #37591, .T. ) ;
#20934=ORIENTED_EDGE ( 'NONE', *, *, #56716, .F. ) ;
#20948=DIRECTION ( 'NONE',  ( 0.2774202615135334948, -0.9607486656258038549, 0.000000000000000000 ) ) ;
#20958=ORIENTED_EDGE ( 'NONE', *, *, #73971, .T. ) ;
#20961=EDGE_CURVE ( 'NONE', #62875, #44322, #99922, .T. ) ;
#20965=DIRECTION ( 'NONE',  ( -0.000000000000000000, -0.000000000000000000, -1.000000000000000000 ) ) ;
#20971=CARTESIAN_POINT ( 'NONE',  ( -18.15312891409030627, 78.77562236714182120, 13.81405534229504894 ) ) ;
#20972=CIRCLE ( 'NONE', #54920, 70.00000000000001421 ) ;
#20973=VERTEX_POINT ( 'NONE', #92839 ) ;
#20979=VECTOR ( 'NONE', #2905, 1000.000000000000000 ) ;
#20984=ORIENTED_EDGE ( 'NONE', *, *, #52362, .T. ) ;
#20989=AXIS2_PLACEMENT_3D ( 'NONE', #2081, #71486, #32958 ) ;
#21002=PLANE ( 'NONE',  #77345 ) ;
#21011=ORIENTED_EDGE ( 'NONE', *, *, #80093, .T. ) ;
#21016=ORIENTED_EDGE ( 'NONE', *, *, #41376, .T. ) ;
#21025=DIRECTION ( 'NONE',  ( 0.000000000000000000, 0.000000000000000000, 1.000000000000000000 ) ) ;
#21034=VERTEX_POINT ( 'NONE', #14314 ) ;
#21042=CARTESIAN_POINT ( 'NONE',  ( 47.39496755818312579, 108.2889530649357681, -10.00000000000000000 ) ) ;
#21049=EDGE_LOOP ( 'NONE', ( #66987, #50665, #33680, #36674 ) ) ;
#21051=ORIENTED_EDGE ( 'NONE', *, *, #25364, .T. ) ;
#21053=CARTESIAN_POINT ( 'NONE',  ( 48.48788556946983874, 102.1758113618167982, 10.00000000000000000 ) ) ;
#21058=EDGE_CURVE ( 'NONE', #3024, #63370, #55775, .T. ) ;
#21065=ORIENTED_EDGE ( 'NONE', *, *, #9843, .T. ) ;
#21069=CIRCLE ( 'NONE', #3279, 49.99999999999999289 ) ;
#21077=PLANE ( 'NONE',  #28540 ) ;
#21085=CYLINDRICAL_SURFACE ( 'NONE', #28961, 49.99999999999999289 ) ;
#21096=DIRECTION ( 'NONE',  ( -1.000000000000000000, 0.000000000000000000, 0.000000000000000000 ) ) ;
#21099=LINE ( 'NONE', #52961, #38797 ) ;
#21103=CYLINDRICAL_SURFACE ( 'NONE', #83944, 70.00000000000002842 ) ;
#21107=DIRECTION ( 'NONE',  ( 0.000000000000000000, -0.000000000000000000, -1.000000000000000000 ) ) ;
#21118=AXIS2_PLACEMENT_3D ( 'NONE', #34399, #65297, #43971 ) ;
#21128=FACE_OUTER_BOUND ( 'NONE', #71795, .T. ) ;
#21136=LINE ( 'NONE', #59591, #93041 ) ;
#21144=LINE ( 'NONE', #77704, #84515 ) ;
#21145=ORIENTED_EDGE ( 'NONE', *, *, #6148, .T. ) ;
#21148=LINE ( 'NONE', #21629, #85540 ) ;
#21149=DIRECTION ( 'NONE',  ( -0.000000000000000000, -0.000000000000000000, -1.000000000000000000 ) ) ;
#21152=ORIENTED_EDGE ( 'NONE', *, *, #63015, .T. ) ;
#21161=CARTESIAN_POINT ( 'NONE',  ( 7.864685750751951865, 30.05722773587472929, -10.00000000000000000 ) ) ;
#21180=EDGE_LOOP ( 'NONE', ( #56271, #71660, #82731, #18567 ) ) ;
#21181=VERTEX_POINT ( 'NONE', #5597 ) ;
#21186=CARTESIAN_POINT ( 'NONE',  ( -26.39329008703066748, 34.77772847211986829, 59.99999999999999289 ) ) ;
#21190=LINE ( 'NONE', #76387, #59167 ) ;
#21192=DIRECTION ( 'NONE',  ( 1.000000000000000000, 0.000000000000000000, 0.000000000000000000 ) ) ;
#21198=ORIENTED_EDGE ( 'NONE', *, *, #78320, .T. ) ;
#21205=DIRECTION ( 'NONE',  ( 0.000000000000000000, -0.000000000000000000, -1.000000000000000000 ) ) ;
#21218=ADVANCED_FACE ( 'NONE', ( #74019 ), #89750, .F. ) ;
#21221=PLANE ( 'NONE',  #52700 ) ;
#21224=CARTESIAN_POINT ( 'NONE',  ( 9.827979128326980174, 29.57595373812808504, 177.5919119679930134 ) ) ;
#21226=DIRECTION ( 'NONE',  ( -0.9974094913373522386, -0.07193265315671491800, 0.000000000000000000 ) ) ;
#21239=EDGE_CURVE ( 'NONE', #66517, #28862, #43593, .T. ) ;
#21247=ORIENTED_EDGE ( 'NONE', *, *, #96749, .T. ) ;
#21248=DIRECTION ( 'NONE',  ( 0.000000000000000000, 0.000000000000000000, 1.000000000000000000 ) ) ;
#21250=DIRECTION ( 'NONE',  ( -0.000000000000000000, -0.000000000000000000, -1.000000000000000000 ) ) ;
#21252=CARTESIAN_POINT ( 'NONE',  ( -73.66720466879951346, 50.53642055324488780, -10.00000000000000000 ) ) ;
#21254=CARTESIAN_POINT ( 'NONE',  ( 45.80758703142363686, 72.03864405183792030, -10.00000000000000000 ) ) ;
#21271=LINE ( 'NONE', #83097, #79499 ) ;
#21282=VERTEX_POINT ( 'NONE', #74897 ) ;
#21285=ORIENTED_EDGE ( 'NONE', *, *, #58981, .F. ) ;
#21289=ADVANCED_FACE ( 'NONE', ( #89158 ), #65282, .F. ) ;
#21294=FACE_OUTER_BOUND ( 'NONE', #23348, .T. ) ;
#21299=LINE ( 'NONE', #73021, #51195 ) ;
#21310=CARTESIAN_POINT ( 'NONE',  ( 25.98835327777827686, 41.64452202306098627, -10.00000000000000000 ) ) ;
#21315=DIRECTION ( 'NONE',  ( -0.9825923819316327856, -0.1857746241280557598, 0.000000000000000000 ) ) ;
#21316=EDGE_LOOP ( 'NONE', ( #25408, #63270, #62858, #21051 ) ) ;
#21320=CARTESIAN_POINT ( 'NONE',  ( 40.70814378237798081, 60.14496435084704018, 10.00000000000000000 ) ) ;
#21328=CARTESIAN_POINT ( 'NONE',  ( -19.65312891409030271, 93.06504152958497400, 10.00000000000000888 ) ) ;
#21329=DIRECTION ( 'NONE',  ( -0.08592509128337570690, 0.9963016002636669866, 0.000000000000000000 ) ) ;
#21341=VECTOR ( 'NONE', #45531, 999.9999999999998863 ) ;
#21365=LINE ( 'NONE', #44635, #29887 ) ;
#21366=FACE_OUTER_BOUND ( 'NONE', #85751, .T. ) ;
#21371=CARTESIAN_POINT ( 'NONE',  ( 32.25894049256043417, 82.26293186637414578, 59.99999999999999289 ) ) ;
#21379=PLANE ( 'NONE',  #27200 ) ;
#21382=ORIENTED_EDGE ( 'NONE', *, *, #29384, .T. ) ;
#21384=EDGE_CURVE ( 'NONE', #80413, #60766, #54045, .T. ) ;
#21385=DIRECTION ( 'NONE',  ( -0.000000000000000000, 0.000000000000000000, 1.000000000000000000 ) ) ;
#21394=EDGE_CURVE ( 'NONE', #91070, #5196, #38857, .T. ) ;
#21399=EDGE_CURVE ( 'NONE', #14302, #43843, #14581, .T. ) ;
#21400=CARTESIAN_POINT ( 'NONE',  ( -69.40242143070356917, 43.82067236826411971, 177.5919119679930134 ) ) ;
#21405=ORIENTED_EDGE ( 'NONE', *, *, #46818, .F. ) ;
#21410=ORIENTED_EDGE ( 'NONE', *, *, #76368, .T. ) ;
#21423=PLANE ( 'NONE',  #75786 ) ;
#21431=CARTESIAN_POINT ( 'NONE',  ( 0.005075371086064872639, 27.18819441265828019, -10.00000000000000000 ) ) ;
#21434=PLANE ( 'NONE',  #74343 ) ;
#21440=VECTOR ( 'NONE', #8830, 1000.000000000000114 ) ;
#21447=DIRECTION ( 'NONE',  ( 0.000000000000000000, 0.000000000000000000, 1.000000000000000000 ) ) ;
#21460=CARTESIAN_POINT ( 'NONE',  ( -25.62627769214124740, 24.57763045674671432, -10.00000000000000000 ) ) ;
#21474=ADVANCED_FACE ( 'NONE', ( #6482 ), #37360, .T. ) ;
#21490=VECTOR ( 'NONE', #40767, 1000.000000000000000 ) ;
#21493=ORIENTED_EDGE ( 'NONE', *, *, #9487, .F. ) ;
#21495=VECTOR ( 'NONE', #23841, 1000.000000000000000 ) ;
#21498=AXIS2_PLACEMENT_3D ( 'NONE', #68330, #99255, #7033 ) ;
#21501=CARTESIAN_POINT ( 'NONE',  ( -11.23413608767112670, 23.57316747377393540, 177.5919119679930134 ) ) ;
#21505=CARTESIAN_POINT ( 'NONE',  ( -77.42978507651396569, 55.80833764325424085, -10.00000000000000000 ) ) ;
#21506=EDGE_CURVE ( 'NONE', #87819, #78948, #34899, .T. ) ;
#21507=CARTESIAN_POINT ( 'NONE',  ( -48.36978223816942801, 29.22654356899180428, 177.5919119679930134 ) ) ;
#21511=CARTESIAN_POINT ( 'NONE',  ( 48.72058909919672942, 76.89514952714607432, 10.00000000000000000 ) ) ;
#21512=CARTESIAN_POINT ( 'NONE',  ( 13.67211979723576931, 32.92651376809308772, 10.00000000000000000 ) ) ;
#21516=FACE_OUTER_BOUND ( 'NONE', #12526, .T. ) ;
#21527=VERTEX_POINT ( 'NONE', #33268 ) ;
#21530=ORIENTED_EDGE ( 'NONE', *, *, #3885, .T. ) ;
#21537=FACE_OUTER_BOUND ( 'NONE', #59865, .T. ) ;
#21541=ORIENTED_EDGE ( 'NONE', *, *, #89686, .T. ) ;
#21544=EDGE_CURVE ( 'NONE', #47670, #82380, #39343, .T. ) ;
#21545=ORIENTED_EDGE ( 'NONE', *, *, #90760, .F. ) ;
#21563=CARTESIAN_POINT ( 'NONE',  ( -71.07364842061382149, 47.42355933771584375, 10.00000000000000000 ) ) ;
#21572=ORIENTED_EDGE ( 'NONE', *, *, #18709, .T. ) ;
#21573=CARTESIAN_POINT ( 'NONE',  ( 0.005075371086064872639, 27.18819441265827308, -10.00000000000000000 ) ) ;
#21583=LINE ( 'NONE', #82922, #59275 ) ;
#21585=VECTOR ( 'NONE', #72117, 1000.000000000000227 ) ;
#21591=DIRECTION ( 'NONE',  ( -0.6857383512133925496, -0.7278481391575704063, 0.000000000000000000 ) ) ;
#21592=CARTESIAN_POINT ( 'NONE',  ( -19.67882664948312765, 93.20451685012037046, 59.99999999999999289 ) ) ;
#21595=EDGE_CURVE ( 'NONE', #76681, #60766, #93092, .T. ) ;
#21598=FACE_OUTER_BOUND ( 'NONE', #65479, .T. ) ;
#21601=EDGE_CURVE ( 'NONE', #57534, #34490, #9023, .T. ) ;
#21602=EDGE_CURVE ( 'NONE', #30966, #19346, #51458, .T. ) ;
#21606=CARTESIAN_POINT ( 'NONE',  ( -31.60385337846877718, 62.05373366572042926, -10.00000000000000000 ) ) ;
#21610=LINE ( 'NONE', #39268, #92430 ) ;
#21611=DIRECTION ( 'NONE',  ( 0.1887253692075822886, -0.9820299053580098247, 0.000000000000000000 ) ) ;
#21617=DIRECTION ( 'NONE',  ( -0.000000000000000000, -0.000000000000000000, -1.000000000000000000 ) ) ;
#21620=EDGE_LOOP ( 'NONE', ( #11809, #26138, #27929, #74974 ) ) ;
#21624=DIRECTION ( 'NONE',  ( 0.9347244501068350253, 0.3553733281669786970, 0.000000000000000000 ) ) ;
#21626=ORIENTED_EDGE ( 'NONE', *, *, #19434, .T. ) ;
#21629=CARTESIAN_POINT ( 'NONE',  ( 47.96820964746023463, 80.67316705762479501, 10.00000000000000000 ) ) ;
#21631=ORIENTED_EDGE ( 'NONE', *, *, #27427, .T. ) ;
#21633=VERTEX_POINT ( 'NONE', #12990 ) ;
#21660=ORIENTED_EDGE ( 'NONE', *, *, #15260, .T. ) ;
#21665=EDGE_CURVE ( 'NONE', #75787, #1098, #26178, .T. ) ;
#21670=CARTESIAN_POINT ( 'NONE',  ( -77.58047734835668052, 56.02942318228900120, -10.00000000000000000 ) ) ;
#21674=EDGE_LOOP ( 'NONE', ( #21826, #59491, #17902, #51437 ) ) ;
#21675=CARTESIAN_POINT ( 'NONE',  ( 28.00427808217458647, 41.79349426999503692, -10.00000000000000000 ) ) ;
#21682=CARTESIAN_POINT ( 'NONE',  ( -8.669243101527598583, 25.19333184544591475, -10.00000000000000000 ) ) ;
#21683=FACE_OUTER_BOUND ( 'NONE', #61724, .T. ) ;
#21692=DIRECTION ( 'NONE',  ( -0.000000000000000000, -0.000000000000000000, -1.000000000000000000 ) ) ;
#21693=CARTESIAN_POINT ( 'NONE',  ( -80.27490717900100492, 58.06504152958491005, 10.00000000000000888 ) ) ;
#21699=DIRECTION ( 'NONE',  ( 0.000000000000000000, 0.000000000000000000, 1.000000000000000000 ) ) ;
#21705=CARTESIAN_POINT ( 'NONE',  ( -46.49770490450612215, 29.77544742692501600, -10.00000000000000000 ) ) ;
#21708=VECTOR ( 'NONE', #66419, 1000.000000000000000 ) ;
#21710=DIRECTION ( 'NONE',  ( -0.000000000000000000, -0.000000000000000000, -1.000000000000000000 ) ) ;
#21711=VECTOR ( 'NONE', #90173, 1000.000000000000000 ) ;
#21721=DIRECTION ( 'NONE',  ( -0.9140770918436990078, -0.4055404667435369426, 0.000000000000000000 ) ) ;
#21727=DIRECTION ( 'NONE',  ( -0.000000000000000000, 0.000000000000000000, -1.000000000000000000 ) ) ;
#21738=ORIENTED_EDGE ( 'NONE', *, *, #14349, .T. ) ;
#21749=CARTESIAN_POINT ( 'NONE',  ( -56.06787742410712383, 34.75406423768147590, 10.00000000000000000 ) ) ;
#21750=ORIENTED_EDGE ( 'NONE', *, *, #21901, .T. ) ;
#21752=CARTESIAN_POINT ( 'NONE',  ( 33.47037235539275457, 49.41749479597460493, -10.00000000000000000 ) ) ;
#21753=VERTEX_POINT ( 'NONE', #88038 ) ;
#21772=FACE_BOUND ( 'NONE', #26126, .T. ) ;
#21781=VERTEX_POINT ( 'NONE', #24425 ) ;
#21782=CIRCLE ( 'NONE', #18616, 70.00000000000001421 ) ;
#21797=ORIENTED_EDGE ( 'NONE', *, *, #12664, .T. ) ;
#21807=DIRECTION ( 'NONE',  ( -0.8902628732232698017, 0.4554470513245731933, 0.000000000000000000 ) ) ;
#21813=VECTOR ( 'NONE', #4691, 1000.000000000000114 ) ;
#21816=EDGE_CURVE ( 'NONE', #23113, #79865, #91003, .T. ) ;
#21826=ORIENTED_EDGE ( 'NONE', *, *, #93450, .T. ) ;
#21827=EDGE_CURVE ( 'NONE', #29478, #23143, #95388, .T. ) ;
#21829=FACE_OUTER_BOUND ( 'NONE', #2748, .T. ) ;
#21861=ORIENTED_EDGE ( 'NONE', *, *, #18709, .F. ) ;
#21863=DIRECTION ( 'NONE',  ( 0.4829524219151267173, -0.8756465943326184886, 0.000000000000000000 ) ) ;
#21866=CARTESIAN_POINT ( 'NONE',  ( 22.87549206224920439, 39.05096577487528009, -10.00000000000000000 ) ) ;
#21881=EDGE_CURVE ( 'NONE', #31813, #60349, #5123, .T. ) ;
#21888=EDGE_CURVE ( 'NONE', #56406, #92904, #73534, .T. ) ;
#21889=ORIENTED_EDGE ( 'NONE', *, *, #40732, .T. ) ;
#21890=CARTESIAN_POINT ( 'NONE',  ( -17.55320919825948778, 75.98467192273231774, 13.40974089753184195 ) ) ;
#21892=DIRECTION ( 'NONE',  ( -0.000000000000000000, -0.000000000000000000, -1.000000000000000000 ) ) ;
#21901=EDGE_CURVE ( 'NONE', #56569, #98290, #66418, .T. ) ;
#21922=VERTEX_POINT ( 'NONE', #20332 ) ;
#21929=CARTESIAN_POINT ( 'NONE',  ( -76.23101443460923576, 54.01191295053621388, -10.00000000000000000 ) ) ;
#21939=DIRECTION ( 'NONE',  ( -0.000000000000000000, -0.000000000000000000, 1.000000000000000000 ) ) ;
#21944=ADVANCED_FACE ( 'NONE', ( #37981 ), #37490, .F. ) ;
#21948=ADVANCED_FACE ( 'NONE', ( #78017 ), #92258, .F. ) ;
#21963=DIRECTION ( 'NONE',  ( -0.9932214622066116716, 0.1162373735601425623, 0.000000000000000000 ) ) ;
#21977=ORIENTED_EDGE ( 'NONE', *, *, #30850, .T. ) ;
#21985=AXIS2_PLACEMENT_3D ( 'NONE', #30272, #45950, #44464 ) ;
#21986=AXIS2_PLACEMENT_3D ( 'NONE', #48510, #71318, #25715 ) ;
#21987=CARTESIAN_POINT ( 'NONE',  ( -3.216670782107629911, 25.02209300385173663, 177.5919119679930134 ) ) ;
#21988=DIRECTION ( 'NONE',  ( 0.5102188382608533468, -0.8600446134263880493, 0.000000000000000000 ) ) ;
#21989=CIRCLE ( 'NONE', #33350, 70.00000000000001421 ) ;
#22013=ORIENTED_EDGE ( 'NONE', *, *, #1628, .T. ) ;
#22016=ORIENTED_EDGE ( 'NONE', *, *, #87191, .T. ) ;
#22018=ORIENTED_EDGE ( 'NONE', *, *, #95774, .T. ) ;
#22020=FACE_OUTER_BOUND ( 'NONE', #67216, .T. ) ;
#22021=CARTESIAN_POINT ( 'NONE',  ( 48.74043828842092552, 100.0309547576005258, 10.00000000000000000 ) ) ;
#22030=ORIENTED_EDGE ( 'NONE', *, *, #899, .T. ) ;
#22034=DIRECTION ( 'NONE',  ( -0.5632146860273805622, 0.8263106059122556912, 0.000000000000000000 ) ) ;
#22036=ADVANCED_FACE ( 'NONE', ( #91741 ), #15691, .F. ) ;
#22043=VERTEX_POINT ( 'NONE', #31394 ) ;
#22045=CARTESIAN_POINT ( 'NONE',  ( 43.54657591670569872, 62.36930841191391295, -10.00000000000000000 ) ) ;
#22058=CARTESIAN_POINT ( 'NONE',  ( -19.65312891409030271, 93.06504152958497400, 10.00000000000000888 ) ) ;
#22059=CARTESIAN_POINT ( 'NONE',  ( 38.04107491472452551, 53.42442038713602415, 10.00000000000000000 ) ) ;
#22062=CIRCLE ( 'NONE', #20494, 0.1418229129681565781 ) ;
#22078=DIRECTION ( 'NONE',  ( -1.000000000000000000, 0.000000000000000000, 0.000000000000000000 ) ) ;
#22087=FACE_OUTER_BOUND ( 'NONE', #19813, .T. ) ;
#22096=DIRECTION ( 'NONE',  ( 0.000000000000000000, 0.000000000000000000, 1.000000000000000000 ) ) ;
#22097=AXIS2_PLACEMENT_3D ( 'NONE', #42793, #58502, #28607 ) ;
#22101=EDGE_LOOP ( 'NONE', ( #83359, #5559, #22514, #75653 ) ) ;
#22103=CARTESIAN_POINT ( 'NONE',  ( 48.05801951159152452, 75.31115804243518141, 10.00000000000000000 ) ) ;
#22125=CARTESIAN_POINT ( 'NONE',  ( -34.46923751714648887, 63.31602547000201042, -10.00000000000000000 ) ) ;
#22129=DIRECTION ( 'NONE',  ( -0.5864613938488684175, 0.8099771808667466377, 0.000000000000000000 ) ) ;
#22130=VECTOR ( 'NONE', #24438, 1000.000000000000000 ) ;
#22136=AXIS2_PLACEMENT_3D ( 'NONE', #41984, #42955, #81045 ) ;
#22138=ORIENTED_EDGE ( 'NONE', *, *, #85187, .T. ) ;
#22139=VERTEX_POINT ( 'NONE', #78521 ) ;
#22142=DIRECTION ( 'NONE',  ( -0.9919422576440838357, -0.1266907948509198578, 0.000000000000000000 ) ) ;
#22143=DIRECTION ( 'NONE',  ( -0.9981117208278915687, 0.06142469166373833167, 0.000000000000000000 ) ) ;
#22155=CARTESIAN_POINT ( 'NONE',  ( 46.15481705937101964, 68.45315478587873770, 10.00000000000000000 ) ) ;
#22163=EDGE_CURVE ( 'NONE', #40778, #69110, #79553, .T. ) ;
#22168=EDGE_LOOP ( 'NONE', ( #29738, #58287, #86115, #91170 ) ) ;
#22169=DIRECTION ( 'NONE',  ( 1.000000000000000000, 1.768426674938641735E-13, 0.000000000000000000 ) ) ;
#22173=CARTESIAN_POINT ( 'NONE',  ( -19.65312891409030271, 93.06504152958497400, 177.5919119679930134 ) ) ;
#22179=VERTEX_POINT ( 'NONE', #11126 ) ;
#22181=CARTESIAN_POINT ( 'NONE',  ( -64.54732778733693976, 39.35739861417317087, -10.00000000000000000 ) ) ;
#22223=DIRECTION ( 'NONE',  ( -0.2197389712097134185, -0.9755587037855265597, 0.000000000000000000 ) ) ;
#22240=ORIENTED_EDGE ( 'NONE', *, *, #43385, .F. ) ;
#22245=ORIENTED_EDGE ( 'NONE', *, *, #16007, .T. ) ;
#22249=ORIENTED_EDGE ( 'NONE', *, *, #56926, .F. ) ;
#22253=CARTESIAN_POINT ( 'NONE',  ( 30.87961294008499635, 109.1271249547276341, 59.99999999999999289 ) ) ;
#22263=EDGE_LOOP ( 'NONE', ( #28365, #15620, #89667, #52826 ) ) ;
#22267=VECTOR ( 'NONE', #55647, 1000.000000000000114 ) ;
#22270=ORIENTED_EDGE ( 'NONE', *, *, #51184, .F. ) ;
#22271=FACE_BOUND ( 'NONE', #71682, .T. ) ;
#22275=CARTESIAN_POINT ( 'NONE',  ( -3.153128914090298274, 64.48620320469859735, 0.000000000000000000 ) ) ;
#22277=EDGE_CURVE ( 'NONE', #79746, #88881, #89648, .T. ) ;
#22278=DIRECTION ( 'NONE',  ( -0.000000000000000000, -0.000000000000000000, 1.000000000000000000 ) ) ;
#22282=VECTOR ( 'NONE', #58924, 1000.000000000000000 ) ;
#22300=LINE ( 'NONE', #30898, #38871 ) ;
#22312=DIRECTION ( 'NONE',  ( -0.9439450758449140499, 0.3301025504114431519, 0.000000000000000000 ) ) ;
#22316=DIRECTION ( 'NONE',  ( 1.000000000000000000, 0.000000000000000000, 0.000000000000000000 ) ) ;
#22322=DIRECTION ( 'NONE',  ( 0.8393827800519358950, 0.5435407515102096410, 0.000000000000000000 ) ) ;
#22324=VECTOR ( 'NONE', #60114, 1000.000000000000000 ) ;
#22343=VECTOR ( 'NONE', #89416, 1000.000000000000227 ) ;
#22350=CARTESIAN_POINT ( 'NONE',  ( 29.12701137275935181, 44.61184105132205957, -10.00000000000000000 ) ) ;
#22354=CARTESIAN_POINT ( 'NONE',  ( -19.65312891409030271, 93.06504152958497400, 59.99999999999999289 ) ) ;
#22359=VERTEX_POINT ( 'NONE', #32776 ) ;
#22363=ORIENTED_EDGE ( 'NONE', *, *, #89267, .F. ) ;
#22370=ORIENTED_EDGE ( 'NONE', *, *, #84497, .T. ) ;
#22376=DIRECTION ( 'NONE',  ( 0.000000000000000000, 0.000000000000000000, 1.000000000000000000 ) ) ;
#22385=VECTOR ( 'NONE', #87023, 1000.000000000000114 ) ;
#22390=CARTESIAN_POINT ( 'NONE',  ( -64.54732778733692555, 39.35739861417317087, 177.5919119679930134 ) ) ;
#22392=CARTESIAN_POINT ( 'NONE',  ( -14.75193346722050158, 72.91080179107989068, 13.82017248825341937 ) ) ;
#22393=CARTESIAN_POINT ( 'NONE',  ( -73.83803415018343230, 50.74234351129840093, -10.00000000000000000 ) ) ;
#22394=DIRECTION ( 'NONE',  ( -0.7080737730998226676, 0.7061384650677096086, 0.000000000000000000 ) ) ;
#22395=LINE ( 'NONE', #13799, #25304 ) ;
#22398=AXIS2_PLACEMENT_3D ( 'NONE', #68983, #21892, #38069 ) ;
#22418=CARTESIAN_POINT ( 'NONE',  ( 3.318370377354149081, 69.04773004486530397, -10.00000000000000000 ) ) ;
#22430=CARTESIAN_POINT ( 'NONE',  ( 36.25628400652970384, 53.06077264917335157, -10.00000000000000000 ) ) ;
#22435=FACE_OUTER_BOUND ( 'NONE', #48337, .T. ) ;
#22439=FACE_OUTER_BOUND ( 'NONE', #69347, .T. ) ;
#22448=AXIS2_PLACEMENT_3D ( 'NONE', #515, #99335, #31402 ) ;
#22451=VECTOR ( 'NONE', #35615, 1000.000000000000114 ) ;
#22465=ORIENTED_EDGE ( 'NONE', *, *, #71565, .T. ) ;
#22473=LINE ( 'NONE', #53366, #58136 ) ;
#22476=CARTESIAN_POINT ( 'NONE',  ( 47.03029105687465261, 114.3563895605556269, 10.00000000000000000 ) ) ;
#22477=DIRECTION ( 'NONE',  ( -0.4242989612870696758, 0.9055221650797476984, 0.000000000000000000 ) ) ;
#22482=LINE ( 'NONE', #78191, #92020 ) ;
#22483=CARTESIAN_POINT ( 'NONE',  ( -76.38857681351474582, 54.22815603855766398, 10.00000000000000000 ) ) ;
#22484=VERTEX_POINT ( 'NONE', #89610 ) ;
#22511=ORIENTED_EDGE ( 'NONE', *, *, #41492, .T. ) ;
#22514=ORIENTED_EDGE ( 'NONE', *, *, #26269, .F. ) ;
#22516=ORIENTED_EDGE ( 'NONE', *, *, #92628, .F. ) ;
#22517=LINE ( 'NONE', #216, #37888 ) ;
#22519=EDGE_CURVE ( 'NONE', #99910, #83671, #69236, .T. ) ;
#22529=ORIENTED_EDGE ( 'NONE', *, *, #13785, .F. ) ;
#22533=CARTESIAN_POINT ( 'NONE',  ( -68.10632939235270555, 44.28490124273479012, 10.00000000000000000 ) ) ;
#22536=ORIENTED_EDGE ( 'NONE', *, *, #66494, .F. ) ;
#22545=ORIENTED_EDGE ( 'NONE', *, *, #64042, .F. ) ;
#22548=DIRECTION ( 'NONE',  ( -0.9991767892008870389, -0.04056776950001317328, 0.000000000000000000 ) ) ;
#22551=CARTESIAN_POINT ( 'NONE',  ( 29.30989995549245464, 44.80713248141895377, -10.00000000000000000 ) ) ;
#22557=AXIS2_PLACEMENT_3D ( 'NONE', #32575, #63471, #94407 ) ;
#22561=CARTESIAN_POINT ( 'NONE',  ( 50.60128122559382291, 92.19983735941717384, -10.00000000000000000 ) ) ;
#22571=CARTESIAN_POINT ( 'NONE',  ( 24.35067441160642687, 40.23626134430271861, 10.00000000000000000 ) ) ;
#22573=DIRECTION ( 'NONE',  ( -0.06442261589617469253, -0.9979227057047523886, 0.000000000000000000 ) ) ;
#22576=DIRECTION ( 'NONE',  ( -1.000000000000000000, 4.892646582057217816E-14, 0.000000000000000000 ) ) ;
#22587=DIRECTION ( 'NONE',  ( -1.000000000000000000, 0.000000000000000000, 0.000000000000000000 ) ) ;
#22591=EDGE_CURVE ( 'NONE', #36742, #45792, #70231, .T. ) ;
#22604=CIRCLE ( 'NONE', #63026, 0.1418229129681591871 ) ;
#22609=VERTEX_POINT ( 'NONE', #89020 ) ;
#22610=EDGE_CURVE ( 'NONE', #10180, #17718, #7424, .T. ) ;
#22615=VECTOR ( 'NONE', #26681, 1000.000000000000114 ) ;
#22634=AXIS2_PLACEMENT_3D ( 'NONE', #95276, #10124, #80563 ) ;
#22653=EDGE_CURVE ( 'NONE', #58863, #5335, #75249, .T. ) ;
#22659=EDGE_LOOP ( 'NONE', ( #44848, #35201, #65489, #8179 ) ) ;
#22663=EDGE_CURVE ( 'NONE', #55387, #82505, #20551, .T. ) ;
#22665=ADVANCED_FACE ( 'NONE', ( #35235 ), #51938, .F. ) ;
#22676=VERTEX_POINT ( 'NONE', #81876 ) ;
#22678=VECTOR ( 'NONE', #42815, 1000.000000000000114 ) ;
#22680=DIRECTION ( 'NONE',  ( -0.000000000000000000, -0.000000000000000000, -1.000000000000000000 ) ) ;
#22690=CARTESIAN_POINT ( 'NONE',  ( -7.521556465916529710, 24.12430647450515053, 10.00000000000000000 ) ) ;
#22692=LINE ( 'NONE', #60163, #79293 ) ;
#22705=DIRECTION ( 'NONE',  ( -0.000000000000000000, -0.000000000000000000, -1.000000000000000000 ) ) ;
#22730=ADVANCED_FACE ( 'NONE', ( #22020 ), #73745, .F. ) ;
#22731=EDGE_CURVE ( 'NONE', #87101, #29478, #89971, .T. ) ;
#22737=VERTEX_POINT ( 'NONE', #59509 ) ;
#22738=CARTESIAN_POINT ( 'NONE',  ( 50.23025173566475132, 97.10399052176643409, 10.00000000000000000 ) ) ;
#22742=CARTESIAN_POINT ( 'NONE',  ( -63.08903959183645327, 39.77784189046417396, -10.00000000000000000 ) ) ;
#22776=PLANE ( 'NONE',  #956 ) ;
#22778=FACE_BOUND ( 'NONE', #27557, .T. ) ;
#22789=VERTEX_POINT ( 'NONE', #90977 ) ;
#22792=ADVANCED_FACE ( 'NONE', ( #21537 ), #83365, .T. ) ;
#22794=CARTESIAN_POINT ( 'NONE',  ( 32.30839531297598910, 123.0650415295850593, -40.00000000000000000 ) ) ;
#22803=CARTESIAN_POINT ( 'NONE',  ( -19.65312891409030271, 93.06504152958497400, -10.00000000000000888 ) ) ;
#22807=DIRECTION ( 'NONE',  ( 0.09248003802711830812, -0.9957145386939485476, 0.000000000000000000 ) ) ;
#22819=CARTESIAN_POINT ( 'NONE',  ( -72.39633208959961053, 47.04162880533178992, -10.00000000000000000 ) ) ;
#22822=DIRECTION ( 'NONE',  ( 0.8755176446346986108, -0.4831861483251662648, 0.000000000000000000 ) ) ;
#22839=EDGE_CURVE ( 'NONE', #43149, #78972, #54390, .T. ) ;
#22841=DIRECTION ( 'NONE',  ( -0.7845058662180028897, -0.6201213960746241316, 0.000000000000000000 ) ) ;
#22859=ORIENTED_EDGE ( 'NONE', *, *, #15139, .F. ) ;
#22860=PLANE ( 'NONE',  #39248 ) ;
#22865=ORIENTED_EDGE ( 'NONE', *, *, #17098, .F. ) ;
#22866=LINE ( 'NONE', #5678, #71370 ) ;
#22867=DIRECTION ( 'NONE',  ( -0.000000000000000000, 0.000000000000000000, 1.000000000000000000 ) ) ;
#22872=DIRECTION ( 'NONE',  ( 0.3693965786901519111, -0.9292718480896805522, 0.000000000000000000 ) ) ;
#22873=ORIENTED_EDGE ( 'NONE', *, *, #84999, .T. ) ;
#22876=CARTESIAN_POINT ( 'NONE',  ( 35.56482384635839367, 110.6301519124606756, 59.99999999999999289 ) ) ;
#22882=CARTESIAN_POINT ( 'NONE',  ( -13.14444822889210762, 72.23936417694854129, 14.22349210779893625 ) ) ;
#22884=CARTESIAN_POINT ( 'NONE',  ( -17.26243516413818924, 24.35187462261283997, 10.00000000000000000 ) ) ;
#22887=VERTEX_POINT ( 'NONE', #92461 ) ;
#22900=DIRECTION ( 'NONE',  ( 0.000000000000000000, -0.000000000000000000, -1.000000000000000000 ) ) ;
#22905=CARTESIAN_POINT ( 'NONE',  ( 36.38358746446922254, 51.11404133282111673, -10.00000000000000000 ) ) ;
#22917=FACE_OUTER_BOUND ( 'NONE', #44197, .T. ) ;
#22924=ORIENTED_EDGE ( 'NONE', *, *, #8854, .T. ) ;
#22931=CARTESIAN_POINT ( 'NONE',  ( 5.181765596169280563, 27.61866642244642023, 177.5919119679930134 ) ) ;
#22932=CARTESIAN_POINT ( 'NONE',  ( -71.61465314115659453, 63.06504152958490295, 203.6502102582797420 ) ) ;
#22936=ORIENTED_EDGE ( 'NONE', *, *, #78821, .T. ) ;
#22943=PLANE ( 'NONE',  #57782 ) ;
#22965=LINE ( 'NONE', #37177, #53552 ) ;
#22975=CARTESIAN_POINT ( 'NONE',  ( 48.81784752633560487, 86.82484054835779830, 10.00000000000000000 ) ) ;
#22984=DIRECTION ( 'NONE',  ( 0.8434505012732891327, -0.5372068985985168910, 0.000000000000000000 ) ) ;
#22991=VECTOR ( 'NONE', #83105, 1000.000000000000227 ) ;
#22998=ORIENTED_EDGE ( 'NONE', *, *, #47829, .F. ) ;
#23001=ORIENTED_EDGE ( 'NONE', *, *, #4555, .F. ) ;
#23013=PLANE ( 'NONE',  #31637 ) ;
#23016=ORIENTED_EDGE ( 'NONE', *, *, #54765, .F. ) ;
#23025=DIRECTION ( 'NONE',  ( -0.8615733660689046669, -0.5076330711061851630, 0.000000000000000000 ) ) ;
#23031=DIRECTION ( 'NONE',  ( -0.7548338719222550397, 0.6559160203858850346, 0.000000000000000000 ) ) ;
#23034=ORIENTED_EDGE ( 'NONE', *, *, #95752, .T. ) ;
#23051=AXIS2_PLACEMENT_3D ( 'NONE', #24479, #87370, #48287 ) ;
#23058=EDGE_CURVE ( 'NONE', #62248, #10169, #59176, .T. ) ;
#23068=EDGE_CURVE ( 'NONE', #28623, #48026, #59382, .T. ) ;
#23073=EDGE_CURVE ( 'NONE', #88859, #85517, #31704, .T. ) ;
#23075=AXIS2_PLACEMENT_3D ( 'NONE', #61529, #62009, #13947 ) ;
#23081=DIRECTION ( 'NONE',  ( 0.000000000000000000, 0.000000000000000000, 1.000000000000000000 ) ) ;
#23092=CARTESIAN_POINT ( 'NONE',  ( -19.65312891409030271, 93.06504152958497400, 59.99999999999999289 ) ) ;
#23096=FACE_OUTER_BOUND ( 'NONE', #68577, .T. ) ;
#23103=ORIENTED_EDGE ( 'NONE', *, *, #14634, .T. ) ;
#23109=FACE_OUTER_BOUND ( 'NONE', #43582, .T. ) ;
#23113=VERTEX_POINT ( 'NONE', #35613 ) ;
#23116=ORIENTED_EDGE ( 'NONE', *, *, #15079, .T. ) ;
#23123=DIRECTION ( 'NONE',  ( 0.000000000000000000, 0.000000000000000000, 1.000000000000000000 ) ) ;
#23126=CYLINDRICAL_SURFACE ( 'NONE', #95486, 70.00000000000002842 ) ;
#23132=ORIENTED_EDGE ( 'NONE', *, *, #28836, .T. ) ;
#23133=ADVANCED_FACE ( 'NONE', ( #19932 ), #19454, .F. ) ;
#23137=EDGE_CURVE ( 'NONE', #97892, #82529, #12298, .T. ) ;
#23138=CARTESIAN_POINT ( 'NONE',  ( -71.61465314115659453, 63.06504152958490295, -60.00000000000000000 ) ) ;
#23142=CARTESIAN_POINT ( 'NONE',  ( -65.22359575898936157, 56.10326143670914689, 59.99999999999999289 ) ) ;
#23143=VERTEX_POINT ( 'NONE', #82267 ) ;
#23144=DIRECTION ( 'NONE',  ( -0.000000000000000000, 0.000000000000000000, 1.000000000000000000 ) ) ;
#23151=AXIS2_PLACEMENT_3D ( 'NONE', #71340, #63723, #39396 ) ;
#23159=ORIENTED_EDGE ( 'NONE', *, *, #64821, .T. ) ;
#23167=EDGE_CURVE ( 'NONE', #76243, #51511, #47192, .T. ) ;
#23190=EDGE_CURVE ( 'NONE', #45441, #54753, #34978, .T. ) ;
#23197=DIRECTION ( 'NONE',  ( -0.000000000000000000, 0.000000000000000000, 1.000000000000000000 ) ) ;
#23206=DIRECTION ( 'NONE',  ( -0.8660254037844380415, -0.5000000000000009992, 0.000000000000000000 ) ) ;
#23216=EDGE_LOOP ( 'NONE', ( #56660, #52057, #88102, #83110 ) ) ;
#23217=AXIS2_PLACEMENT_3D ( 'NONE', #20005, #56492, #50884 ) ;
#23224=ORIENTED_EDGE ( 'NONE', *, *, #51085, .F. ) ;
#23226=ORIENTED_EDGE ( 'NONE', *, *, #10876, .F. ) ;
#23229=CARTESIAN_POINT ( 'NONE',  ( -19.65312891409030271, 93.06504152958497400, -40.00000000000000000 ) ) ;
#23233=CARTESIAN_POINT ( 'NONE',  ( 8.106622824862185439, 30.17147933776455204, -10.00000000000000000 ) ) ;
#23238=ORIENTED_EDGE ( 'NONE', *, *, #19700, .F. ) ;
#23243=DIRECTION ( 'NONE',  ( -0.000000000000000000, -0.000000000000000000, 1.000000000000000000 ) ) ;
#23251=VERTEX_POINT ( 'NONE', #76385 ) ;
#23268=ORIENTED_EDGE ( 'NONE', *, *, #2129, .T. ) ;
#23277=VERTEX_POINT ( 'NONE', #60639 ) ;
#23285=VECTOR ( 'NONE', #20051, 1000.000000000000114 ) ;
#23286=CARTESIAN_POINT ( 'NONE',  ( 32.30839531297598910, 123.0650415295850593, 10.00000000000000888 ) ) ;
#23287=ORIENTED_EDGE ( 'NONE', *, *, #79595, .F. ) ;
#23295=AXIS2_PLACEMENT_3D ( 'NONE', #66347, #83083, #82096 ) ;
#23298=PLANE ( 'NONE',  #93887 ) ;
#23307=EDGE_CURVE ( 'NONE', #96434, #7039, #7453, .T. ) ;
#23309=CARTESIAN_POINT ( 'NONE',  ( 29.30989995549245464, 44.80713248141894667, -10.00000000000000000 ) ) ;
#23315=CARTESIAN_POINT ( 'NONE',  ( 31.76832553566411121, 98.72342451966777332, 59.99999999999999289 ) ) ;
#23322=EDGE_CURVE ( 'NONE', #30767, #33732, #39827, .T. ) ;
#23327=DIRECTION ( 'NONE',  ( -0.6201213960746324583, 0.7845058662179964504, 0.000000000000000000 ) ) ;
#23331=CARTESIAN_POINT ( 'NONE',  ( -4.878521687326337286, 80.51981399750955859, 13.50774849792892418 ) ) ;
#23340=LINE ( 'NONE', #30949, #51545 ) ;
#23341=LINE ( 'NONE', #54229, #21495 ) ;
#23348=EDGE_LOOP ( 'NONE', ( #11556, #86494, #10754, #78662 ) ) ;
#23349=DIRECTION ( 'NONE',  ( -0.9708212084269268738, 0.2398044646550215042, 0.000000000000000000 ) ) ;
#23351=CARTESIAN_POINT ( 'NONE',  ( -66.34925969370661392, 42.61035540433362456, -10.00000000000000000 ) ) ;
#23355=ORIENTED_EDGE ( 'NONE', *, *, #31964, .F. ) ;
#23357=ORIENTED_EDGE ( 'NONE', *, *, #94207, .T. ) ;
#23365=CIRCLE ( 'NONE', #36319, 70.00000000000001421 ) ;
#23367=ORIENTED_EDGE ( 'NONE', *, *, #3285, .T. ) ;
#23369=CARTESIAN_POINT ( 'NONE',  ( 42.32809528168264990, 126.1521775423068163, 10.00000000000000000 ) ) ;
#23374=ORIENTED_EDGE ( 'NONE', *, *, #62981, .T. ) ;
#23375=PLANE ( 'NONE',  #95141 ) ;
#23378=CARTESIAN_POINT ( 'NONE',  ( -59.29375005653866282, 35.37083770076974076, 177.5919119679930134 ) ) ;
#23379=EDGE_LOOP ( 'NONE', ( #86465, #50146, #4722, #89582 ) ) ;
#23384=ORIENTED_EDGE ( 'NONE', *, *, #83883, .T. ) ;
#23401=EDGE_CURVE ( 'NONE', #58030, #48601, #46958, .T. ) ;
#23420=CARTESIAN_POINT ( 'NONE',  ( -69.85371643402891095, 44.28081239092799848, 177.5919119679930134 ) ) ;
#23424=VECTOR ( 'NONE', #69123, 1000.000000000000000 ) ;
#23425=CARTESIAN_POINT ( 'NONE',  ( -19.65312891409030271, 93.06504152958497400, -60.00000000000000000 ) ) ;
#23430=DIRECTION ( 'NONE',  ( 1.000000000000000000, 0.000000000000000000, 0.000000000000000000 ) ) ;
#23431=VERTEX_POINT ( 'NONE', #88523 ) ;
#23432=AXIS2_PLACEMENT_3D ( 'NONE', #26486, #72604, #10785 ) ;
#23438=DIRECTION ( 'NONE',  ( 0.000000000000000000, -0.000000000000000000, -1.000000000000000000 ) ) ;
#23439=PLANE ( 'NONE',  #29679 ) ;
#23457=DIRECTION ( 'NONE',  ( 1.000000000000000000, 0.000000000000000000, 0.000000000000000000 ) ) ;
#23460=DIRECTION ( 'NONE',  ( 0.1266907948509090887, -0.9919422576440851680, 0.000000000000000000 ) ) ;
#23464=VECTOR ( 'NONE', #97267, 1000.000000000000114 ) ;
#23470=CYLINDRICAL_SURFACE ( 'NONE', #6332, 14.99999999999967493 ) ;
#23472=VERTEX_POINT ( 'NONE', #56554 ) ;
#23475=ORIENTED_EDGE ( 'NONE', *, *, #50394, .F. ) ;
#23488=CARTESIAN_POINT ( 'NONE',  ( 48.29091023345864642, 82.53782597618220507, 10.00000000000000000 ) ) ;
#23489=ORIENTED_EDGE ( 'NONE', *, *, #68382, .F. ) ;
#23490=ORIENTED_EDGE ( 'NONE', *, *, #72763, .F. ) ;
#23493=VECTOR ( 'NONE', #19919, 1000.000000000000000 ) ;
#23496=EDGE_LOOP ( 'NONE', ( #26354, #46080, #57923, #60999 ) ) ;
#23509=ORIENTED_EDGE ( 'NONE', *, *, #23307, .F. ) ;
#23517=ADVANCED_FACE ( 'NONE', ( #82893 ), #21077, .F. ) ;
#23520=VERTEX_POINT ( 'NONE', #5358 ) ;
#23523=DIRECTION ( 'NONE',  ( -0.4340522123146939859, 0.9008877160804890094, 0.000000000000000000 ) ) ;
#23529=LINE ( 'NONE', #53437, #83900 ) ;
#23538=AXIS2_PLACEMENT_3D ( 'NONE', #42462, #12599, #34868 ) ;
#23548=DIRECTION ( 'NONE',  ( -0.3696446237802352708, -0.9291732088853876803, 0.000000000000000000 ) ) ;
#23552=AXIS2_PLACEMENT_3D ( 'NONE', #29794, #21699, #392 ) ;
#23553=LINE ( 'NONE', #76302, #20881 ) ;
#23560=LINE ( 'NONE', #54452, #5941 ) ;
#23561=ORIENTED_EDGE ( 'NONE', *, *, #68907, .F. ) ;
#23562=AXIS2_PLACEMENT_3D ( 'NONE', #39220, #40225, #78261 ) ;
#23563=DIRECTION ( 'NONE',  ( -1.000000000000000000, 0.000000000000000000, 0.000000000000000000 ) ) ;
#23574=DIRECTION ( 'NONE',  ( -0.000000000000000000, -0.000000000000000000, -1.000000000000000000 ) ) ;
#23575=EDGE_CURVE ( 'NONE', #100024, #69721, #74779, .T. ) ;
#23591=VERTEX_POINT ( 'NONE', #68631 ) ;
#23598=VERTEX_POINT ( 'NONE', #75265 ) ;
#23603=AXIS2_PLACEMENT_3D ( 'NONE', #71300, #81300, #73666 ) ;
#23610=VERTEX_POINT ( 'NONE', #35753 ) ;
#23613=ORIENTED_EDGE ( 'NONE', *, *, #85332, .F. ) ;
#23628=VECTOR ( 'NONE', #50344, 1000.000000000000227 ) ;
#23633=CARTESIAN_POINT ( 'NONE',  ( 49.83874514172083536, 101.4840343560033915, -10.00000000000000000 ) ) ;
#23638=VECTOR ( 'NONE', #94140, 1000.000000000000000 ) ;
#23641=VERTEX_POINT ( 'NONE', #67642 ) ;
#23644=VERTEX_POINT ( 'NONE', #98574 ) ;
#23645=ADVANCED_FACE ( 'NONE', ( #83383 ), #13949, .F. ) ;
#23658=LINE ( 'NONE', #67406, #99171 ) ;
#23671=VECTOR ( 'NONE', #92123, 1000.000000000000114 ) ;
#23674=VECTOR ( 'NONE', #30968, 1000.000000000000000 ) ;
#23682=FACE_OUTER_BOUND ( 'NONE', #65080, .T. ) ;
#23690=CARTESIAN_POINT ( 'NONE',  ( 35.19727222974664471, 74.38379681254539832, 59.99999999999999289 ) ) ;
#23694=AXIS2_PLACEMENT_3D ( 'NONE', #31775, #15577, #100219 ) ;
#23705=CIRCLE ( 'NONE', #46335, 45.00000000000000000 ) ;
#23718=ORIENTED_EDGE ( 'NONE', *, *, #76046, .F. ) ;
#23720=ORIENTED_EDGE ( 'NONE', *, *, #97626, .T. ) ;
#23728=DIRECTION ( 'NONE',  ( -0.8098206029991054100, 0.5866775868892259993, 0.000000000000000000 ) ) ;
#23733=ADVANCED_FACE ( 'NONE', ( #5667 ), #5178, .T. ) ;
#23734=CARTESIAN_POINT ( 'NONE',  ( -69.94229046795800286, 43.99946344738946635, 10.00000000000000000 ) ) ;
#23742=CARTESIAN_POINT ( 'NONE',  ( -69.42519150082246426, 45.64199051378594874, -10.00000000000000000 ) ) ;
#23745=CARTESIAN_POINT ( 'NONE',  ( 38.34592905085143855, 84.17966526993892273, 59.99999999999999289 ) ) ;
#23751=VECTOR ( 'NONE', #64020, 1000.000000000000000 ) ;
#23752=EDGE_LOOP ( 'NONE', ( #88368, #82259, #78232, #14028 ) ) ;
#23754=AXIS2_PLACEMENT_3D ( 'NONE', #88227, #65363, #57751 ) ;
#23766=EDGE_CURVE ( 'NONE', #46169, #1959, #38036, .T. ) ;
#23770=AXIS2_PLACEMENT_3D ( 'NONE', #58577, #59061, #28187 ) ;
#23783=VECTOR ( 'NONE', #31728, 1000.000000000000000 ) ;
#23793=DIRECTION ( 'NONE',  ( 1.000000000000000000, 8.921435019309292501E-15, 0.000000000000000000 ) ) ;
#23800=DIRECTION ( 'NONE',  ( 0.000000000000000000, 0.000000000000000000, -1.000000000000000000 ) ) ;
#23808=CARTESIAN_POINT ( 'NONE',  ( 47.83996289752661113, 111.6306699247848826, 177.5919119679930134 ) ) ;
#23812=CARTESIAN_POINT ( 'NONE',  ( -2.330697855141256269, 26.52822386297705393, 10.00000000000000000 ) ) ;
#23815=CARTESIAN_POINT ( 'NONE',  ( -18.45562326176555956, 23.07528527759725989, -10.00000000000000000 ) ) ;
#23825=VECTOR ( 'NONE', #59776, 1000.000000000000341 ) ;
#23828=CARTESIAN_POINT ( 'NONE',  ( 5.871984111234073822, 29.22396284167520619, 10.00000000000000000 ) ) ;
#23835=EDGE_CURVE ( 'NONE', #23520, #68063, #72392, .T. ) ;
#23836=LINE ( 'NONE', #55225, #12721 ) ;
#23837=CARTESIAN_POINT ( 'NONE',  ( -48.34856483818852979, 28.93234566034054822, -10.00000000000000000 ) ) ;
#23841=DIRECTION ( 'NONE',  ( 0.000000000000000000, 0.000000000000000000, 1.000000000000000000 ) ) ;
#23843=VERTEX_POINT ( 'NONE', #88132 ) ;
#23855=EDGE_CURVE ( 'NONE', #61495, #11375, #26769, .T. ) ;
#23856=CARTESIAN_POINT ( 'NONE',  ( -51.48155258352917230, 83.50091703386740960, -10.00000000000000000 ) ) ;
#23858=ORIENTED_EDGE ( 'NONE', *, *, #50367, .T. ) ;
#23859=VECTOR ( 'NONE', #57361, 1000.000000000000227 ) ;
#23869=ORIENTED_EDGE ( 'NONE', *, *, #71711, .F. ) ;
#23877=DIRECTION ( 'NONE',  ( -0.7300871660154544251, -0.6833540297821638632, 0.000000000000000000 ) ) ;
#23883=ADVANCED_FACE ( 'NONE', ( #97202 ), #3965, .F. ) ;
#23891=PLANE ( 'NONE',  #28908 ) ;
#23893=ADVANCED_FACE ( 'NONE', ( #19195 ), #66267, .T. ) ;
#23902=VERTEX_POINT ( 'NONE', #89617 ) ;
#23905=EDGE_CURVE ( 'NONE', #41771, #55869, #20178, .T. ) ;
#23924=ORIENTED_EDGE ( 'NONE', *, *, #47540, .F. ) ;
#23926=CARTESIAN_POINT ( 'NONE',  ( 27.58098951138967436, 43.10352854649765675, -10.00000000000000000 ) ) ;
#23943=LINE ( 'NONE', #71073, #73374 ) ;
#23953=DIRECTION ( 'NONE',  ( -0.8599083858334093389, 0.5104483989331149996, 0.000000000000000000 ) ) ;
#23962=EDGE_CURVE ( 'NONE', #89739, #93198, #72899, .T. ) ;
#23967=LINE ( 'NONE', #1696, #84401 ) ;
#23978=DIRECTION ( 'NONE',  ( -0.9182972510888884887, 0.3958915996110436430, 0.000000000000000000 ) ) ;
#23979=DIRECTION ( 'NONE',  ( -1.000000000000000000, 0.000000000000000000, 0.000000000000000000 ) ) ;
#23980=ADVANCED_FACE ( 'NONE', ( #89136 ), #50549, .T. ) ;
#23993=CIRCLE ( 'NONE', #66022, 70.00000000000001421 ) ;
#24002=ORIENTED_EDGE ( 'NONE', *, *, #49069, .T. ) ;
#24004=EDGE_LOOP ( 'NONE', ( #12365, #69253, #35227, #12059 ) ) ;
#24006=VERTEX_POINT ( 'NONE', #84002 ) ;
#24008=ORIENTED_EDGE ( 'NONE', *, *, #6392, .T. ) ;
#24010=CIRCLE ( 'NONE', #14250, 70.00000000000001421 ) ;
#24012=EDGE_CURVE ( 'NONE', #44226, #41771, #13081, .T. ) ;
#24027=DIRECTION ( 'NONE',  ( -1.000000000000000000, -9.785293164110366372E-14, 0.000000000000000000 ) ) ;
#24034=VECTOR ( 'NONE', #97969, 1000.000000000000000 ) ;
#24049=ORIENTED_EDGE ( 'NONE', *, *, #26198, .F. ) ;
#24062=ORIENTED_EDGE ( 'NONE', *, *, #82016, .F. ) ;
#24065=VECTOR ( 'NONE', #67923, 1000.000000000000000 ) ;
#24089=CARTESIAN_POINT ( 'NONE',  ( 44.08135397534552169, 118.8355609772188188, -10.00000000000000000 ) ) ;
#24090=DIRECTION ( 'NONE',  ( 0.3371987438498062484, -0.9414334852479556703, 0.000000000000000000 ) ) ;
#24091=CARTESIAN_POINT ( 'NONE',  ( -76.86719868626529717, 52.73452925779879763, 177.5919119679930134 ) ) ;
#24092=LINE ( 'NONE', #54988, #96033 ) ;
#24094=CARTESIAN_POINT ( 'NONE',  ( -25.89332989531674301, 24.59406508915897760, -10.00000000000000000 ) ) ;
#24098=EDGE_CURVE ( 'NONE', #30721, #23251, #4324, .T. ) ;
#24101=EDGE_CURVE ( 'NONE', #38684, #32988, #68243, .T. ) ;
#24104=CARTESIAN_POINT ( 'NONE',  ( 48.23560136428437772, 110.1272893647940379, 10.00000000000000000 ) ) ;
#24107=ADVANCED_FACE ( 'NONE', ( #98179 ), #91581, .F. ) ;
#24112=EDGE_CURVE ( 'NONE', #23472, #43827, #12443, .T. ) ;
#24113=CARTESIAN_POINT ( 'NONE',  ( 40.70814378237798081, 60.14496435084704018, -10.00000000000000000 ) ) ;
#24119=DIRECTION ( 'NONE',  ( 0.000000000000000000, 0.000000000000000000, -1.000000000000000000 ) ) ;
#24120=CARTESIAN_POINT ( 'NONE',  ( 36.25628400652970384, 53.06077264917335867, -10.00000000000000000 ) ) ;
#24123=VECTOR ( 'NONE', #67270, 1000.000000000000114 ) ;
#24128=ORIENTED_EDGE ( 'NONE', *, *, #9839, .T. ) ;
#24137=VERTEX_POINT ( 'NONE', #90100 ) ;
#24144=LINE ( 'NONE', #7955, #35535 ) ;
#24149=EDGE_LOOP ( 'NONE', ( #77602, #65354, #15268, #67250 ) ) ;
#24154=CARTESIAN_POINT ( 'NONE',  ( 32.46731799634992655, 102.8122225124608633, 59.99999999999999289 ) ) ;
#24165=ORIENTED_EDGE ( 'NONE', *, *, #73883, .T. ) ;
#24170=CARTESIAN_POINT ( 'NONE',  ( 30.09478592234441408, 78.87673185299470902, 59.99999999999999289 ) ) ;
#24171=ADVANCED_FACE ( 'NONE', ( #36348 ), #99167, .T. ) ;
#24176=ORIENTED_EDGE ( 'NONE', *, *, #39691, .F. ) ;
#24178=DIRECTION ( 'NONE',  ( 1.000000000000000000, 1.465097884282125932E-13, 0.000000000000000000 ) ) ;
#24186=DIRECTION ( 'NONE',  ( 0.3887219701523905169, 0.9213551052231945260, 0.000000000000000000 ) ) ;
#24191=DIRECTION ( 'NONE',  ( 0.000000000000000000, 0.000000000000000000, 1.000000000000000000 ) ) ;
#24192=EDGE_CURVE ( 'NONE', #41961, #36501, #6944, .T. ) ;
#24194=AXIS2_PLACEMENT_3D ( 'NONE', #85164, #8627, #31413 ) ;
#24198=DIRECTION ( 'NONE',  ( 0.000000000000000000, 0.000000000000000000, -1.000000000000000000 ) ) ;
#24207=VECTOR ( 'NONE', #58149, 1000.000000000000114 ) ;
#24226=DIRECTION ( 'NONE',  ( -0.7845058662180028897, -0.6201213960746241316, 0.000000000000000000 ) ) ;
#24227=CARTESIAN_POINT ( 'NONE',  ( 7.225231395932164347, 28.43104314603599647, 177.5919119679930134 ) ) ;
#24229=CARTESIAN_POINT ( 'NONE',  ( -19.65312891409030271, 93.06504152958497400, 45.00000000000000711 ) ) ;
#24236=ORIENTED_EDGE ( 'NONE', *, *, #93715, .T. ) ;
#24241=ORIENTED_EDGE ( 'NONE', *, *, #91067, .T. ) ;
#24246=PLANE ( 'NONE',  #7824 ) ;
#24252=ADVANCED_FACE ( 'NONE', ( #87530 ), #40822, .F. ) ;
#24256=DIRECTION ( 'NONE',  ( -0.000000000000000000, -0.000000000000000000, -1.000000000000000000 ) ) ;
#24265=LINE ( 'NONE', #78995, #17692 ) ;
#24270=CARTESIAN_POINT ( 'NONE',  ( 19.31801425620940194, 115.5650415295850451, 60.00000000000000000 ) ) ;
#24271=FACE_OUTER_BOUND ( 'NONE', #69584, .T. ) ;
#24273=LINE ( 'NONE', #77487, #8978 ) ;
#24274=ORIENTED_EDGE ( 'NONE', *, *, #50941, .F. ) ;
#24278=CARTESIAN_POINT ( 'NONE',  ( -52.52455383977511616, 97.96304663431351401, -10.00000000000000000 ) ) ;
#24296=ORIENTED_EDGE ( 'NONE', *, *, #84274, .T. ) ;
#24300=EDGE_CURVE ( 'NONE', #63648, #25248, #50437, .T. ) ;
#24301=DIRECTION ( 'NONE',  ( -0.2774202615135436534, 0.9607486656258009683, 0.000000000000000000 ) ) ;
#24306=DIRECTION ( 'NONE',  ( -0.7893155279419928894, -0.6139877827364751406, 0.000000000000000000 ) ) ;
#24316=CARTESIAN_POINT ( 'NONE',  ( 48.05801951159151031, 75.31115804243518141, 177.5919119679930134 ) ) ;
#24320=EDGE_CURVE ( 'NONE', #166, #47151, #27660, .T. ) ;
#24323=FACE_OUTER_BOUND ( 'NONE', #35145, .T. ) ;
#24328=VECTOR ( 'NONE', #53982, 1000.000000000000114 ) ;
#24331=CARTESIAN_POINT ( 'NONE',  ( -0.2492734796364604877, 27.10516647459197515, -10.00000000000000000 ) ) ;
#24333=DIRECTION ( 'NONE',  ( -0.07193265315672570104, 0.9974094913373514615, 0.000000000000000000 ) ) ;
#24339=EDGE_CURVE ( 'NONE', #88734, #68766, #59010, .T. ) ;
#24342=AXIS2_PLACEMENT_3D ( 'NONE', #8603, #95251, #39469 ) ;
#24349=LINE ( 'NONE', #69440, #61370 ) ;
#24362=ORIENTED_EDGE ( 'NONE', *, *, #84952, .F. ) ;
#24365=CARTESIAN_POINT ( 'NONE',  ( 47.32807415326522715, 108.5480133836684900, -10.00000000000000000 ) ) ;
#24377=EDGE_LOOP ( 'NONE', ( #83250, #26653, #88115, #62861 ) ) ;
#24390=CARTESIAN_POINT ( 'NONE',  ( -19.65312891409030271, 93.06504152958497400, 10.00000000000000888 ) ) ;
#24408=EDGE_CURVE ( 'NONE', #33333, #79838, #86384, .T. ) ;
#24421=CIRCLE ( 'NONE', #14722, 70.00000000000001421 ) ;
#24423=ORIENTED_EDGE ( 'NONE', *, *, #55203, .T. ) ;
#24425=CARTESIAN_POINT ( 'NONE',  ( 32.31598214102135103, 82.54078291444118065, 59.99999999999999289 ) ) ;
#24429=ADVANCED_FACE ( 'NONE', ( #55399 ), #46823, .F. ) ;
#24438=DIRECTION ( 'NONE',  ( 0.000000000000000000, 0.000000000000000000, 1.000000000000000000 ) ) ;
#24440=ADVANCED_FACE ( 'NONE', ( #15917 ), #77225, .F. ) ;
#24441=FACE_OUTER_BOUND ( 'NONE', #50304, .T. ) ;
#24443=CARTESIAN_POINT ( 'NONE',  ( -4.170157060006060235, 26.08383846222962177, -10.00000000000000000 ) ) ;
#24474=ORIENTED_EDGE ( 'NONE', *, *, #26705, .F. ) ;
#24479=CARTESIAN_POINT ( 'NONE',  ( -19.65312891409030271, 93.06504152958497400, 177.5919119679930134 ) ) ;
#24483=DIRECTION ( 'NONE',  ( -0.000000000000000000, -0.000000000000000000, -1.000000000000000000 ) ) ;
#24490=CARTESIAN_POINT ( 'NONE',  ( -54.45295541630240166, 33.76759809053437067, -10.00000000000000000 ) ) ;
#24495=ORIENTED_EDGE ( 'NONE', *, *, #91136, .F. ) ;
#24502=LINE ( 'NONE', #54896, #7367 ) ;
#24504=LINE ( 'NONE', #24998, #38015 ) ;
#24506=VERTEX_POINT ( 'NONE', #18443 ) ;
#24509=VERTEX_POINT ( 'NONE', #64026 ) ;
#24511=ORIENTED_EDGE ( 'NONE', *, *, #79150, .T. ) ;
#24519=LINE ( 'NONE', #70108, #78996 ) ;
#24529=CARTESIAN_POINT ( 'NONE',  ( 45.19716250472275476, 70.24742367233086782, -10.00000000000000000 ) ) ;
#24530=CARTESIAN_POINT ( 'NONE',  ( 45.19716250472276187, 70.24742367233086782, -10.00000000000000000 ) ) ;
#24546=ORIENTED_EDGE ( 'NONE', *, *, #90879, .F. ) ;
#24547=DIRECTION ( 'NONE',  ( -0.000000000000000000, -0.000000000000000000, 1.000000000000000000 ) ) ;
#24549=EDGE_CURVE ( 'NONE', #83565, #44311, #88898, .T. ) ;
#24550=CARTESIAN_POINT ( 'NONE',  ( -57.46197106626857476, 34.15416430719361784, 177.5919119679930134 ) ) ;
#24553=LINE ( 'NONE', #64570, #99677 ) ;
#24554=DIRECTION ( 'NONE',  ( 0.000000000000000000, 0.000000000000000000, 1.000000000000000000 ) ) ;
#24573=VERTEX_POINT ( 'NONE', #72660 ) ;
#24577=DIRECTION ( 'NONE',  ( 0.5000000000000012212, -0.8660254037844380415, 0.000000000000000000 ) ) ;
#24586=DIRECTION ( 'NONE',  ( -1.000000000000000000, 4.892646582057217816E-14, 0.000000000000000000 ) ) ;
#24591=AXIS2_PLACEMENT_3D ( 'NONE', #35947, #34945, #66357 ) ;
#24595=VERTEX_POINT ( 'NONE', #33125 ) ;
#24605=AXIS2_PLACEMENT_3D ( 'NONE', #83807, #52856, #78173 ) ;
#24608=EDGE_LOOP ( 'NONE', ( #45041, #87929, #73483, #10983 ) ) ;
#24612=EDGE_LOOP ( 'NONE', ( #70760, #34447, #66251, #63305 ) ) ;
#24618=LINE ( 'NONE', #10433, #75386 ) ;
#24619=ORIENTED_EDGE ( 'NONE', *, *, #10268, .T. ) ;
#24622=ORIENTED_EDGE ( 'NONE', *, *, #29227, .T. ) ;
#24628=ORIENTED_EDGE ( 'NONE', *, *, #51184, .T. ) ;
#24636=ADVANCED_FACE ( 'NONE', ( #95490 ), #17944, .F. ) ;
#24637=FACE_OUTER_BOUND ( 'NONE', #90339, .T. ) ;
#24641=ORIENTED_EDGE ( 'NONE', *, *, #45507, .T. ) ;
#24645=CARTESIAN_POINT ( 'NONE',  ( -29.31672308591111431, 23.47304723416778316, 10.00000000000000000 ) ) ;
#24646=FACE_OUTER_BOUND ( 'NONE', #87543, .T. ) ;
#24657=VERTEX_POINT ( 'NONE', #41206 ) ;
#24662=CARTESIAN_POINT ( 'NONE',  ( -40.42249077443059235, 27.53003111760058630, 10.00000000000000000 ) ) ;
#24666=AXIS2_PLACEMENT_3D ( 'NONE', #89703, #20263, #66842 ) ;
#24667=CARTESIAN_POINT ( 'NONE',  ( 48.87252615048947035, 107.3561085985703016, -10.00000000000000000 ) ) ;
#24671=PLANE ( 'NONE',  #81412 ) ;
#24676=EDGE_CURVE ( 'NONE', #70726, #2112, #90128, .T. ) ;
#24687=DIRECTION ( 'NONE',  ( 0.06415622980647761597, -0.9979398670145503969, 0.000000000000000000 ) ) ;
#24695=DIRECTION ( 'NONE',  ( 0.000000000000000000, 0.000000000000000000, 1.000000000000000000 ) ) ;
#24714=CARTESIAN_POINT ( 'NONE',  ( -50.03504209260853486, 51.19473430114911139, 59.99999999999999289 ) ) ;
#24719=LINE ( 'NONE', #39403, #52287 ) ;
#24728=ORIENTED_EDGE ( 'NONE', *, *, #90732, .F. ) ;
#24730=VERTEX_POINT ( 'NONE', #73147 ) ;
#24744=LINE ( 'NONE', #86608, #2922 ) ;
#24759=VERTEX_POINT ( 'NONE', #50316 ) ;
#24762=ORIENTED_EDGE ( 'NONE', *, *, #50252, .T. ) ;
#24764=VERTEX_POINT ( 'NONE', #29512 ) ;
#24767=CARTESIAN_POINT ( 'NONE',  ( 46.43574122514301195, 74.10519008736565638, 10.00000000000000000 ) ) ;
#24773=VERTEX_POINT ( 'NONE', #4217 ) ;
#24774=ORIENTED_EDGE ( 'NONE', *, *, #53512, .T. ) ;
#24779=CARTESIAN_POINT ( 'NONE',  ( -71.61465314115659453, 63.06504152958490295, 203.6502102582797420 ) ) ;
#24791=CARTESIAN_POINT ( 'NONE',  ( -26.59607535340072104, 23.41021043553327630, -10.00000000000000000 ) ) ;
#24796=DIRECTION ( 'NONE',  ( 0.9576970189910596343, 0.2877784213863818774, 0.000000000000000000 ) ) ;
#24804=CARTESIAN_POINT ( 'NONE',  ( 13.67211979723576931, 32.92651376809308772, -10.00000000000000000 ) ) ;
#24809=FACE_OUTER_BOUND ( 'NONE', #78852, .T. ) ;
#24810=DIRECTION ( 'NONE',  ( 0.000000000000000000, -0.000000000000000000, 1.000000000000000000 ) ) ;
#24839=LINE ( 'NONE', #70965, #77272 ) ;
#24840=CARTESIAN_POINT ( 'NONE',  ( 17.38248943320504836, 35.13769309531819829, 10.00000000000000000 ) ) ;
#24842=FACE_OUTER_BOUND ( 'NONE', #53761, .T. ) ;
#24850=EDGE_CURVE ( 'NONE', #36314, #92132, #83751, .T. ) ;
#24864=ORIENTED_EDGE ( 'NONE', *, *, #92511, .F. ) ;
#24871=CARTESIAN_POINT ( 'NONE',  ( -32.30932376655839988, 25.48519649537502119, -10.00000000000000000 ) ) ;
#24879=VERTEX_POINT ( 'NONE', #70498 ) ;
#24887=ORIENTED_EDGE ( 'NONE', *, *, #41478, .F. ) ;
#24890=AXIS2_PLACEMENT_3D ( 'NONE', #38383, #13126, #36393 ) ;
#24898=VECTOR ( 'NONE', #85987, 1000.000000000000227 ) ;
#24899=CARTESIAN_POINT ( 'NONE',  ( -19.65312891409030271, 93.06504152958497400, 10.00000000000000888 ) ) ;
#24904=DIRECTION ( 'NONE',  ( -0.000000000000000000, 0.000000000000000000, -1.000000000000000000 ) ) ;
#24915=VERTEX_POINT ( 'NONE', #85249 ) ;
#24918=LINE ( 'NONE', #73048, #1499 ) ;
#24933=DIRECTION ( 'NONE',  ( -1.000000000000000000, 0.000000000000000000, 0.000000000000000000 ) ) ;
#24937=VERTEX_POINT ( 'NONE', #94344 ) ;
#24943=DIRECTION ( 'NONE',  ( -0.000000000000000000, 0.000000000000000000, 1.000000000000000000 ) ) ;
#24944=LINE ( 'NONE', #40133, #10311 ) ;
#24945=PLANE ( 'NONE',  #26710 ) ;
#24948=CARTESIAN_POINT ( 'NONE',  ( -62.83817737799399339, 37.97373922903765475, 177.5919119679930134 ) ) ;
#24951=ORIENTED_EDGE ( 'NONE', *, *, #25964, .T. ) ;
#24960=CARTESIAN_POINT ( 'NONE',  ( -19.65312891409030271, 93.06504152958497400, 10.00000000000000888 ) ) ;
#24963=VECTOR ( 'NONE', #64253, 1000.000000000000227 ) ;
#24968=DIRECTION ( 'NONE',  ( 1.000000000000000000, 0.000000000000000000, 0.000000000000000000 ) ) ;
#24972=EDGE_CURVE ( 'NONE', #50442, #17777, #44575, .T. ) ;
#24973=CARTESIAN_POINT ( 'NONE',  ( -52.32156893544651410, 31.15564784356141814, 10.00000000000000000 ) ) ;
#24975=CARTESIAN_POINT ( 'NONE',  ( -38.61298035630893111, 26.97617139035147460, -10.00000000000000000 ) ) ;
#24980=DIRECTION ( 'NONE',  ( -0.8660254037844380415, -0.5000000000000011102, 0.000000000000000000 ) ) ;
#24981=ORIENTED_EDGE ( 'NONE', *, *, #55264, .T. ) ;
#24985=ORIENTED_EDGE ( 'NONE', *, *, #75425, .F. ) ;
#24988=ORIENTED_EDGE ( 'NONE', *, *, #4114, .T. ) ;
#24995=DIRECTION ( 'NONE',  ( -0.8278489937552474531, 0.5609510170580175314, 0.000000000000000000 ) ) ;
#24998=CARTESIAN_POINT ( 'NONE',  ( 9.830230629461709668, 30.95267373526312227, -10.00000000000000000 ) ) ;
#25003=EDGE_CURVE ( 'NONE', #86003, #77450, #89748, .T. ) ;
#25012=DIRECTION ( 'NONE',  ( -1.000000000000000000, 0.000000000000000000, 0.000000000000000000 ) ) ;
#25022=EDGE_CURVE ( 'NONE', #19465, #70901, #98317, .T. ) ;
#25025=FACE_OUTER_BOUND ( 'NONE', #51032, .T. ) ;
#25027=VECTOR ( 'NONE', #26544, 1000.000000000000227 ) ;
#25029=PLANE ( 'NONE',  #83921 ) ;
#25039=EDGE_CURVE ( 'NONE', #48736, #6194, #5106, .T. ) ;
#25046=EDGE_CURVE ( 'NONE', #65825, #96856, #81643, .T. ) ;
#25048=VERTEX_POINT ( 'NONE', #97821 ) ;
#25050=ORIENTED_EDGE ( 'NONE', *, *, #65196, .T. ) ;
#25051=ADVANCED_FACE ( 'NONE', ( #84505 ), #76858, .F. ) ;
#25059=CARTESIAN_POINT ( 'NONE',  ( -19.65312891409030271, 93.06504152958497400, 177.5919119679930134 ) ) ;
#25062=CARTESIAN_POINT ( 'NONE',  ( -3.153128914090298274, 64.48620320469859735, 0.000000000000000000 ) ) ;
#25063=VECTOR ( 'NONE', #100244, 1000.000000000000000 ) ;
#25080=CARTESIAN_POINT ( 'NONE',  ( -4.429217378738782962, 26.01694505731172313, -10.00000000000000000 ) ) ;
#25086=LINE ( 'NONE', #92536, #63661 ) ;
#25102=CYLINDRICAL_SURFACE ( 'NONE', #52983, 70.00000000000002842 ) ;
#25106=CARTESIAN_POINT ( 'NONE',  ( -18.31116180715439512, 22.81812098060338911, 10.00000000000000000 ) ) ;
#25108=ORIENTED_EDGE ( 'NONE', *, *, #97124, .F. ) ;
#25117=ORIENTED_EDGE ( 'NONE', *, *, #47205, .T. ) ;
#25124=EDGE_LOOP ( 'NONE', ( #8412, #17290, #37946, #24762, #72113, #14987 ) ) ;
#25125=CARTESIAN_POINT ( 'NONE',  ( -44.30466402961320682, 27.54938068083718505, 177.5919119679930134 ) ) ;
#25130=CARTESIAN_POINT ( 'NONE',  ( 48.98810889288134263, 89.24608170897542436, -10.00000000000000000 ) ) ;
#25141=ORIENTED_EDGE ( 'NONE', *, *, #92878, .F. ) ;
#25155=DIRECTION ( 'NONE',  ( -0.9756173257765569096, -0.2194785493951510180, 0.000000000000000000 ) ) ;
#25156=ORIENTED_EDGE ( 'NONE', *, *, #57718, .F. ) ;
#25157=CARTESIAN_POINT ( 'NONE',  ( 49.42830306794132866, 81.76213237698443947, 10.00000000000000000 ) ) ;
#25170=EDGE_CURVE ( 'NONE', #53015, #43292, #29980, .T. ) ;
#25188=FACE_OUTER_BOUND ( 'NONE', #60642, .T. ) ;
#25200=CARTESIAN_POINT ( 'NONE',  ( 47.43014843991451102, 113.9519901285712251, -10.00000000000000000 ) ) ;
#25206=VECTOR ( 'NONE', #15145, 1000.000000000000000 ) ;
#25210=ORIENTED_EDGE ( 'NONE', *, *, #51662, .T. ) ;
#25214=LINE ( 'NONE', #93149, #65597 ) ;
#25218=VECTOR ( 'NONE', #74544, 1000.000000000000000 ) ;
#25224=ORIENTED_EDGE ( 'NONE', *, *, #54389, .F. ) ;
#25226=VERTEX_POINT ( 'NONE', #95623 ) ;
#25228=LINE ( 'NONE', #56115, #40089 ) ;
#25236=CARTESIAN_POINT ( 'NONE',  ( -56.29836151245349640, 34.88994676555962116, -10.00000000000000000 ) ) ;
#25241=DIRECTION ( 'NONE',  ( -0.9682419296822714072, -0.2500151307524236532, 0.000000000000000000 ) ) ;
#25245=CIRCLE ( 'NONE', #20422, 0.1418229129680828593 ) ;
#25246=EDGE_CURVE ( 'NONE', #43827, #39443, #79906, .T. ) ;
#25247=EDGE_LOOP ( 'NONE', ( #78005, #90715, #46808, #82389 ) ) ;
#25248=VERTEX_POINT ( 'NONE', #26172 ) ;
#25266=ORIENTED_EDGE ( 'NONE', *, *, #47982, .T. ) ;
#25276=EDGE_CURVE ( 'NONE', #73478, #69482, #13857, .T. ) ;
#25280=CIRCLE ( 'NONE', #2664, 0.1418229129681557177 ) ;
#25282=CARTESIAN_POINT ( 'NONE',  ( -19.65312891409030271, 93.06504152958497400, 177.5919119679930134 ) ) ;
#25283=DIRECTION ( 'NONE',  ( -0.7763215174174805666, 0.6303371332823576312, 0.000000000000000000 ) ) ;
#25289=LINE ( 'NONE', #33918, #38202 ) ;
#25291=VECTOR ( 'NONE', #7972, 1000.000000000000000 ) ;
#25303=EDGE_CURVE ( 'NONE', #89390, #1098, #15430, .T. ) ;
#25304=VECTOR ( 'NONE', #76127, 1000.000000000000114 ) ;
#25318=DIRECTION ( 'NONE',  ( 1.000000000000000000, 0.000000000000000000, 0.000000000000000000 ) ) ;
#25330=DIRECTION ( 'NONE',  ( -1.000000000000000000, 0.000000000000000000, 0.000000000000000000 ) ) ;
#25336=CARTESIAN_POINT ( 'NONE',  ( 41.51553799054924099, 59.02985107750643579, 10.00000000000000000 ) ) ;
#25337=CARTESIAN_POINT ( 'NONE',  ( 42.65610334793076674, 64.00004027534475881, 10.00000000000000000 ) ) ;
#25345=DIRECTION ( 'NONE',  ( -0.000000000000000000, -0.000000000000000000, -1.000000000000000000 ) ) ;
#25347=LINE ( 'NONE', #63353, #26168 ) ;
#25354=VECTOR ( 'NONE', #17789, 1000.000000000000000 ) ;
#25359=CARTESIAN_POINT ( 'NONE',  ( -27.62287085492247485, 60.80044415029907867, -10.00000000000000000 ) ) ;
#25364=EDGE_CURVE ( 'NONE', #28623, #31851, #74783, .T. ) ;
#25367=CARTESIAN_POINT ( 'NONE',  ( -21.95578541582649379, 35.16639575222019687, 59.99999999999999289 ) ) ;
#25368=CARTESIAN_POINT ( 'NONE',  ( 46.08672700828314106, 69.01776843458345922, 177.5919119679930134 ) ) ;
#25378=CARTESIAN_POINT ( 'NONE',  ( 41.37327796571900507, 124.7191351846657028, -10.00000000000000000 ) ) ;
#25380=VECTOR ( 'NONE', #14471, 1000.000000000000000 ) ;
#25381=VECTOR ( 'NONE', #9200, 1000.000000000000000 ) ;
#25383=EDGE_LOOP ( 'NONE', ( #25648, #39068, #40306, #36320 ) ) ;
#25392=VECTOR ( 'NONE', #83347, 1000.000000000000227 ) ;
#25406=DIRECTION ( 'NONE',  ( -1.000000000000000000, 0.000000000000000000, 0.000000000000000000 ) ) ;
#25408=ORIENTED_EDGE ( 'NONE', *, *, #69358, .F. ) ;
#25415=ORIENTED_EDGE ( 'NONE', *, *, #51791, .F. ) ;
#25423=DIRECTION ( 'NONE',  ( -0.1963739994383812415, 0.9805290675673896672, 0.000000000000000000 ) ) ;
#25427=VECTOR ( 'NONE', #30430, 1000.000000000000000 ) ;
#25441=VERTEX_POINT ( 'NONE', #39705 ) ;
#25448=CIRCLE ( 'NONE', #43231, 45.00000000000000000 ) ;
#25452=DIRECTION ( 'NONE',  ( 0.3668518372888612822, 0.9302793824855987159, 0.000000000000000000 ) ) ;
#25458=ORIENTED_EDGE ( 'NONE', *, *, #40577, .T. ) ;
#25462=AXIS2_PLACEMENT_3D ( 'NONE', #86674, #3051, #95275 ) ;
#25475=CARTESIAN_POINT ( 'NONE',  ( 29.41244916810467203, 42.77587997571678358, 10.00000000000000000 ) ) ;
#25480=DIRECTION ( 'NONE',  ( -0.9957145386939475484, -0.09248003802712848054, 0.000000000000000000 ) ) ;
#25484=VERTEX_POINT ( 'NONE', #16931 ) ;
#25490=ORIENTED_EDGE ( 'NONE', *, *, #5236, .T. ) ;
#25505=ORIENTED_EDGE ( 'NONE', *, *, #211, .T. ) ;
#25508=AXIS2_PLACEMENT_3D ( 'NONE', #91784, #84202, #14748 ) ;
#25512=ORIENTED_EDGE ( 'NONE', *, *, #46857, .T. ) ;
#25518=ORIENTED_EDGE ( 'NONE', *, *, #68711, .T. ) ;
#25527=DIRECTION ( 'NONE',  ( 0.000000000000000000, 0.000000000000000000, 1.000000000000000000 ) ) ;
#25530=VECTOR ( 'NONE', #15014, 1000.000000000000000 ) ;
#25537=ORIENTED_EDGE ( 'NONE', *, *, #47229, .F. ) ;
#25539=ORIENTED_EDGE ( 'NONE', *, *, #19700, .T. ) ;
#25549=VECTOR ( 'NONE', #27072, 1000.000000000000000 ) ;
#25551=LINE ( 'NONE', #34154, #17608 ) ;
#25564=EDGE_CURVE ( 'NONE', #100252, #30838, #48857, .T. ) ;
#25579=AXIS2_PLACEMENT_3D ( 'NONE', #16824, #39104, #40112 ) ;
#25581=CIRCLE ( 'NONE', #38497, 60.00000000000002132 ) ;
#25589=DIRECTION ( 'NONE',  ( 1.000000000000000000, 1.962715704248044129E-13, 0.000000000000000000 ) ) ;
#25591=ORIENTED_EDGE ( 'NONE', *, *, #55712, .T. ) ;
#25592=VECTOR ( 'NONE', #60066, 1000.000000000000000 ) ;
#25593=CARTESIAN_POINT ( 'NONE',  ( -21.58168810074490551, 24.33735145887881757, -10.00000000000000000 ) ) ;
#25599=LINE ( 'NONE', #54981, #51680 ) ;
#25612=EDGE_CURVE ( 'NONE', #84918, #89501, #79790, .T. ) ;
#25615=DIRECTION ( 'NONE',  ( -0.000000000000000000, 0.000000000000000000, -1.000000000000000000 ) ) ;
#25619=CIRCLE ( 'NONE', #54722, 70.00000000000001421 ) ;
#25623=EDGE_LOOP ( 'NONE', ( #57896, #51189, #6668, #32941 ) ) ;
#25628=VERTEX_POINT ( 'NONE', #4229 ) ;
#25639=ORIENTED_EDGE ( 'NONE', *, *, #11296, .T. ) ;
#25640=EDGE_CURVE ( 'NONE', #59964, #18914, #18963, .T. ) ;
#25648=ORIENTED_EDGE ( 'NONE', *, *, #37624, .T. ) ;
#25653=LINE ( 'NONE', #56534, #72621 ) ;
#25656=PLANE ( 'NONE',  #12939 ) ;
#25663=EDGE_LOOP ( 'NONE', ( #3357, #52186, #89888, #23561 ) ) ;
#25669=CARTESIAN_POINT ( 'NONE',  ( -66.55019942848203129, 42.78701949053055387, 10.00000000000000000 ) ) ;
#25676=ORIENTED_EDGE ( 'NONE', *, *, #81062, .T. ) ;
#25679=EDGE_LOOP ( 'NONE', ( #23869, #36088, #48076, #42930 ) ) ;
#25690=ORIENTED_EDGE ( 'NONE', *, *, #77199, .F. ) ;
#25706=CARTESIAN_POINT ( 'NONE',  ( 49.04287251715432205, 95.72274150194785136, -10.00000000000000000 ) ) ;
#25713=EDGE_CURVE ( 'NONE', #47742, #99040, #10618, .T. ) ;
#25715=DIRECTION ( 'NONE',  ( 1.000000000000000000, 2.149074569095838299E-13, 0.000000000000000000 ) ) ;
#25721=AXIS2_PLACEMENT_3D ( 'NONE', #62017, #31621, #30652 ) ;
#25726=DIRECTION ( 'NONE',  ( 0.000000000000000000, -0.000000000000000000, -1.000000000000000000 ) ) ;
#25728=VECTOR ( 'NONE', #3405, 1000.000000000000114 ) ;
#25736=FACE_OUTER_BOUND ( 'NONE', #5550, .T. ) ;
#25737=VECTOR ( 'NONE', #85524, 1000.000000000000114 ) ;
#25750=ORIENTED_EDGE ( 'NONE', *, *, #73887, .T. ) ;
#25752=FACE_OUTER_BOUND ( 'NONE', #69, .T. ) ;
#25762=CIRCLE ( 'NONE', #53280, 0.1418229129680863287 ) ;
#25776=CARTESIAN_POINT ( 'NONE',  ( -72.30469571560091424, 48.86078274006645472, -10.00000000000000000 ) ) ;
#25781=DIRECTION ( 'NONE',  ( 0.08498217737243618508, 0.9963824715083258177, 0.000000000000000000 ) ) ;
#25791=DIRECTION ( 'NONE',  ( 1.000000000000000000, 0.000000000000000000, 0.000000000000000000 ) ) ;
#25795=DIRECTION ( 'NONE',  ( 0.000000000000000000, -0.000000000000000000, -1.000000000000000000 ) ) ;
#25798=VERTEX_POINT ( 'NONE', #65418 ) ;
#25819=ORIENTED_EDGE ( 'NONE', *, *, #11861, .F. ) ;
#25821=VECTOR ( 'NONE', #100194, 1000.000000000000114 ) ;
#25830=ADVANCED_FACE ( 'NONE', ( #33018 ), #37001, .F. ) ;
#25840=EDGE_CURVE ( 'NONE', #75907, #58283, #44587, .T. ) ;
#25844=ORIENTED_EDGE ( 'NONE', *, *, #32096, .F. ) ;
#25849=LINE ( 'NONE', #17743, #11900 ) ;
#25851=LINE ( 'NONE', #57217, #44863 ) ;
#25857=CARTESIAN_POINT ( 'NONE',  ( 46.30674614090290220, 112.4688969640381231, -10.00000000000000000 ) ) ;
#25860=EDGE_CURVE ( 'NONE', #71283, #8735, #20314, .T. ) ;
#25865=CARTESIAN_POINT ( 'NONE',  ( -7.503431993918264098, 84.28954770299061749, 13.68879844432522219 ) ) ;
#25895=ORIENTED_EDGE ( 'NONE', *, *, #5839, .F. ) ;
#25915=ORIENTED_EDGE ( 'NONE', *, *, #2735, .T. ) ;
#25919=ORIENTED_EDGE ( 'NONE', *, *, #33960, .T. ) ;
#25929=CARTESIAN_POINT ( 'NONE',  ( -19.65312891409030271, 93.06504152958497400, 59.99999999999999289 ) ) ;
#25936=CARTESIAN_POINT ( 'NONE',  ( -45.75347490765857117, 28.11296735934751112, 10.00000000000000000 ) ) ;
#25946=VECTOR ( 'NONE', #45354, 1000.000000000000000 ) ;
#25963=EDGE_LOOP ( 'NONE', ( #50817, #81719, #18063, #84939 ) ) ;
#25964=EDGE_CURVE ( 'NONE', #84967, #31576, #85661, .T. ) ;
#25979=DIRECTION ( 'NONE',  ( -0.000000000000000000, 0.000000000000000000, -1.000000000000000000 ) ) ;
#25986=PLANE ( 'NONE',  #92144 ) ;
#25990=CARTESIAN_POINT ( 'NONE',  ( 46.99867368304095550, 76.19044720721625197, -10.00000000000000000 ) ) ;
#25991=DIRECTION ( 'NONE',  ( 0.5076330711061761702, -0.8615733660689098850, 0.000000000000000000 ) ) ;
#25993=DIRECTION ( 'NONE',  ( -0.9041295198387040433, 0.4272584830711199100, 0.000000000000000000 ) ) ;
#25998=DIRECTION ( 'NONE',  ( -0.7280311630581435267, -0.6855440362341479466, 0.000000000000000000 ) ) ;
#26001=LINE ( 'NONE', #24975, #78704 ) ;
#26007=LINE ( 'NONE', #78707, #96995 ) ;
#26008=VERTEX_POINT ( 'NONE', #16699 ) ;
#26010=CARTESIAN_POINT ( 'NONE',  ( 40.82928596147627331, 60.38352576601455723, 10.00000000000000000 ) ) ;
#26012=VERTEX_POINT ( 'NONE', #55181 ) ;
#26015=ORIENTED_EDGE ( 'NONE', *, *, #99895, .T. ) ;
#26019=ADVANCED_FACE ( 'NONE', ( #55672 ), #79034, .T. ) ;
#26024=CARTESIAN_POINT ( 'NONE',  ( -19.55231060296998180, 93.16478824274193471, 59.99999999999999289 ) ) ;
#26031=ORIENTED_EDGE ( 'NONE', *, *, #81804, .F. ) ;
#26041=EDGE_LOOP ( 'NONE', ( #39544, #36261, #25537, #71489 ) ) ;
#26042=DIRECTION ( 'NONE',  ( 0.000000000000000000, 0.000000000000000000, 1.000000000000000000 ) ) ;
#26047=EDGE_LOOP ( 'NONE', ( #30199, #16062, #68868, #84504 ) ) ;
#26065=VERTEX_POINT ( 'NONE', #24791 ) ;
#26067=ORIENTED_EDGE ( 'NONE', *, *, #70293, .T. ) ;
#26071=CARTESIAN_POINT ( 'NONE',  ( 46.50192534792603283, 74.36443251879779837, 10.00000000000000000 ) ) ;
#26091=ORIENTED_EDGE ( 'NONE', *, *, #31023, .F. ) ;
#26092=VECTOR ( 'NONE', #66740, 1000.000000000000114 ) ;
#26100=CARTESIAN_POINT ( 'NONE',  ( -19.65312891409030271, 93.06504152958497400, -10.00000000000000888 ) ) ;
#26121=LINE ( 'NONE', #96556, #93457 ) ;
#26122=VERTEX_POINT ( 'NONE', #63297 ) ;
#26126=EDGE_LOOP ( 'NONE', ( #97833, #89627, #66610, #53277 ) ) ;
#26127=FACE_OUTER_BOUND ( 'NONE', #42335, .T. ) ;
#26132=DIRECTION ( 'NONE',  ( -0.6386832404231596039, -0.7694697644498922351, 0.000000000000000000 ) ) ;
#26136=ORIENTED_EDGE ( 'NONE', *, *, #86793, .T. ) ;
#26138=ORIENTED_EDGE ( 'NONE', *, *, #37336, .F. ) ;
#26151=CARTESIAN_POINT ( 'NONE',  ( -71.36129514276956343, 45.88172302328153052, 10.00000000000000000 ) ) ;
#26154=ORIENTED_EDGE ( 'NONE', *, *, #98689, .F. ) ;
#26158=CARTESIAN_POINT ( 'NONE',  ( 13.90223112049948639, 33.06302660730329279, 10.00000000000000000 ) ) ;
#26160=CARTESIAN_POINT ( 'NONE',  ( 46.30674614090290220, 112.4688969640381231, -10.00000000000000000 ) ) ;
#26162=CARTESIAN_POINT ( 'NONE',  ( -19.65312891409030271, 93.06504152958497400, 203.6502102582797420 ) ) ;
#26168=VECTOR ( 'NONE', #48668, 1000.000000000000000 ) ;
#26169=CARTESIAN_POINT ( 'NONE',  ( 48.77433535142598231, 99.76555324011610537, 10.00000000000000000 ) ) ;
#26172=CARTESIAN_POINT ( 'NONE',  ( 32.30839531297598910, 123.0650415295850593, 40.00000000000000711 ) ) ;
#26174=ORIENTED_EDGE ( 'NONE', *, *, #65257, .T. ) ;
#26178=LINE ( 'NONE', #81410, #91565 ) ;
#26180=PLANE ( 'NONE',  #67891 ) ;
#26187=ADVANCED_FACE ( 'NONE', ( #41994 ), #78519, .F. ) ;
#26198=EDGE_CURVE ( 'NONE', #77230, #77384, #60688, .T. ) ;
#26204=EDGE_CURVE ( 'NONE', #43030, #6693, #88662, .T. ) ;
#26206=CARTESIAN_POINT ( 'NONE',  ( 50.13870555935886841, 87.67061469898740711, -10.00000000000000000 ) ) ;
#26217=DIRECTION ( 'NONE',  ( 0.000000000000000000, 0.000000000000000000, 1.000000000000000000 ) ) ;
#26221=CARTESIAN_POINT ( 'NONE',  ( -75.14068524134967220, 52.46521621197197760, -10.00000000000000000 ) ) ;
#26229=CARTESIAN_POINT ( 'NONE',  ( 41.37327796571899796, 124.7191351846657028, 10.00000000000000000 ) ) ;
#26230=ORIENTED_EDGE ( 'NONE', *, *, #30062, .T. ) ;
#26233=DIRECTION ( 'NONE',  ( 0.000000000000000000, 0.000000000000000000, 1.000000000000000000 ) ) ;
#26239=VERTEX_POINT ( 'NONE', #66299 ) ;
#26241=ORIENTED_EDGE ( 'NONE', *, *, #44193, .F. ) ;
#26245=ORIENTED_EDGE ( 'NONE', *, *, #13041, .T. ) ;
#26247=ORIENTED_EDGE ( 'NONE', *, *, #23835, .F. ) ;
#26264=CARTESIAN_POINT ( 'NONE',  ( 46.80869107419874098, 110.6443039040113092, -10.00000000000000000 ) ) ;
#26269=EDGE_CURVE ( 'NONE', #59430, #3700, #10691, .T. ) ;
#26274=CARTESIAN_POINT ( 'NONE',  ( -74.97640825042664403, 52.25402898078436920, 10.00000000000000000 ) ) ;
#26304=DIRECTION ( 'NONE',  ( -1.000000000000000000, 0.000000000000000000, 0.000000000000000000 ) ) ;
#26306=CYLINDRICAL_SURFACE ( 'NONE', #1272, 70.00000000000002842 ) ;
#26318=EDGE_CURVE ( 'NONE', #62259, #93301, #98209, .T. ) ;
#26336=AXIS2_PLACEMENT_3D ( 'NONE', #40019, #32445, #48138 ) ;
#26337=VECTOR ( 'NONE', #93925, 1000.000000000000000 ) ;
#26345=CARTESIAN_POINT ( 'NONE',  ( 36.76746430747500227, 51.63176190406338151, 177.5919119679930134 ) ) ;
#26350=DIRECTION ( 'NONE',  ( 0.000000000000000000, 0.000000000000000000, 1.000000000000000000 ) ) ;
#26351=DIRECTION ( 'NONE',  ( -1.000000000000000000, 4.892646582057217816E-14, 0.000000000000000000 ) ) ;
#26354=ORIENTED_EDGE ( 'NONE', *, *, #78516, .F. ) ;
#26355=DIRECTION ( 'NONE',  ( -0.9956898167541090583, 0.09274582908232931189, 0.000000000000000000 ) ) ;
#26358=ORIENTED_EDGE ( 'NONE', *, *, #36258, .T. ) ;
#26359=VECTOR ( 'NONE', #56120, 999.9999999999998863 ) ;
#26360=CARTESIAN_POINT ( 'NONE',  ( 37.67364948790085322, 52.89489741671174272, 10.00000000000000000 ) ) ;
#26371=LINE ( 'NONE', #20773, #42372 ) ;
#26380=CARTESIAN_POINT ( 'NONE',  ( 46.30674614090290220, 112.4688969640381231, 10.00000000000000000 ) ) ;
#26389=ADVANCED_FACE ( 'NONE', ( #3998 ), #34884, .F. ) ;
#26390=CARTESIAN_POINT ( 'NONE',  ( -78.71521058394759507, 57.86724000996476747, -10.00000000000000000 ) ) ;
#26403=LINE ( 'NONE', #58281, #12741 ) ;
#26408=CARTESIAN_POINT ( 'NONE',  ( 13.90223112049948639, 33.06302660730329279, 10.00000000000000000 ) ) ;
#26415=VECTOR ( 'NONE', #56571, 1000.000000000000114 ) ;
#26418=LINE ( 'NONE', #18818, #12104 ) ;
#26423=ORIENTED_EDGE ( 'NONE', *, *, #91424, .F. ) ;
#26426=AXIS2_PLACEMENT_3D ( 'NONE', #82085, #89208, #5045 ) ;
#26428=DIRECTION ( 'NONE',  ( -0.3668518372888710521, -0.9302793824855948301, 0.000000000000000000 ) ) ;
#26431=EDGE_LOOP ( 'NONE', ( #8578, #17421, #84231, #59870 ) ) ;
#26440=AXIS2_PLACEMENT_3D ( 'NONE', #88468, #81346, #26609 ) ;
#26442=ADVANCED_FACE ( 'NONE', ( #882 ), #84035, .T. ) ;
#26443=DIRECTION ( 'NONE',  ( -0.5632146860273895550, 0.8263106059122495850, 0.000000000000000000 ) ) ;
#26447=ADVANCED_FACE ( 'NONE', ( #69279 ), #93108, .F. ) ;
#26456=VERTEX_POINT ( 'NONE', #92621 ) ;
#26473=EDGE_CURVE ( 'NONE', #32988, #36501, #85018, .T. ) ;
#26486=CARTESIAN_POINT ( 'NONE',  ( 48.32408078245681793, 82.80331927372955647, -10.00000000000000000 ) ) ;
#26487=DIRECTION ( 'NONE',  ( -0.000000000000000000, 0.000000000000000000, -1.000000000000000000 ) ) ;
#26491=CARTESIAN_POINT ( 'NONE',  ( -78.71521058394759507, 57.86724000996476747, -10.00000000000000000 ) ) ;
#26501=VERTEX_POINT ( 'NONE', #21693 ) ;
#26504=CARTESIAN_POINT ( 'NONE',  ( -19.65312891409030271, 93.06504152958497400, 10.00000000000000888 ) ) ;
#26505=CIRCLE ( 'NONE', #20078, 70.00000000000001421 ) ;
#26510=ORIENTED_EDGE ( 'NONE', *, *, #55574, .T. ) ;
#26511=LINE ( 'NONE', #71622, #71787 ) ;
#26513=AXIS2_PLACEMENT_3D ( 'NONE', #28062, #41388, #79450 ) ;
#26516=EDGE_LOOP ( 'NONE', ( #34947, #28169, #23287, #31908 ) ) ;
#26519=CARTESIAN_POINT ( 'NONE',  ( -19.65312891409030271, 93.06504152958497400, 177.5919119679930134 ) ) ;
#26522=DIRECTION ( 'NONE',  ( 0.4813790724697852297, 0.8765125147926464688, 0.000000000000000000 ) ) ;
#26528=EDGE_CURVE ( 'NONE', #89390, #36862, #52575, .T. ) ;
#26533=CARTESIAN_POINT ( 'NONE',  ( 15.67199189347853761, 32.63213790969698636, 10.00000000000000000 ) ) ;
#26538=ORIENTED_EDGE ( 'NONE', *, *, #12664, .F. ) ;
#26544=DIRECTION ( 'NONE',  ( -0.2805612043866616001, -0.9598361373656993933, 0.000000000000000000 ) ) ;
#26571=VECTOR ( 'NONE', #62547, 1000.000000000000000 ) ;
#26578=ORIENTED_EDGE ( 'NONE', *, *, #30407, .F. ) ;
#26581=LINE ( 'NONE', #34176, #97079 ) ;
#26582=EDGE_CURVE ( 'NONE', #28659, #23610, #81791, .T. ) ;
#26594=DIRECTION ( 'NONE',  ( 1.000000000000000000, 0.000000000000000000, 0.000000000000000000 ) ) ;
#26601=EDGE_LOOP ( 'NONE', ( #62988, #53371, #94476, #88483 ) ) ;
#26609=DIRECTION ( 'NONE',  ( -1.000000000000000000, 0.000000000000000000, 0.000000000000000000 ) ) ;
#26612=DIRECTION ( 'NONE',  ( 0.8660254037844379305, 0.5000000000000011102, 0.000000000000000000 ) ) ;
#26616=VERTEX_POINT ( 'NONE', #50841 ) ;
#26624=ORIENTED_EDGE ( 'NONE', *, *, #94328, .T. ) ;
#26627=VERTEX_POINT ( 'NONE', #32774 ) ;
#26631=ORIENTED_EDGE ( 'NONE', *, *, #45997, .F. ) ;
#26634=ORIENTED_EDGE ( 'NONE', *, *, #70890, .F. ) ;
#26650=CARTESIAN_POINT ( 'NONE',  ( 48.32408078245681793, 82.80331927372955647, 10.00000000000000000 ) ) ;
#26653=ORIENTED_EDGE ( 'NONE', *, *, #88749, .F. ) ;
#26656=DIRECTION ( 'NONE',  ( 0.000000000000000000, 0.000000000000000000, 1.000000000000000000 ) ) ;
#26670=DIRECTION ( 'NONE',  ( 0.3595896960900372696, 0.9331105242498740626, 0.000000000000000000 ) ) ;
#26673=DIRECTION ( 'NONE',  ( -0.3958915996110536906, -0.9182972510888841589, 0.000000000000000000 ) ) ;
#26677=ORIENTED_EDGE ( 'NONE', *, *, #24850, .T. ) ;
#26680=DIRECTION ( 'NONE',  ( 0.000000000000000000, 0.000000000000000000, 1.000000000000000000 ) ) ;
#26681=DIRECTION ( 'NONE',  ( -0.9331105242498700658, 0.3595896960900473172, 0.000000000000000000 ) ) ;
#26683=LINE ( 'NONE', #80433, #80646 ) ;
#26691=DIRECTION ( 'NONE',  ( -0.9888308262251267466, 0.1490422661761856560, 0.000000000000000000 ) ) ;
#26693=EDGE_CURVE ( 'NONE', #54647, #11375, #34892, .T. ) ;
#26695=DIRECTION ( 'NONE',  ( 0.000000000000000000, 0.000000000000000000, 1.000000000000000000 ) ) ;
#26699=DIRECTION ( 'NONE',  ( -0.9689225787001330970, 0.2473641778533918756, 0.000000000000000000 ) ) ;
#26705=EDGE_CURVE ( 'NONE', #37717, #56418, #42728, .T. ) ;
#26707=ADVANCED_FACE ( 'NONE', ( #66055 ), #27572, .F. ) ;
#26710=AXIS2_PLACEMENT_3D ( 'NONE', #40639, #63950, #72072 ) ;
#26714=DIRECTION ( 'NONE',  ( 0.5076330711061762813, -0.8615733660689097739, 0.000000000000000000 ) ) ;
#26717=CARTESIAN_POINT ( 'NONE',  ( -19.65312891409030271, 93.06504152958497400, -10.00000000000000888 ) ) ;
#26723=DIRECTION ( 'NONE',  ( -0.9506327454577400138, -0.3103181967972222788, 0.000000000000000000 ) ) ;
#26731=ORIENTED_EDGE ( 'NONE', *, *, #83987, .F. ) ;
#26737=ORIENTED_EDGE ( 'NONE', *, *, #77236, .F. ) ;
#26739=ORIENTED_EDGE ( 'NONE', *, *, #63363, .T. ) ;
#26742=CARTESIAN_POINT ( 'NONE',  ( 48.83428215874786815, 87.09189275153327969, 10.00000000000000000 ) ) ;
#26746=AXIS2_PLACEMENT_3D ( 'NONE', #88863, #4698, #88357 ) ;
#26753=VERTEX_POINT ( 'NONE', #60417 ) ;
#26765=DIRECTION ( 'NONE',  ( -0.2168075248790319320, -0.9762143704923770260, 0.000000000000000000 ) ) ;
#26769=LINE ( 'NONE', #27768, #80377 ) ;
#26771=EDGE_LOOP ( 'NONE', ( #19058, #37229, #43558, #17827 ) ) ;
#26775=LINE ( 'NONE', #19693, #77048 ) ;
#26784=VERTEX_POINT ( 'NONE', #28537 ) ;
#26786=CARTESIAN_POINT ( 'NONE',  ( -19.65312891409030271, 93.06504152958497400, -10.00000000000000888 ) ) ;
#26795=CARTESIAN_POINT ( 'NONE',  ( 22.45462004596304695, 37.14601545153949047, 10.00000000000000000 ) ) ;
#26796=CARTESIAN_POINT ( 'NONE',  ( -19.65312891409030271, 93.06504152958497400, 177.5919119679930134 ) ) ;
#26801=DIRECTION ( 'NONE',  ( 0.000000000000000000, 0.000000000000000000, 1.000000000000000000 ) ) ;
#26811=EDGE_CURVE ( 'NONE', #29721, #51689, #44227, .T. ) ;
#26819=DIRECTION ( 'NONE',  ( -0.9514785060800255989, 0.3077152132536228324, 0.000000000000000000 ) ) ;
#26832=EDGE_CURVE ( 'NONE', #55869, #70967, #75165, .T. ) ;
#26836=LINE ( 'NONE', #35425, #28566 ) ;
#26837=AXIS2_PLACEMENT_3D ( 'NONE', #55058, #86041, #54544 ) ;
#26838=AXIS2_PLACEMENT_3D ( 'NONE', #56200, #41505, #2537 ) ;
#26840=CARTESIAN_POINT ( 'NONE',  ( 35.03822396736671152, 49.37458582131907292, -10.00000000000000000 ) ) ;
#26843=LINE ( 'NONE', #88697, #40153 ) ;
#26845=AXIS2_PLACEMENT_3D ( 'NONE', #67231, #19667, #98160 ) ;
#26847=DIRECTION ( 'NONE',  ( -0.4554470513245823526, -0.8902628732232651387, 0.000000000000000000 ) ) ;
#26851=CARTESIAN_POINT ( 'NONE',  ( -10.52443098933919785, 85.48226290750096723, 14.42878460834265120 ) ) ;
#26862=ORIENTED_EDGE ( 'NONE', *, *, #97469, .F. ) ;
#26868=ORIENTED_EDGE ( 'NONE', *, *, #73876, .F. ) ;
#26872=LINE ( 'NONE', #49658, #43120 ) ;
#26877=LINE ( 'NONE', #26380, #63725 ) ;
#26879=ORIENTED_EDGE ( 'NONE', *, *, #21399, .T. ) ;
#26886=EDGE_CURVE ( 'NONE', #1592, #45024, #61425, .T. ) ;
#26890=EDGE_CURVE ( 'NONE', #96352, #23472, #92378, .T. ) ;
#26893=EDGE_CURVE ( 'NONE', #89775, #52670, #70527, .T. ) ;
#26895=FACE_BOUND ( 'NONE', #33140, .T. ) ;
#26898=FACE_OUTER_BOUND ( 'NONE', #67472, .T. ) ;
#26918=VECTOR ( 'NONE', #89146, 1000.000000000000114 ) ;
#26922=CIRCLE ( 'NONE', #39748, 60.00000000000002132 ) ;
#26925=FACE_OUTER_BOUND ( 'NONE', #63892, .T. ) ;
#26926=ORIENTED_EDGE ( 'NONE', *, *, #8556, .F. ) ;
#26934=CARTESIAN_POINT ( 'NONE',  ( -19.65312891409030271, 93.06504152958497400, 177.5919119679930134 ) ) ;
#26935=CARTESIAN_POINT ( 'NONE',  ( -19.78992125718828277, 93.02760366756663757, 59.99999999999999289 ) ) ;
#26938=DIRECTION ( 'NONE',  ( 0.02977611660964677234, -0.9995565931350004485, -0.000000000000000000 ) ) ;
#26949=AXIS2_PLACEMENT_3D ( 'NONE', #37848, #90625, #52068 ) ;
#26956=AXIS2_PLACEMENT_3D ( 'NONE', #44463, #75395, #5978 ) ;
#26959=DIRECTION ( 'NONE',  ( 0.000000000000000000, 0.000000000000000000, 1.000000000000000000 ) ) ;
#26987=VERTEX_POINT ( 'NONE', #84122 ) ;
#26989=CARTESIAN_POINT ( 'NONE',  ( 47.39496755818312579, 108.2889530649357681, 10.00000000000000000 ) ) ;
#26990=ORIENTED_EDGE ( 'NONE', *, *, #39507, .T. ) ;
#26998=EDGE_CURVE ( 'NONE', #48579, #20542, #68855, .T. ) ;
#26999=CARTESIAN_POINT ( 'NONE',  ( -19.65312891409030271, 93.06504152958497400, -10.00000000000000888 ) ) ;
#27005=ORIENTED_EDGE ( 'NONE', *, *, #47231, .F. ) ;
#27009=EDGE_CURVE ( 'NONE', #18914, #90330, #53183, .T. ) ;
#27012=ORIENTED_EDGE ( 'NONE', *, *, #33619, .T. ) ;
#27020=EDGE_CURVE ( 'NONE', #34033, #81073, #15671, .T. ) ;
#27024=LINE ( 'NONE', #50305, #75179 ) ;
#27025=VERTEX_POINT ( 'NONE', #7579 ) ;
#27029=DIRECTION ( 'NONE',  ( -0.000000000000000000, -0.000000000000000000, -1.000000000000000000 ) ) ;
#27036=VECTOR ( 'NONE', #48998, 1000.000000000000000 ) ;
#27041=ORIENTED_EDGE ( 'NONE', *, *, #9324, .F. ) ;
#27042=VECTOR ( 'NONE', #42923, 1000.000000000000114 ) ;
#27046=LINE ( 'NONE', #42221, #90053 ) ;
#27052=DIRECTION ( 'NONE',  ( -1.000000000000000000, 0.000000000000000000, 0.000000000000000000 ) ) ;
#27054=PLANE ( 'NONE',  #72677 ) ;
#27055=ADVANCED_FACE ( 'NONE', ( #46565 ), #76017, .F. ) ;
#27065=VECTOR ( 'NONE', #10065, 1000.000000000000114 ) ;
#27071=DIRECTION ( 'NONE',  ( 0.9839629614562466209, -0.1783728972749306640, 0.000000000000000000 ) ) ;
#27072=DIRECTION ( 'NONE',  ( 0.000000000000000000, 0.000000000000000000, 1.000000000000000000 ) ) ;
#27074=VECTOR ( 'NONE', #23438, 1000.000000000000000 ) ;
#27077=VERTEX_POINT ( 'NONE', #37469 ) ;
#27080=EDGE_CURVE ( 'NONE', #38416, #24759, #99304, .T. ) ;
#27107=VECTOR ( 'NONE', #43597, 1000.000000000000114 ) ;
#27111=ORIENTED_EDGE ( 'NONE', *, *, #100167, .F. ) ;
#27123=ADVANCED_FACE ( 'NONE', ( #66280 ), #27287, .F. ) ;
#27130=DIRECTION ( 'NONE',  ( -0.9413434404457866611, 0.3374500364938339270, 0.000000000000000000 ) ) ;
#27134=DIRECTION ( 'NONE',  ( -0.8806841296921844586, 0.4737039832092607705, 0.000000000000000000 ) ) ;
#27142=DIRECTION ( 'NONE',  ( -0.5632146860273895550, 0.8263106059122495850, 0.000000000000000000 ) ) ;
#27145=ORIENTED_EDGE ( 'NONE', *, *, #3015, .T. ) ;
#27155=DIRECTION ( 'NONE',  ( 0.000000000000000000, 0.000000000000000000, 1.000000000000000000 ) ) ;
#27160=ORIENTED_EDGE ( 'NONE', *, *, #95627, .T. ) ;
#27171=VERTEX_POINT ( 'NONE', #89629 ) ;
#27172=CARTESIAN_POINT ( 'NONE',  ( -19.77595115955931249, 92.99413007310096191, 59.99999999999999289 ) ) ;
#27174=VERTEX_POINT ( 'NONE', #34379 ) ;
#27175=CIRCLE ( 'NONE', #78964, 45.00000000000000000 ) ;
#27180=CIRCLE ( 'NONE', #69162, 70.00000000000001421 ) ;
#27182=CARTESIAN_POINT ( 'NONE',  ( 47.22349865033175575, 113.7415181542323097, -10.00000000000000000 ) ) ;
#27185=ORIENTED_EDGE ( 'NONE', *, *, #223, .F. ) ;
#27200=AXIS2_PLACEMENT_3D ( 'NONE', #97403, #83206, #45162 ) ;
#27206=EDGE_CURVE ( 'NONE', #16059, #38622, #88644, .T. ) ;
#27211=CIRCLE ( 'NONE', #72569, 50.00000000000000711 ) ;
#27213=EDGE_CURVE ( 'NONE', #79909, #8078, #66770, .T. ) ;
#27214=ADVANCED_FACE ( 'NONE', ( #5478 ), #18691, .F. ) ;
#27217=DIRECTION ( 'NONE',  ( 0.000000000000000000, 0.000000000000000000, 1.000000000000000000 ) ) ;
#27233=CARTESIAN_POINT ( 'NONE',  ( -52.35448371757384223, 98.99314617336143840, -10.00000000000000000 ) ) ;
#27242=FACE_OUTER_BOUND ( 'NONE', #85339, .T. ) ;
#27245=VERTEX_POINT ( 'NONE', #21675 ) ;
#27246=VECTOR ( 'NONE', #13648, 1000.000000000000000 ) ;
#27249=CARTESIAN_POINT ( 'NONE',  ( 27.87199545867176198, 72.63159553030519078, 59.99999999999999289 ) ) ;
#27251=DIRECTION ( 'NONE',  ( 1.000000000000000000, 0.000000000000000000, 0.000000000000000000 ) ) ;
#27258=ORIENTED_EDGE ( 'NONE', *, *, #88403, .F. ) ;
#27259=CARTESIAN_POINT ( 'NONE',  ( 30.34687108590969373, 93.06504152958497400, -20.00000000000000355 ) ) ;
#27268=LINE ( 'NONE', #88128, #77649 ) ;
#27269=AXIS2_PLACEMENT_3D ( 'NONE', #86566, #17096, #54581 ) ;
#27270=CARTESIAN_POINT ( 'NONE',  ( 10.12303320400422635, 49.19103222140901011, 59.99999999999999289 ) ) ;
#27275=EDGE_CURVE ( 'NONE', #3488, #12952, #21190, .T. ) ;
#27287=PLANE ( 'NONE',  #76980 ) ;
#27288=ORIENTED_EDGE ( 'NONE', *, *, #64821, .F. ) ;
#27289=EDGE_CURVE ( 'NONE', #17528, #36742, #93219, .T. ) ;
#27297=ORIENTED_EDGE ( 'NONE', *, *, #29049, .F. ) ;
#27308=VECTOR ( 'NONE', #37594, 1000.000000000000114 ) ;
#27310=CARTESIAN_POINT ( 'NONE',  ( -63.30067564770008914, 39.94154026010144065, -10.00000000000000000 ) ) ;
#27313=AXIS2_PLACEMENT_3D ( 'NONE', #58225, #19752, #23430 ) ;
#27314=VECTOR ( 'NONE', #18440, 1000.000000000000227 ) ;
#27315=AXIS2_PLACEMENT_3D ( 'NONE', #98023, #28599, #51915 ) ;
#27317=CARTESIAN_POINT ( 'NONE',  ( 47.54560441532652959, 78.55524412553474178, -10.00000000000000000 ) ) ;
#27322=CARTESIAN_POINT ( 'NONE',  ( -19.65312891409030271, 93.06504152958497400, -10.00000000000000888 ) ) ;
#27330=EDGE_CURVE ( 'NONE', #4429, #83781, #44958, .T. ) ;
#27335=VECTOR ( 'NONE', #50844, 1000.000000000000000 ) ;
#27339=CARTESIAN_POINT ( 'NONE',  ( 45.79324619304848909, 117.8999360398438654, -10.00000000000000000 ) ) ;
#27350=ORIENTED_EDGE ( 'NONE', *, *, #18531, .T. ) ;
#27351=CARTESIAN_POINT ( 'NONE',  ( -14.40683470423637580, 84.83712956603842770, 15.00048218900240116 ) ) ;
#27357=DIRECTION ( 'NONE',  ( -0.000000000000000000, -0.000000000000000000, -1.000000000000000000 ) ) ;
#27367=VERTEX_POINT ( 'NONE', #67773 ) ;
#27370=PLANE ( 'NONE',  #77127 ) ;
#27373=CARTESIAN_POINT ( 'NONE',  ( 46.80869107419874098, 110.6443039040113092, 10.00000000000000000 ) ) ;
#27386=CARTESIAN_POINT ( 'NONE',  ( 42.76202708541289610, 64.24573752441608576, -10.00000000000000000 ) ) ;
#27387=EDGE_CURVE ( 'NONE', #26784, #7334, #77372, .T. ) ;
#27395=EDGE_CURVE ( 'NONE', #82333, #57637, #6476, .T. ) ;
#27403=VECTOR ( 'NONE', #16005, 1000.000000000000000 ) ;
#27411=EDGE_CURVE ( 'NONE', #68946, #72634, #98057, .T. ) ;
#27416=VECTOR ( 'NONE', #33580, 1000.000000000000114 ) ;
#27425=CARTESIAN_POINT ( 'NONE',  ( -19.65312891409030271, 93.06504152958497400, -45.00000000000001421 ) ) ;
#27427=EDGE_CURVE ( 'NONE', #78977, #38977, #45941, .T. ) ;
#27431=CARTESIAN_POINT ( 'NONE',  ( 25.88271472100439041, 39.90032630942971537, 177.5919119679930134 ) ) ;
#27432=ORIENTED_EDGE ( 'NONE', *, *, #99971, .F. ) ;
#27436=DIRECTION ( 'NONE',  ( 1.000000000000000000, 0.000000000000000000, 0.000000000000000000 ) ) ;
#27439=DIRECTION ( 'NONE',  ( 0.6778389383370672094, 0.7352104281592295454, 0.000000000000000000 ) ) ;
#27443=EDGE_CURVE ( 'NONE', #79838, #35708, #36866, .T. ) ;
#27453=ORIENTED_EDGE ( 'NONE', *, *, #68021, .T. ) ;
#27461=VECTOR ( 'NONE', #18877, 1000.000000000000000 ) ;
#27467=DIRECTION ( 'NONE',  ( 0.000000000000000000, 0.000000000000000000, 1.000000000000000000 ) ) ;
#27470=ADVANCED_FACE ( 'NONE', ( #61152 ), #6962, .F. ) ;
#27472=EDGE_CURVE ( 'NONE', #75021, #61794, #99680, .T. ) ;
#27475=DIRECTION ( 'NONE',  ( -0.000000000000000000, -0.000000000000000000, -1.000000000000000000 ) ) ;
#27491=VECTOR ( 'NONE', #69787, 1000.000000000000000 ) ;
#27492=DIRECTION ( 'NONE',  ( -0.8756465943326132706, -0.4829524219151361542, 0.000000000000000000 ) ) ;
#27503=ORIENTED_EDGE ( 'NONE', *, *, #80937, .F. ) ;
#27508=EDGE_LOOP ( 'NONE', ( #80006, #51258, #24236, #78729 ) ) ;
#27517=ORIENTED_EDGE ( 'NONE', *, *, #97146, .T. ) ;
#27521=VERTEX_POINT ( 'NONE', #28772 ) ;
#27528=PLANE ( 'NONE',  #71925 ) ;
#27529=EDGE_LOOP ( 'NONE', ( #40979, #1339, #1711, #1666 ) ) ;
#27536=CIRCLE ( 'NONE', #6480, 0.1418229129681522482 ) ;
#27543=CARTESIAN_POINT ( 'NONE',  ( 45.88188149789386472, 72.29567966924399514, -10.00000000000000000 ) ) ;
#27551=EDGE_CURVE ( 'NONE', #28990, #32652, #55539, .T. ) ;
#27557=EDGE_LOOP ( 'NONE', ( #77994, #33716, #38358, #56879 ) ) ;
#27559=LINE ( 'NONE', #58425, #16022 ) ;
#27571=EDGE_LOOP ( 'NONE', ( #46715, #54521, #58489, #90954 ) ) ;
#27572=PLANE ( 'NONE',  #23603 ) ;
#27574=EDGE_CURVE ( 'NONE', #89501, #76706, #17563, .T. ) ;
#27580=EDGE_CURVE ( 'NONE', #89979, #44653, #366, .T. ) ;
#27583=ORIENTED_EDGE ( 'NONE', *, *, #75842, .T. ) ;
#27591=DIRECTION ( 'NONE',  ( -0.9708212084269268738, 0.2398044646550214765, 0.000000000000000000 ) ) ;
#27597=ORIENTED_EDGE ( 'NONE', *, *, #51710, .T. ) ;
#27604=CARTESIAN_POINT ( 'NONE',  ( -78.10577900106846982, 54.55156729251706338, -10.00000000000000000 ) ) ;
#27611=DIRECTION ( 'NONE',  ( -0.9054088711727195093, 0.4245406647209920559, 0.000000000000000000 ) ) ;
#27621=VECTOR ( 'NONE', #69139, 1000.000000000000000 ) ;
#27623=EDGE_LOOP ( 'NONE', ( #15511, #65158, #94261, #71366 ) ) ;
#27625=CARTESIAN_POINT ( 'NONE',  ( 3.854092266844447501, 28.45370138451379560, 10.00000000000000000 ) ) ;
#27627=CARTESIAN_POINT ( 'NONE',  ( 13.67211979723576931, 32.92651376809308772, -10.00000000000000000 ) ) ;
#27641=DIRECTION ( 'NONE',  ( 0.000000000000000000, 0.000000000000000000, 1.000000000000000000 ) ) ;
#27644=VERTEX_POINT ( 'NONE', #67150 ) ;
#27647=CARTESIAN_POINT ( 'NONE',  ( 24.55112987542764458, 40.41347472807389352, -10.00000000000000000 ) ) ;
#27649=LINE ( 'NONE', #51933, #12048 ) ;
#27653=CARTESIAN_POINT ( 'NONE',  ( -76.99869489832862257, 52.47050021824117749, -10.00000000000000000 ) ) ;
#27659=ORIENTED_EDGE ( 'NONE', *, *, #54391, .F. ) ;
#27660=LINE ( 'NONE', #90982, #54407 ) ;
#27681=DIRECTION ( 'NONE',  ( 1.000000000000000000, 1.784287003861858500E-15, 0.000000000000000000 ) ) ;
#27682=DIRECTION ( 'NONE',  ( -0.8450603975019853609, 0.5346708562973920831, 0.000000000000000000 ) ) ;
#27684=DIRECTION ( 'NONE',  ( -0.9331105242498700658, 0.3595896960900473172, 0.000000000000000000 ) ) ;
#27695=CIRCLE ( 'NONE', #87562, 70.00000000000001421 ) ;
#27704=DIRECTION ( 'NONE',  ( 1.000000000000000000, 0.000000000000000000, 0.000000000000000000 ) ) ;
#27708=ADVANCED_FACE ( 'NONE', ( #2261 ), #85910, .F. ) ;
#27722=CARTESIAN_POINT ( 'NONE',  ( 37.37548992677025694, 106.8700141554178913, 59.99999999999999289 ) ) ;
#27723=VERTEX_POINT ( 'NONE', #15420 ) ;
#27726=DIRECTION ( 'NONE',  ( -0.000000000000000000, -0.000000000000000000, -1.000000000000000000 ) ) ;
#27729=EDGE_CURVE ( 'NONE', #70893, #59464, #25280, .T. ) ;
#27730=DIRECTION ( 'NONE',  ( -1.000000000000000000, 0.000000000000000000, 0.000000000000000000 ) ) ;
#27738=LINE ( 'NONE', #59096, #6225 ) ;
#27740=ADVANCED_FACE ( 'NONE', ( #32130 ), #64043, .F. ) ;
#27741=ORIENTED_EDGE ( 'NONE', *, *, #74460, .F. ) ;
#27743=ORIENTED_EDGE ( 'NONE', *, *, #86488, .F. ) ;
#27750=DIRECTION ( 'NONE',  ( -0.8082118706970123911, -0.5888918169447047157, 0.000000000000000000 ) ) ;
#27752=DIRECTION ( 'NONE',  ( 0.000000000000000000, 0.000000000000000000, 1.000000000000000000 ) ) ;
#27754=VECTOR ( 'NONE', #15865, 1000.000000000000000 ) ;
#27768=CARTESIAN_POINT ( 'NONE',  ( 44.18536904650256503, 64.34838820550514527, 177.5919119679930134 ) ) ;
#27783=EDGE_CURVE ( 'NONE', #40696, #15491, #80801, .T. ) ;
#27784=ORIENTED_EDGE ( 'NONE', *, *, #34637, .T. ) ;
#27800=DIRECTION ( 'NONE',  ( 1.000000000000000000, 0.000000000000000000, 0.000000000000000000 ) ) ;
#27812=CARTESIAN_POINT ( 'NONE',  ( -44.26501565779586400, 27.25709555612339230, 10.00000000000000000 ) ) ;
#27817=ORIENTED_EDGE ( 'NONE', *, *, #23575, .T. ) ;
#27831=CARTESIAN_POINT ( 'NONE',  ( -15.18581709147259140, 60.13231987269209355, -10.00000000000000000 ) ) ;
#27836=CARTESIAN_POINT ( 'NONE',  ( 15.67199189347853761, 32.63213790969698636, -10.00000000000000000 ) ) ;
#27844=VERTEX_POINT ( 'NONE', #74161 ) ;
#27847=DIRECTION ( 'NONE',  ( -0.000000000000000000, -0.000000000000000000, -1.000000000000000000 ) ) ;
#27861=FACE_OUTER_BOUND ( 'NONE', #50782, .T. ) ;
#27869=CARTESIAN_POINT ( 'NONE',  ( 8.106622824862185439, 30.17147933776455204, 10.00000000000000000 ) ) ;
#27870=DIRECTION ( 'NONE',  ( -0.000000000000000000, 0.000000000000000000, 1.000000000000000000 ) ) ;
#27877=ORIENTED_EDGE ( 'NONE', *, *, #80048, .F. ) ;
#27879=FACE_BOUND ( 'NONE', #47778, .T. ) ;
#27880=LINE ( 'NONE', #5577, #66069 ) ;
#27888=EDGE_CURVE ( 'NONE', #36836, #85089, #3757, .T. ) ;
#27893=DIRECTION ( 'NONE',  ( -1.000000000000000000, 0.000000000000000000, 0.000000000000000000 ) ) ;
#27898=DIRECTION ( 'NONE',  ( 0.000000000000000000, -0.000000000000000000, 1.000000000000000000 ) ) ;
#27916=CARTESIAN_POINT ( 'NONE',  ( -71.61465314115659453, 63.06504152958490295, 45.00000000000001421 ) ) ;
#27917=VECTOR ( 'NONE', #43934, 1000.000000000000000 ) ;
#27918=DIRECTION ( 'NONE',  ( 0.2639761180675095353, -0.9645292162967424865, 0.000000000000000000 ) ) ;
#27929=ORIENTED_EDGE ( 'NONE', *, *, #62397, .F. ) ;
#27960=CARTESIAN_POINT ( 'NONE',  ( 43.25185672232382217, 62.35734246106903811, 177.5919119679930134 ) ) ;
#27962=CARTESIAN_POINT ( 'NONE',  ( -76.23101443460924997, 54.01191295053621388, -10.00000000000000000 ) ) ;
#27963=LINE ( 'NONE', #20386, #87279 ) ;
#27964=ORIENTED_EDGE ( 'NONE', *, *, #57179, .F. ) ;
#27969=EDGE_LOOP ( 'NONE', ( #15187, #83211, #77055, #82360 ) ) ;
#27980=EDGE_LOOP ( 'NONE', ( #91384, #61472, #12594, #18279 ) ) ;
#27985=CARTESIAN_POINT ( 'NONE',  ( -28.04097607764120781, 24.82386083235215679, 10.00000000000000000 ) ) ;
#27990=ORIENTED_EDGE ( 'NONE', *, *, #7917, .T. ) ;
#27994=ORIENTED_EDGE ( 'NONE', *, *, #95052, .F. ) ;
#27995=EDGE_CURVE ( 'NONE', #55869, #67607, #25289, .T. ) ;
#27999=ORIENTED_EDGE ( 'NONE', *, *, #58548, .F. ) ;
#28000=FACE_OUTER_BOUND ( 'NONE', #12954, .T. ) ;
#28011=EDGE_CURVE ( 'NONE', #2192, #62885, #94881, .T. ) ;
#28019=ORIENTED_EDGE ( 'NONE', *, *, #54249, .F. ) ;
#28028=ORIENTED_EDGE ( 'NONE', *, *, #62275, .F. ) ;
#28053=CARTESIAN_POINT ( 'NONE',  ( -19.75394722521053126, 92.96529481642809856, 59.99999999999999289 ) ) ;
#28057=VECTOR ( 'NONE', #67205, 1000.000000000000000 ) ;
#28062=CARTESIAN_POINT ( 'NONE',  ( -19.65312891409030271, 93.06504152958497400, 10.00000000000000888 ) ) ;
#28069=ORIENTED_EDGE ( 'NONE', *, *, #27574, .F. ) ;
#28073=VECTOR ( 'NONE', #33713, 1000.000000000000000 ) ;
#28080=VECTOR ( 'NONE', #88869, 1000.000000000000000 ) ;
#28086=DIRECTION ( 'NONE',  ( -0.000000000000000000, -0.000000000000000000, -1.000000000000000000 ) ) ;
#28088=PLANE ( 'NONE',  #64496 ) ;
#28092=LINE ( 'NONE', #13411, #87959 ) ;
#28103=DIRECTION ( 'NONE',  ( -0.9662637919863231728, -0.2575544297740022248, 0.000000000000000000 ) ) ;
#28118=EDGE_CURVE ( 'NONE', #68592, #37083, #42473, .T. ) ;
#28121=ORIENTED_EDGE ( 'NONE', *, *, #79077, .F. ) ;
#28123=ORIENTED_EDGE ( 'NONE', *, *, #71694, .T. ) ;
#28124=LINE ( 'NONE', #21053, #65401 ) ;
#28127=EDGE_CURVE ( 'NONE', #8862, #32206, #28279, .T. ) ;
#28134=EDGE_CURVE ( 'NONE', #90765, #32988, #19224, .T. ) ;
#28136=EDGE_LOOP ( 'NONE', ( #53981, #70327, #65719, #50064 ) ) ;
#28137=DIRECTION ( 'NONE',  ( 0.000000000000000000, -0.000000000000000000, 1.000000000000000000 ) ) ;
#28140=LINE ( 'NONE', #90497, #4176 ) ;
#28142=VERTEX_POINT ( 'NONE', #73408 ) ;
#28144=DIRECTION ( 'NONE',  ( 1.000000000000000000, 1.252965984934105094E-13, 0.000000000000000000 ) ) ;
#28151=AXIS2_PLACEMENT_3D ( 'NONE', #50538, #51547, #89604 ) ;
#28152=DIRECTION ( 'NONE',  ( 0.000000000000000000, 0.000000000000000000, 1.000000000000000000 ) ) ;
#28161=LINE ( 'NONE', #4881, #53048 ) ;
#28169=ORIENTED_EDGE ( 'NONE', *, *, #31216, .F. ) ;
#28170=CARTESIAN_POINT ( 'NONE',  ( -41.60683341252619272, 44.79949203189799078, 59.99999999999999289 ) ) ;
#28176=CARTESIAN_POINT ( 'NONE',  ( -9.055497838557604595, 23.87190447404379157, 10.00000000000000000 ) ) ;
#28187=DIRECTION ( 'NONE',  ( 1.000000000000000000, 0.000000000000000000, 0.000000000000000000 ) ) ;
#28194=DIRECTION ( 'NONE',  ( -1.000000000000000000, 0.000000000000000000, 0.000000000000000000 ) ) ;
#28203=ORIENTED_EDGE ( 'NONE', *, *, #62836, .F. ) ;
#28209=ORIENTED_EDGE ( 'NONE', *, *, #96190, .T. ) ;
#28210=ADVANCED_FACE ( 'NONE', ( #50095 ), #92137, .F. ) ;
#28212=LINE ( 'NONE', #52018, #260 ) ;
#28213=AXIS2_PLACEMENT_3D ( 'NONE', #61946, #1178, #70053 ) ;
#28215=CARTESIAN_POINT ( 'NONE',  ( 48.58227110419247907, 77.44677708231240842, 10.00000000000000000 ) ) ;
#28221=ORIENTED_EDGE ( 'NONE', *, *, #59693, .T. ) ;
#28224=ORIENTED_EDGE ( 'NONE', *, *, #100057, .F. ) ;
#28226=AXIS2_PLACEMENT_3D ( 'NONE', #81749, #12323, #43188 ) ;
#28230=DIRECTION ( 'NONE',  ( -1.000000000000000000, 0.000000000000000000, 0.000000000000000000 ) ) ;
#28237=ORIENTED_EDGE ( 'NONE', *, *, #57800, .T. ) ;
#28238=VERTEX_POINT ( 'NONE', #22690 ) ;
#28239=LINE ( 'NONE', #20656, #63808 ) ;
#28244=DIRECTION ( 'NONE',  ( 0.09547062131715937372, -0.9954322480537364237, 0.000000000000000000 ) ) ;
#28245=FACE_OUTER_BOUND ( 'NONE', #79284, .T. ) ;
#28250=ADVANCED_FACE ( 'NONE', ( #67606 ), #19551, .F. ) ;
#28252=VERTEX_POINT ( 'NONE', #98030 ) ;
#28253=DIRECTION ( 'NONE',  ( -0.7845058662180028897, -0.6201213960746241316, 0.000000000000000000 ) ) ;
#28257=ORIENTED_EDGE ( 'NONE', *, *, #78939, .T. ) ;
#28279=LINE ( 'NONE', #36375, #7483 ) ;
#28281=VECTOR ( 'NONE', #49337, 1000.000000000000227 ) ;
#28283=DIRECTION ( 'NONE',  ( -0.9738769792773346312, -0.2270762630343691746, 0.000000000000000000 ) ) ;
#28297=CARTESIAN_POINT ( 'NONE',  ( -19.59711038235854019, 93.19533221515142429, 59.99999999999999289 ) ) ;
#28302=ORIENTED_EDGE ( 'NONE', *, *, #86274, .F. ) ;
#28306=DIRECTION ( 'NONE',  ( -0.8660254037844378194, -0.5000000000000013323, 0.000000000000000000 ) ) ;
#28309=VECTOR ( 'NONE', #21727, 1000.000000000000000 ) ;
#28321=EDGE_CURVE ( 'NONE', #81514, #709, #91628, .T. ) ;
#28323=CARTESIAN_POINT ( 'NONE',  ( -77.58047734835668052, 56.02942318228900120, -10.00000000000000000 ) ) ;
#28325=DIRECTION ( 'NONE',  ( -0.9599109957006544125, -0.2803049773603352168, 0.000000000000000000 ) ) ;
#28333=ORIENTED_EDGE ( 'NONE', *, *, #48161, .F. ) ;
#28343=DIRECTION ( 'NONE',  ( -0.5169068966820336009, 0.8560416229147678191, 0.000000000000000000 ) ) ;
#28346=VERTEX_POINT ( 'NONE', #12434 ) ;
#28353=EDGE_CURVE ( 'NONE', #76243, #8463, #50411, .T. ) ;
#28361=DIRECTION ( 'NONE',  ( 0.000000000000000000, 0.000000000000000000, 1.000000000000000000 ) ) ;
#28362=VECTOR ( 'NONE', #99617, 1000.000000000000000 ) ;
#28365=ORIENTED_EDGE ( 'NONE', *, *, #42972, .T. ) ;
#28368=VERTEX_POINT ( 'NONE', #74249 ) ;
#28375=DIRECTION ( 'NONE',  ( -0.000000000000000000, 0.000000000000000000, 1.000000000000000000 ) ) ;
#28389=EDGE_CURVE ( 'NONE', #68818, #35708, #51410, .T. ) ;
#28401=DIRECTION ( 'NONE',  ( 0.000000000000000000, -0.000000000000000000, 1.000000000000000000 ) ) ;
#28402=CARTESIAN_POINT ( 'NONE',  ( -19.65312891409030271, 93.06504152958497400, 177.5919119679930134 ) ) ;
#28404=DIRECTION ( 'NONE',  ( -1.000000000000000000, 0.000000000000000000, 0.000000000000000000 ) ) ;
#28410=CARTESIAN_POINT ( 'NONE',  ( 3.330649899756923382, 26.67094063374350554, -10.00000000000000000 ) ) ;
#28412=VECTOR ( 'NONE', #78556, 1000.000000000000000 ) ;
#28417=FACE_OUTER_BOUND ( 'NONE', #4258, .T. ) ;
#28418=VECTOR ( 'NONE', #326, 1000.000000000000000 ) ;
#28424=ORIENTED_EDGE ( 'NONE', *, *, #45997, .T. ) ;
#28454=CARTESIAN_POINT ( 'NONE',  ( 46.88368875251780565, 110.3874725885333135, -10.00000000000000000 ) ) ;
#28460=AXIS2_PLACEMENT_3D ( 'NONE', #89172, #4494, #27800 ) ;
#28468=LINE ( 'NONE', #4690, #57917 ) ;
#28469=VECTOR ( 'NONE', #59161, 1000.000000000000000 ) ;
#28472=VERTEX_POINT ( 'NONE', #95467 ) ;
#28473=ORIENTED_EDGE ( 'NONE', *, *, #21602, .F. ) ;
#28480=DIRECTION ( 'NONE',  ( -0.000000000000000000, 0.000000000000000000, -1.000000000000000000 ) ) ;
#28484=VERTEX_POINT ( 'NONE', #33102 ) ;
#28486=AXIS2_PLACEMENT_3D ( 'NONE', #74171, #33667, #41743 ) ;
#28488=ORIENTED_EDGE ( 'NONE', *, *, #45507, .F. ) ;
#28492=DIRECTION ( 'NONE',  ( -0.8718556560469457040, -0.4897629171537489778, 0.000000000000000000 ) ) ;
#28494=VECTOR ( 'NONE', #147, 999.9999999999998863 ) ;
#28495=VERTEX_POINT ( 'NONE', #47783 ) ;
#28497=VERTEX_POINT ( 'NONE', #16892 ) ;
#28501=DIRECTION ( 'NONE',  ( 1.000000000000000000, 1.776356839400250212E-13, 0.000000000000000000 ) ) ;
#28512=DIRECTION ( 'NONE',  ( 0.000000000000000000, 0.000000000000000000, 1.000000000000000000 ) ) ;
#28514=VERTEX_POINT ( 'NONE', #48817 ) ;
#28533=VECTOR ( 'NONE', #5571, 1000.000000000000114 ) ;
#28534=PLANE ( 'NONE',  #91586 ) ;
#28537=CARTESIAN_POINT ( 'NONE',  ( 30.34687108590970794, 93.06504152958497400, 40.00000000000000000 ) ) ;
#28540=AXIS2_PLACEMENT_3D ( 'NONE', #28643, #97579, #20071 ) ;
#28555=AXIS2_PLACEMENT_3D ( 'NONE', #25059, #55935, #48374 ) ;
#28565=ORIENTED_EDGE ( 'NONE', *, *, #15064, .T. ) ;
#28566=VECTOR ( 'NONE', #18742, 1000.000000000000000 ) ;
#28574=CARTESIAN_POINT ( 'NONE',  ( 16.83152549358277739, 56.39007365579823983, 59.99999999999999289 ) ) ;
#28575=DIRECTION ( 'NONE',  ( -0.9576970189910627429, -0.2877784213863714968, 0.000000000000000000 ) ) ;
#28579=ORIENTED_EDGE ( 'NONE', *, *, #720, .T. ) ;
#28582=LINE ( 'NONE', #51895, #13565 ) ;
#28597=EDGE_LOOP ( 'NONE', ( #36715, #64230 ) ) ;
#28599=DIRECTION ( 'NONE',  ( 0.9932214622066130039, -0.1162373735601320568, 0.000000000000000000 ) ) ;
#28605=CARTESIAN_POINT ( 'NONE',  ( -63.34358462235560694, 38.37368864812747660, 177.5919119679930134 ) ) ;
#28607=DIRECTION ( 'NONE',  ( 0.9999986627203610867, -0.001635407438361268905, 0.000000000000000000 ) ) ;
#28614=ORIENTED_EDGE ( 'NONE', *, *, #40477, .T. ) ;
#28615=VERTEX_POINT ( 'NONE', #4191 ) ;
#28618=DIRECTION ( 'NONE',  ( 1.000000000000000000, 0.000000000000000000, 0.000000000000000000 ) ) ;
#28623=VERTEX_POINT ( 'NONE', #35091 ) ;
#28634=VECTOR ( 'NONE', #78654, 1000.000000000000114 ) ;
#28639=EDGE_CURVE ( 'NONE', #43030, #179, #73813, .T. ) ;
#28643=CARTESIAN_POINT ( 'NONE',  ( -19.65312891409030271, 93.06504152958497400, 59.99999999999999289 ) ) ;
#28659=VERTEX_POINT ( 'NONE', #25378 ) ;
#28662=DIRECTION ( 'NONE',  ( -0.1860369090531061309, -0.9825427565607343094, 0.000000000000000000 ) ) ;
#28666=EDGE_CURVE ( 'NONE', #98668, #92719, #70474, .T. ) ;
#28676=CARTESIAN_POINT ( 'NONE',  ( 47.32807415326522715, 108.5480133836684900, 10.00000000000000000 ) ) ;
#28677=AXIS2_PLACEMENT_3D ( 'NONE', #16479, #62559, #23563 ) ;
#28679=VECTOR ( 'NONE', #8033, 1000.000000000000000 ) ;
#28694=LINE ( 'NONE', #13513, #67566 ) ;
#28701=DIRECTION ( 'NONE',  ( -0.000000000000000000, -0.000000000000000000, -1.000000000000000000 ) ) ;
#28707=CARTESIAN_POINT ( 'NONE',  ( 6.117390533544194930, 29.33055864014943026, 10.00000000000000000 ) ) ;
#28711=AXIS2_PLACEMENT_3D ( 'NONE', #2128, #9218, #1122 ) ;
#28718=ORIENTED_EDGE ( 'NONE', *, *, #13269, .F. ) ;
#28727=LINE ( 'NONE', #89580, #52044 ) ;
#28731=ORIENTED_EDGE ( 'NONE', *, *, #42578, .T. ) ;
#28738=CARTESIAN_POINT ( 'NONE',  ( -24.92793671336084671, 23.00358903956173862, -10.00000000000000000 ) ) ;
#28739=DIRECTION ( 'NONE',  ( -1.000000000000000000, 0.000000000000000000, 0.000000000000000000 ) ) ;
#28742=DIRECTION ( 'NONE',  ( -0.000000000000000000, -0.000000000000000000, -1.000000000000000000 ) ) ;
#28743=LINE ( 'NONE', #98667, #15721 ) ;
#28745=ORIENTED_EDGE ( 'NONE', *, *, #51700, .F. ) ;
#28751=DIRECTION ( 'NONE',  ( -0.4055404667435467125, 0.9140770918436946779, 0.000000000000000000 ) ) ;
#28753=VECTOR ( 'NONE', #15068, 1000.000000000000000 ) ;
#28758=ORIENTED_EDGE ( 'NONE', *, *, #4394, .T. ) ;
#28759=CARTESIAN_POINT ( 'NONE',  ( 6.212693912817788267, 48.26412221380545731, 59.99999999999999289 ) ) ;
#28769=DIRECTION ( 'NONE',  ( -0.9302793824855987159, 0.3668518372888613377, 0.000000000000000000 ) ) ;
#28770=VERTEX_POINT ( 'NONE', #27386 ) ;
#28772=CARTESIAN_POINT ( 'NONE',  ( 41.82599275875796963, 62.29945068332010294, -10.00000000000000000 ) ) ;
#28774=EDGE_CURVE ( 'NONE', #30966, #34443, #72245, .T. ) ;
#28781=DIRECTION ( 'NONE',  ( 0.05364311403569549386, 0.9985601716053735810, 0.000000000000000000 ) ) ;
#28795=CIRCLE ( 'NONE', #14192, 70.00000000000001421 ) ;
#28811=EDGE_CURVE ( 'NONE', #64867, #17145, #74991, .T. ) ;
#28813=AXIS2_PLACEMENT_3D ( 'NONE', #10897, #24577, #71712 ) ;
#28823=CIRCLE ( 'NONE', #14290, 70.00000000000001421 ) ;
#28826=CARTESIAN_POINT ( 'NONE',  ( 48.98007068238331385, 88.97864505566217019, -10.00000000000000000 ) ) ;
#28836=EDGE_CURVE ( 'NONE', #28142, #54381, #49578, .T. ) ;
#28837=CARTESIAN_POINT ( 'NONE',  ( 48.95103868752454446, 97.61288834769685252, 10.00000000000000000 ) ) ;
#28838=AXIS2_PLACEMENT_3D ( 'NONE', #6799, #69587, #8300 ) ;
#28844=ORIENTED_EDGE ( 'NONE', *, *, #21881, .T. ) ;
#28846=DIRECTION ( 'NONE',  ( -0.000000000000000000, -0.000000000000000000, -1.000000000000000000 ) ) ;
#28854=CARTESIAN_POINT ( 'NONE',  ( 42.87860686303044844, 124.5258428655388911, 10.00000000000000000 ) ) ;
#28862=VERTEX_POINT ( 'NONE', #60246 ) ;
#28874=CARTESIAN_POINT ( 'NONE',  ( -19.65312891409030271, 93.06504152958497400, 20.00000000000000355 ) ) ;
#28887=FACE_BOUND ( 'NONE', #48527, .T. ) ;
#28896=ORIENTED_EDGE ( 'NONE', *, *, #58915, .F. ) ;
#28900=AXIS2_PLACEMENT_3D ( 'NONE', #18354, #41626, #72568 ) ;
#28901=VERTEX_POINT ( 'NONE', #84608 ) ;
#28908=AXIS2_PLACEMENT_3D ( 'NONE', #32511, #2115, #70496 ) ;
#28912=AXIS2_PLACEMENT_3D ( 'NONE', #1455, #56118, #70843 ) ;
#28914=VERTEX_POINT ( 'NONE', #92703 ) ;
#28917=PLANE ( 'NONE',  #46464 ) ;
#28934=DIRECTION ( 'NONE',  ( -0.9999990636452668058, -0.001368469433204066998, 0.000000000000000000 ) ) ;
#28951=DIRECTION ( 'NONE',  ( 0.000000000000000000, 0.000000000000000000, 1.000000000000000000 ) ) ;
#28952=CARTESIAN_POINT ( 'NONE',  ( -50.44023328799576689, 80.54804368980198603, -10.00000000000000000 ) ) ;
#28961=AXIS2_PLACEMENT_3D ( 'NONE', #67650, #11978, #66657 ) ;
#28981=VECTOR ( 'NONE', #70898, 1000.000000000000000 ) ;
#28982=CARTESIAN_POINT ( 'NONE',  ( -19.65312891409030271, 93.06504152958497400, 177.5919119679930134 ) ) ;
#28990=VERTEX_POINT ( 'NONE', #67876 ) ;
#28994=CARTESIAN_POINT ( 'NONE',  ( -25.89332989531674301, 24.59406508915897760, -10.00000000000000000 ) ) ;
#29001=ADVANCED_FACE ( 'NONE', ( #59758 ), #45553, .F. ) ;
#29005=VECTOR ( 'NONE', #77811, 999.9999999999998863 ) ;
#29032=DIRECTION ( 'NONE',  ( 0.000000000000000000, 0.000000000000000000, 1.000000000000000000 ) ) ;
#29040=EDGE_CURVE ( 'NONE', #56569, #79042, #85275, .T. ) ;
#29044=VERTEX_POINT ( 'NONE', #15651 ) ;
#29049=EDGE_CURVE ( 'NONE', #6804, #40677, #13679, .T. ) ;
#29053=VECTOR ( 'NONE', #62067, 1000.000000000000227 ) ;
#29054=DIRECTION ( 'NONE',  ( -0.5888918169447132644, 0.8082118706970061739, 0.000000000000000000 ) ) ;
#29080=CARTESIAN_POINT ( 'NONE',  ( 5.871984111234073822, 29.22396284167520619, 10.00000000000000000 ) ) ;
#29092=PLANE ( 'NONE',  #31314 ) ;
#29094=CARTESIAN_POINT ( 'NONE',  ( -23.32062891409032090, 78.77562236714182120, 59.99999999999999289 ) ) ;
#29098=ORIENTED_EDGE ( 'NONE', *, *, #75358, .F. ) ;
#29105=ORIENTED_EDGE ( 'NONE', *, *, #14355, .F. ) ;
#29107=DIRECTION ( 'NONE',  ( 0.9505498757754579087, -0.3105719460338643434, 0.000000000000000000 ) ) ;
#29111=CARTESIAN_POINT ( 'NONE',  ( 13.13128053955749408, 45.28703501410428345, 59.99999999999999289 ) ) ;
#29113=CARTESIAN_POINT ( 'NONE',  ( 43.63646518856938172, 66.22046553916848666, -10.00000000000000000 ) ) ;
#29116=ORIENTED_EDGE ( 'NONE', *, *, #19468, .F. ) ;
#29118=ADVANCED_FACE ( 'NONE', ( #24271 ), #39440, .F. ) ;
#29122=VECTOR ( 'NONE', #50433, 1000.000000000000000 ) ;
#29133=ORIENTED_EDGE ( 'NONE', *, *, #97670, .F. ) ;
#29138=LINE ( 'NONE', #12955, #86505 ) ;
#29139=VECTOR ( 'NONE', #88048, 1000.000000000000000 ) ;
#29146=VERTEX_POINT ( 'NONE', #95219 ) ;
#29151=CARTESIAN_POINT ( 'NONE',  ( -19.65312891409030271, 93.06504152958497400, 10.00000000000000888 ) ) ;
#29163=ORIENTED_EDGE ( 'NONE', *, *, #40432, .F. ) ;
#29175=VERTEX_POINT ( 'NONE', #31849 ) ;
#29177=DIRECTION ( 'NONE',  ( -0.8868092729070087277, -0.4621356007560363244, 0.000000000000000000 ) ) ;
#29178=CARTESIAN_POINT ( 'NONE',  ( 38.14196570358561900, 88.90782515902715488, 59.99999999999999289 ) ) ;
#29188=DIRECTION ( 'NONE',  ( -1.000000000000000000, 0.000000000000000000, 0.000000000000000000 ) ) ;
#29190=VECTOR ( 'NONE', #1334, 1000.000000000000227 ) ;
#29197=LINE ( 'NONE', #38253, #1247 ) ;
#29202=CARTESIAN_POINT ( 'NONE',  ( 40.41628377845469089, 57.12529113016345406, 10.00000000000000000 ) ) ;
#29203=CIRCLE ( 'NONE', #84192, 70.00000000000001421 ) ;
#29207=DIRECTION ( 'NONE',  ( 0.000000000000000000, 0.000000000000000000, 1.000000000000000000 ) ) ;
#29214=EDGE_CURVE ( 'NONE', #65497, #37415, #79515, .T. ) ;
#29218=ORIENTED_EDGE ( 'NONE', *, *, #1304, .F. ) ;
#29220=CARTESIAN_POINT ( 'NONE',  ( -19.51336063033015122, 93.04098814110220417, 59.99999999999999289 ) ) ;
#29227=EDGE_CURVE ( 'NONE', #46907, #79781, #80008, .T. ) ;
#29228=CARTESIAN_POINT ( 'NONE',  ( -71.61465314115659453, 63.06504152958490295, -45.00000000000001421 ) ) ;
#29230=ORIENTED_EDGE ( 'NONE', *, *, #35773, .T. ) ;
#29232=ORIENTED_EDGE ( 'NONE', *, *, #85259, .T. ) ;
#29238=ORIENTED_EDGE ( 'NONE', *, *, #91059, .F. ) ;
#29247=CARTESIAN_POINT ( 'NONE',  ( -61.61048871844075592, 38.59675092633816007, -10.00000000000000000 ) ) ;
#29268=VERTEX_POINT ( 'NONE', #94701 ) ;
#29275=CARTESIAN_POINT ( 'NONE',  ( -66.55019942848203129, 42.78701949053055387, -10.00000000000000000 ) ) ;
#29278=AXIS2_PLACEMENT_3D ( 'NONE', #12988, #29654, #91001 ) ;
#29279=VERTEX_POINT ( 'NONE', #49561 ) ;
#29290=PLANE ( 'NONE',  #21985 ) ;
#29291=ORIENTED_EDGE ( 'NONE', *, *, #21595, .F. ) ;
#29301=LINE ( 'NONE', #384, #46905 ) ;
#29302=CARTESIAN_POINT ( 'NONE',  ( -67.83107014231842413, 42.28230845022619633, 177.5919119679930134 ) ) ;
#29307=FACE_OUTER_BOUND ( 'NONE', #94106, .T. ) ;
#29312=DIRECTION ( 'NONE',  ( -0.9963824715083249295, 0.08498217737244645464, 0.000000000000000000 ) ) ;
#29319=CARTESIAN_POINT ( 'NONE',  ( 42.16454434324483458, 125.9067112960471064, 177.5919119679930134 ) ) ;
#29321=CARTESIAN_POINT ( 'NONE',  ( -62.95439910331221256, 68.06504152958493137, -24.99999999999999289 ) ) ;
#29323=EDGE_CURVE ( 'NONE', #5053, #37567, #14077, .T. ) ;
#29328=PLANE ( 'NONE',  #94222 ) ;
#29348=LINE ( 'NONE', #22742, #32136 ) ;
#29356=ORIENTED_EDGE ( 'NONE', *, *, #91935, .F. ) ;
#29361=VERTEX_POINT ( 'NONE', #26533 ) ;
#29365=EDGE_LOOP ( 'NONE', ( #85215, #37453, #73155, #28237 ) ) ;
#29366=ORIENTED_EDGE ( 'NONE', *, *, #59666, .T. ) ;
#29379=DIRECTION ( 'NONE',  ( -0.9999580202055560196, -0.009162850352621043637, 0.000000000000000000 ) ) ;
#29383=ORIENTED_EDGE ( 'NONE', *, *, #25640, .F. ) ;
#29384=EDGE_CURVE ( 'NONE', #8463, #4641, #2743, .T. ) ;
#29385=FACE_BOUND ( 'NONE', #84476, .T. ) ;
#29392=ORIENTED_EDGE ( 'NONE', *, *, #14115, .T. ) ;
#29406=EDGE_CURVE ( 'NONE', #74380, #15461, #68003, .T. ) ;
#29414=CARTESIAN_POINT ( 'NONE',  ( 48.92549481379852949, 97.87922363803308201, 10.00000000000000000 ) ) ;
#29436=CIRCLE ( 'NONE', #8476, 70.00000000000001421 ) ;
#29439=CARTESIAN_POINT ( 'NONE',  ( -18.15312891409030627, 78.77562236714182120, 59.99999999999999289 ) ) ;
#29446=CARTESIAN_POINT ( 'NONE',  ( -71.61465314115659453, 63.06504152958490295, -25.00000000000000000 ) ) ;
#29453=PLANE ( 'NONE',  #17470 ) ;
#29455=EDGE_CURVE ( 'NONE', #87618, #17797, #51819, .T. ) ;
#29459=LINE ( 'NONE', #91290, #56877 ) ;
#29465=DIRECTION ( 'NONE',  ( 0.8080546441192343332, -0.5891075386695858729, 0.000000000000000000 ) ) ;
#29466=DIRECTION ( 'NONE',  ( -1.000000000000000000, 0.000000000000000000, 0.000000000000000000 ) ) ;
#29473=DIRECTION ( 'NONE',  ( -0.1269555777209495084, -0.9919084036772447543, 0.000000000000000000 ) ) ;
#29478=VERTEX_POINT ( 'NONE', #88891 ) ;
#29485=LINE ( 'NONE', #7678, #75939 ) ;
#29490=LINE ( 'NONE', #60366, #49404 ) ;
#29495=CARTESIAN_POINT ( 'NONE',  ( -18.06678529174625325, 77.67718851601459562, 13.60376042076901371 ) ) ;
#29496=LINE ( 'NONE', #35605, #14293 ) ;
#29497=CYLINDRICAL_SURFACE ( 'NONE', #22398, 70.00000000000002842 ) ;
#29500=ORIENTED_EDGE ( 'NONE', *, *, #37989, .F. ) ;
#29504=DIRECTION ( 'NONE',  ( 0.3301025504114332154, 0.9439450758449174916, 0.000000000000000000 ) ) ;
#29512=CARTESIAN_POINT ( 'NONE',  ( -38.35373792487678202, 26.90998726756845727, -10.00000000000000000 ) ) ;
#29514=CARTESIAN_POINT ( 'NONE',  ( -78.57153713424663977, 57.64153020465174393, -10.00000000000000000 ) ) ;
#29515=VECTOR ( 'NONE', #43004, 1000.000000000000000 ) ;
#29517=DIRECTION ( 'NONE',  ( 1.000000000000000000, 0.000000000000000000, 0.000000000000000000 ) ) ;
#29518=CARTESIAN_POINT ( 'NONE',  ( -70.89022602266993545, 47.22876919346843749, -10.00000000000000000 ) ) ;
#29520=CARTESIAN_POINT ( 'NONE',  ( 50.13870555935887552, 87.67061469898740711, 177.5919119679930134 ) ) ;
#29521=EDGE_LOOP ( 'NONE', ( #59503, #582, #42785, #93330 ) ) ;
#29524=EDGE_CURVE ( 'NONE', #45207, #66378, #9726, .T. ) ;
#29532=CARTESIAN_POINT ( 'NONE',  ( 36.10619739613039769, 52.83927550304669296, -10.00000000000000000 ) ) ;
#29537=VECTOR ( 'NONE', #43002, 1000.000000000000114 ) ;
#29546=DIRECTION ( 'NONE',  ( 0.000000000000000000, 0.000000000000000000, 1.000000000000000000 ) ) ;
#29570=ORIENTED_EDGE ( 'NONE', *, *, #49180, .F. ) ;
#29578=DIRECTION ( 'NONE',  ( -0.9756173257765591300, -0.2194785493951409983, 0.000000000000000000 ) ) ;
#29588=EDGE_LOOP ( 'NONE', ( #39074, #15614, #38970, #72391 ) ) ;
#29595=CARTESIAN_POINT ( 'NONE',  ( 35.32845566053276087, 49.32197259295687530, 10.00000000000000000 ) ) ;
#29596=CARTESIAN_POINT ( 'NONE',  ( -49.12564547450223529, 77.70627210468882140, -10.00000000000000000 ) ) ;
#29601=CARTESIAN_POINT ( 'NONE',  ( -19.65312891409030271, 93.06504152958497400, -10.00000000000000888 ) ) ;
#29604=ORIENTED_EDGE ( 'NONE', *, *, #36576, .F. ) ;
#29608=ORIENTED_EDGE ( 'NONE', *, *, #57373, .F. ) ;
#29610=PLANE ( 'NONE',  #15188 ) ;
#29611=AXIS2_PLACEMENT_3D ( 'NONE', #97660, #74857, #68715 ) ;
#29614=ORIENTED_EDGE ( 'NONE', *, *, #50427, .T. ) ;
#29620=VERTEX_POINT ( 'NONE', #17813 ) ;
#29621=ORIENTED_EDGE ( 'NONE', *, *, #75477, .F. ) ;
#29630=CARTESIAN_POINT ( 'NONE',  ( -19.66825484588498085, 93.20605551765035557, 59.99999999999999289 ) ) ;
#29631=CARTESIAN_POINT ( 'NONE',  ( -19.65312891409030271, 93.06504152958497400, 177.5919119679930134 ) ) ;
#29633=CARTESIAN_POINT ( 'NONE',  ( -4.170157060006060235, 26.08383846222962887, -10.00000000000000000 ) ) ;
#29637=ORIENTED_EDGE ( 'NONE', *, *, #30883, .T. ) ;
#29649=ORIENTED_EDGE ( 'NONE', *, *, #18453, .F. ) ;
#29654=DIRECTION ( 'NONE',  ( 0.000000000000000000, 0.000000000000000000, 1.000000000000000000 ) ) ;
#29657=EDGE_CURVE ( 'NONE', #7863, #45522, #79144, .T. ) ;
#29662=ORIENTED_EDGE ( 'NONE', *, *, #63348, .F. ) ;
#29664=DIRECTION ( 'NONE',  ( -0.000000000000000000, -0.000000000000000000, -1.000000000000000000 ) ) ;
#29665=CARTESIAN_POINT ( 'NONE',  ( -19.65312891409030271, 93.06504152958497400, 59.99999999999999289 ) ) ;
#29673=VECTOR ( 'NONE', #37295, 1000.000000000000000 ) ;
#29679=AXIS2_PLACEMENT_3D ( 'NONE', #59945, #85300, #7755 ) ;
#29695=DIRECTION ( 'NONE',  ( 1.000000000000000000, -7.930164461608259453E-16, 0.000000000000000000 ) ) ;
#29696=CARTESIAN_POINT ( 'NONE',  ( 49.93886538132678510, 83.40144735776343055, -10.00000000000000000 ) ) ;
#29706=CARTESIAN_POINT ( 'NONE',  ( 28.35053034700846197, 115.5856344849812274, 59.99999999999999289 ) ) ;
#29710=ADVANCED_FACE ( 'NONE', ( #71021 ), #2618, .F. ) ;
#29714=EDGE_CURVE ( 'NONE', #14275, #91554, #99779, .T. ) ;
#29716=LINE ( 'NONE', #82961, #98008 ) ;
#29721=VERTEX_POINT ( 'NONE', #94337 ) ;
#29734=DIRECTION ( 'NONE',  ( -0.000000000000000000, 0.000000000000000000, 1.000000000000000000 ) ) ;
#29738=ORIENTED_EDGE ( 'NONE', *, *, #78554, .T. ) ;
#29751=AXIS2_PLACEMENT_3D ( 'NONE', #39426, #99764, #15131 ) ;
#29759=ORIENTED_EDGE ( 'NONE', *, *, #54053, .F. ) ;
#29775=DIRECTION ( 'NONE',  ( -0.000000000000000000, 0.000000000000000000, -1.000000000000000000 ) ) ;
#29776=CARTESIAN_POINT ( 'NONE',  ( -19.65312891409030271, 93.06504152958497400, -10.00000000000000888 ) ) ;
#29786=ADVANCED_FACE ( 'NONE', ( #11713 ), #90240, .F. ) ;
#29794=CARTESIAN_POINT ( 'NONE',  ( -53.13161237510370682, 51.94668121853939624, 59.99999999999999289 ) ) ;
#29803=DIRECTION ( 'NONE',  ( -0.000000000000000000, -0.000000000000000000, -1.000000000000000000 ) ) ;
#29804=DIRECTION ( 'NONE',  ( -0.4055404667435369426, 0.9140770918436990078, 0.000000000000000000 ) ) ;
#29806=VECTOR ( 'NONE', #62670, 1000.000000000000000 ) ;
#29811=DIRECTION ( 'NONE',  ( 0.8660254037844379305, 0.5000000000000011102, 0.000000000000000000 ) ) ;
#29826=DIRECTION ( 'NONE',  ( 0.1783728972749415442, 0.9839629614562446225, 0.000000000000000000 ) ) ;
#29834=EDGE_CURVE ( 'NONE', #31605, #1734, #43586, .T. ) ;
#29843=CARTESIAN_POINT ( 'NONE',  ( 44.08135397534552169, 118.8355609772188188, 10.00000000000000000 ) ) ;
#29846=EDGE_LOOP ( 'NONE', ( #40355, #98523, #86147, #56384 ) ) ;
#29853=DIRECTION ( 'NONE',  ( 0.4242989612870595728, -0.9055221650797523614, 0.000000000000000000 ) ) ;
#29858=CARTESIAN_POINT ( 'NONE',  ( -68.10632939235270555, 44.28490124273479012, 10.00000000000000000 ) ) ;
#29862=DIRECTION ( 'NONE',  ( 1.000000000000000000, 0.000000000000000000, 0.000000000000000000 ) ) ;
#29871=FACE_OUTER_BOUND ( 'NONE', #52060, .T. ) ;
#29873=ORIENTED_EDGE ( 'NONE', *, *, #95425, .T. ) ;
#29881=VERTEX_POINT ( 'NONE', #62169 ) ;
#29884=VERTEX_POINT ( 'NONE', #8495 ) ;
#29887=VECTOR ( 'NONE', #6157, 1000.000000000000000 ) ;
#29893=ORIENTED_EDGE ( 'NONE', *, *, #21601, .F. ) ;
#29912=AXIS2_PLACEMENT_3D ( 'NONE', #57610, #80473, #48014 ) ;
#29914=PLANE ( 'NONE',  #67947 ) ;
#29921=CARTESIAN_POINT ( 'NONE',  ( -18.45562326176555956, 23.07528527759725989, 10.00000000000000000 ) ) ;
#29924=PLANE ( 'NONE',  #76005 ) ;
#29925=ORIENTED_EDGE ( 'NONE', *, *, #12935, .F. ) ;
#29935=EDGE_CURVE ( 'NONE', #95983, #6973, #42860, .T. ) ;
#29948=DIRECTION ( 'NONE',  ( -0.03004293549037828290, -0.9995486091367047354, 0.000000000000000000 ) ) ;
#29960=DIRECTION ( 'NONE',  ( -0.3986482622784180418, -0.9171038997749370036, 0.000000000000000000 ) ) ;
#29969=ORIENTED_EDGE ( 'NONE', *, *, #17035, .T. ) ;
#29973=EDGE_LOOP ( 'NONE', ( #17516, #44959, #33866, #39659 ) ) ;
#29980=CIRCLE ( 'NONE', #39652, 70.00000000000001421 ) ;
#29986=DIRECTION ( 'NONE',  ( 0.000000000000000000, 0.000000000000000000, 1.000000000000000000 ) ) ;
#29987=ORIENTED_EDGE ( 'NONE', *, *, #79857, .T. ) ;
#29988=CARTESIAN_POINT ( 'NONE',  ( -17.45610439730315733, 75.77995691783453935, 13.40053368761685704 ) ) ;
#29992=ORIENTED_EDGE ( 'NONE', *, *, #27289, .F. ) ;
#30004=DIRECTION ( 'NONE',  ( -0.9377374661009826307, -0.3473448497826164827, 0.000000000000000000 ) ) ;
#30008=ORIENTED_EDGE ( 'NONE', *, *, #58416, .T. ) ;
#30014=CIRCLE ( 'NONE', #68841, 70.00000000000001421 ) ;
#30018=ORIENTED_EDGE ( 'NONE', *, *, #60232, .T. ) ;
#30019=DIRECTION ( 'NONE',  ( 1.000000000000000000, 0.000000000000000000, 0.000000000000000000 ) ) ;
#30030=DIRECTION ( 'NONE',  ( -0.5369817302126803638, 0.8435938723211520163, 0.000000000000000000 ) ) ;
#30036=EDGE_CURVE ( 'NONE', #26501, #99967, #83677, .T. ) ;
#30037=LINE ( 'NONE', #37626, #74304 ) ;
#30039=LINE ( 'NONE', #22932, #41436 ) ;
#30052=CARTESIAN_POINT ( 'NONE',  ( -52.33464467766007999, 32.58262665401804270, -10.00000000000000000 ) ) ;
#30061=AXIS2_PLACEMENT_3D ( 'NONE', #71392, #70367, #48065 ) ;
#30062=EDGE_CURVE ( 'NONE', #24937, #64281, #3895, .T. ) ;
#30072=FACE_OUTER_BOUND ( 'NONE', #76340, .T. ) ;
#30074=ADVANCED_FACE ( 'NONE', ( #56584 ), #57076, .F. ) ;
#30075=CARTESIAN_POINT ( 'NONE',  ( -58.21247931993242730, 56.66826942632778241, 59.99999999999999289 ) ) ;
#30076=VERTEX_POINT ( 'NONE', #80440 ) ;
#30078=PLANE ( 'NONE',  #1869 ) ;
#30080=PLANE ( 'NONE',  #7871 ) ;
#30084=CARTESIAN_POINT ( 'NONE',  ( -19.79397322353313271, 93.08167340080578356, 59.99999999999999289 ) ) ;
#30086=EDGE_CURVE ( 'NONE', #27367, #95983, #59310, .T. ) ;
#30091=VECTOR ( 'NONE', #6751, 1000.000000000000000 ) ;
#30103=ORIENTED_EDGE ( 'NONE', *, *, #62630, .T. ) ;
#30113=ORIENTED_EDGE ( 'NONE', *, *, #30036, .T. ) ;
#30117=ORIENTED_EDGE ( 'NONE', *, *, #77542, .F. ) ;
#30122=EDGE_CURVE ( 'NONE', #69482, #35722, #34291, .T. ) ;
#30139=ORIENTED_EDGE ( 'NONE', *, *, #25276, .T. ) ;
#30153=ORIENTED_EDGE ( 'NONE', *, *, #5832, .F. ) ;
#30155=FACE_OUTER_BOUND ( 'NONE', #19019, .T. ) ;
#30167=CYLINDRICAL_SURFACE ( 'NONE', #96890, 70.00000000000002842 ) ;
#30168=LINE ( 'NONE', #22571, #78701 ) ;
#30182=DIRECTION ( 'NONE',  ( -0.5104483989331149996, -0.8599083858334093389, 0.000000000000000000 ) ) ;
#30190=FACE_OUTER_BOUND ( 'NONE', #95625, .T. ) ;
#30197=CYLINDRICAL_SURFACE ( 'NONE', #96866, 70.00000000000002842 ) ;
#30199=ORIENTED_EDGE ( 'NONE', *, *, #94964, .T. ) ;
#30202=VECTOR ( 'NONE', #3482, 1000.000000000000000 ) ;
#30208=AXIS2_PLACEMENT_3D ( 'NONE', #12575, #45438, #43452 ) ;
#30210=LINE ( 'NONE', #76805, #43928 ) ;
#30220=ORIENTED_EDGE ( 'NONE', *, *, #58439, .T. ) ;
#30222=CARTESIAN_POINT ( 'NONE',  ( 33.63888670793727442, 47.67824751478842416, 177.5919119679930134 ) ) ;
#30227=DIRECTION ( 'NONE',  ( -0.000000000000000000, 0.000000000000000000, -1.000000000000000000 ) ) ;
#30228=CIRCLE ( 'NONE', #48001, 70.00000000000001421 ) ;
#30237=ORIENTED_EDGE ( 'NONE', *, *, #12607, .T. ) ;
#30250=ORIENTED_EDGE ( 'NONE', *, *, #75038, .T. ) ;
#30251=DIRECTION ( 'NONE',  ( -1.000000000000000000, -4.892646582057367384E-14, 0.000000000000000000 ) ) ;
#30254=ORIENTED_EDGE ( 'NONE', *, *, #9254, .F. ) ;
#30262=VERTEX_POINT ( 'NONE', #760 ) ;
#30263=CARTESIAN_POINT ( 'NONE',  ( 45.80758703142363686, 72.03864405183792030, -10.00000000000000000 ) ) ;
#30272=CARTESIAN_POINT ( 'NONE',  ( -44.74834796241764678, 29.05375577536863929, -10.00000000000000000 ) ) ;
#30282=DIRECTION ( 'NONE',  ( -1.000000000000000000, 0.000000000000000000, 0.000000000000000000 ) ) ;
#30285=CIRCLE ( 'NONE', #7636, 70.00000000000001421 ) ;
#30298=AXIS2_PLACEMENT_3D ( 'NONE', #95381, #73524, #56806 ) ;
#30310=LINE ( 'NONE', #97735, #32086 ) ;
#30326=CARTESIAN_POINT ( 'NONE',  ( -19.15453390681661716, 24.31945705462846163, -10.00000000000000000 ) ) ;
#30332=VERTEX_POINT ( 'NONE', #50358 ) ;
#30336=ORIENTED_EDGE ( 'NONE', *, *, #40477, .F. ) ;
#30342=VECTOR ( 'NONE', #50444, 1000.000000000000000 ) ;
#30345=VECTOR ( 'NONE', #28103, 1000.000000000000114 ) ;
#30351=CARTESIAN_POINT ( 'NONE',  ( -22.23917875008777756, 35.17836123037032792, 59.99999999999999289 ) ) ;
#30353=VERTEX_POINT ( 'NONE', #11397 ) ;
#30365=AXIS2_PLACEMENT_3D ( 'NONE', #21161, #35339, #89596 ) ;
#30370=DIRECTION ( 'NONE',  ( 1.000000000000000000, 0.000000000000000000, 0.000000000000000000 ) ) ;
#30371=ORIENTED_EDGE ( 'NONE', *, *, #13923, .F. ) ;
#30373=ORIENTED_EDGE ( 'NONE', *, *, #69795, .T. ) ;
#30374=ORIENTED_EDGE ( 'NONE', *, *, #31964, .T. ) ;
#30382=ORIENTED_EDGE ( 'NONE', *, *, #49755, .T. ) ;
#30391=FACE_OUTER_BOUND ( 'NONE', #4173, .T. ) ;
#30398=CARTESIAN_POINT ( 'NONE',  ( 45.80758703142363686, 72.03864405183792030, 10.00000000000000000 ) ) ;
#30399=ORIENTED_EDGE ( 'NONE', *, *, #50966, .F. ) ;
#30407=EDGE_CURVE ( 'NONE', #47882, #4221, #45242, .T. ) ;
#30411=VECTOR ( 'NONE', #56318, 1000.000000000000114 ) ;
#30421=VECTOR ( 'NONE', #65797, 1000.000000000000000 ) ;
#30430=DIRECTION ( 'NONE',  ( -0.1963739994383812415, 0.9805290675673896672, 0.000000000000000000 ) ) ;
#30439=VECTOR ( 'NONE', #85474, 1000.000000000000000 ) ;
#30443=DIRECTION ( 'NONE',  ( -0.8278489937552534483, 0.5609510170580086497, 0.000000000000000000 ) ) ;
#30473=AXIS2_PLACEMENT_3D ( 'NONE', #7099, #93234, #23793 ) ;
#30474=CARTESIAN_POINT ( 'NONE',  ( 33.29350273542976879, 95.92556709114796831, 59.99999999999999289 ) ) ;
#30477=ORIENTED_EDGE ( 'NONE', *, *, #52947, .F. ) ;
#30481=AXIS2_PLACEMENT_3D ( 'NONE', #57046, #34261, #65156 ) ;
#30484=AXIS2_PLACEMENT_3D ( 'NONE', #22275, #76970, #38460 ) ;
#30490=CARTESIAN_POINT ( 'NONE',  ( -13.56329049382775231, 72.36584674931148697, 14.11802994067470074 ) ) ;
#30493=DIRECTION ( 'NONE',  ( 0.1266907948509091442, -0.9919422576440851680, 0.000000000000000000 ) ) ;
#30502=DIRECTION ( 'NONE',  ( 0.000000000000000000, 0.000000000000000000, 1.000000000000000000 ) ) ;
#30507=CARTESIAN_POINT ( 'NONE',  ( 42.55121439978241682, 60.39930420098813357, 10.00000000000000000 ) ) ;
#30531=DIRECTION ( 'NONE',  ( -0.9008877160804935613, -0.4340522123146846045, 0.000000000000000000 ) ) ;
#30539=EDGE_CURVE ( 'NONE', #24506, #42773, #64320, .T. ) ;
#30542=EDGE_CURVE ( 'NONE', #62846, #43149, #6043, .T. ) ;
#30546=DIRECTION ( 'NONE',  ( -1.000000000000000000, 0.000000000000000000, 0.000000000000000000 ) ) ;
#30550=AXIS2_PLACEMENT_3D ( 'NONE', #40840, #40346, #79910 ) ;
#30552=ORIENTED_EDGE ( 'NONE', *, *, #67692, .F. ) ;
#30565=CARTESIAN_POINT ( 'NONE',  ( -23.51620074007619010, 60.05598660948531631, -10.00000000000000000 ) ) ;
#30578=ORIENTED_EDGE ( 'NONE', *, *, #97085, .F. ) ;
#30581=DIRECTION ( 'NONE',  ( -0.000000000000000000, -0.000000000000000000, -1.000000000000000000 ) ) ;
#30584=VECTOR ( 'NONE', #28934, 1000.000000000000114 ) ;
#30591=DIRECTION ( 'NONE',  ( -0.000000000000000000, 0.000000000000000000, -1.000000000000000000 ) ) ;
#30599=ORIENTED_EDGE ( 'NONE', *, *, #34639, .T. ) ;
#30601=CARTESIAN_POINT ( 'NONE',  ( 1.638219116881074022, 26.38162155862025671, -10.00000000000000000 ) ) ;
#30605=DIRECTION ( 'NONE',  ( -0.000000000000000000, -0.000000000000000000, -1.000000000000000000 ) ) ;
#30608=CARTESIAN_POINT ( 'NONE',  ( -52.57320609282758994, 32.70376883311633520, 10.00000000000000000 ) ) ;
#30610=ORIENTED_EDGE ( 'NONE', *, *, #96899, .F. ) ;
#30617=EDGE_CURVE ( 'NONE', #46146, #30076, #31295, .T. ) ;
#30625=ORIENTED_EDGE ( 'NONE', *, *, #95425, .F. ) ;
#30636=AXIS2_PLACEMENT_3D ( 'NONE', #51972, #75288, #74309 ) ;
#30637=CARTESIAN_POINT ( 'NONE',  ( 50.33970617970973649, 92.06352491358971690, 10.00000000000000000 ) ) ;
#30648=ORIENTED_EDGE ( 'NONE', *, *, #23073, .F. ) ;
#30652=DIRECTION ( 'NONE',  ( 1.000000000000000000, 0.000000000000000000, 0.000000000000000000 ) ) ;
#30655=EDGE_CURVE ( 'NONE', #73229, #28615, #64711, .T. ) ;
#30656=DIRECTION ( 'NONE',  ( 0.000000000000000000, 0.000000000000000000, -1.000000000000000000 ) ) ;
#30665=VERTEX_POINT ( 'NONE', #29202 ) ;
#30666=DIRECTION ( 'NONE',  ( 1.000000000000000000, 0.000000000000000000, 0.000000000000000000 ) ) ;
#30683=DIRECTION ( 'NONE',  ( -0.000000000000000000, -0.000000000000000000, 1.000000000000000000 ) ) ;
#30690=ORIENTED_EDGE ( 'NONE', *, *, #52570, .T. ) ;
#30702=DIRECTION ( 'NONE',  ( 0.000000000000000000, 0.000000000000000000, 1.000000000000000000 ) ) ;
#30706=ORIENTED_EDGE ( 'NONE', *, *, #69637, .F. ) ;
#30708=DIRECTION ( 'NONE',  ( 0.000000000000000000, 0.000000000000000000, 1.000000000000000000 ) ) ;
#30712=DIRECTION ( 'NONE',  ( -0.000000000000000000, 0.000000000000000000, -1.000000000000000000 ) ) ;
#30716=AXIS2_PLACEMENT_3D ( 'NONE', #61171, #21692, #30282 ) ;
#30721=VERTEX_POINT ( 'NONE', #5403 ) ;
#30723=CARTESIAN_POINT ( 'NONE',  ( -55.59287931351117606, 32.99562883703961091, -10.00000000000000000 ) ) ;
#30731=CARTESIAN_POINT ( 'NONE',  ( 46.88368875251778434, 110.3874725885333135, -10.00000000000000000 ) ) ;
#30736=EDGE_CURVE ( 'NONE', #82113, #3476, #91520, .T. ) ;
#30737=ORIENTED_EDGE ( 'NONE', *, *, #61054, .F. ) ;
#30739=EDGE_CURVE ( 'NONE', #70875, #45464, #82458, .T. ) ;
#30746=DIRECTION ( 'NONE',  ( 0.000000000000000000, 0.000000000000000000, 1.000000000000000000 ) ) ;
#30759=ORIENTED_EDGE ( 'NONE', *, *, #48568, .T. ) ;
#30765=CARTESIAN_POINT ( 'NONE',  ( 33.63407072503001416, 49.62913085183823370, 10.00000000000000000 ) ) ;
#30767=VERTEX_POINT ( 'NONE', #76309 ) ;
#30771=EDGE_CURVE ( 'NONE', #18450, #27245, #91033, .T. ) ;
#30774=ADVANCED_FACE ( 'NONE', ( #21598 ), #75813, .F. ) ;
#30792=VECTOR ( 'NONE', #72428, 1000.000000000000227 ) ;
#30809=EDGE_CURVE ( 'NONE', #55246, #93711, #75312, .T. ) ;
#30810=EDGE_CURVE ( 'NONE', #6582, #51970, #37282, .T. ) ;
#30834=ORIENTED_EDGE ( 'NONE', *, *, #94923, .F. ) ;
#30838=VERTEX_POINT ( 'NONE', #35794 ) ;
#30840=ORIENTED_EDGE ( 'NONE', *, *, #11154, .F. ) ;
#30846=DIRECTION ( 'NONE',  ( -0.000000000000000000, -0.000000000000000000, -1.000000000000000000 ) ) ;
#30850=EDGE_CURVE ( 'NONE', #22043, #94679, #67186, .T. ) ;
#30851=DIRECTION ( 'NONE',  ( -0.6625377181876315191, -0.7490285521785713385, 0.000000000000000000 ) ) ;
#30853=ORIENTED_EDGE ( 'NONE', *, *, #10882, .F. ) ;
#30854=AXIS2_PLACEMENT_3D ( 'NONE', #15250, #84224, #91311 ) ;
#30860=EDGE_CURVE ( 'NONE', #3474, #88681, #6882, .T. ) ;
#30868=EDGE_LOOP ( 'NONE', ( #45675, #97921, #85353, #96788 ) ) ;
#30877=LINE ( 'NONE', #77989, #92012 ) ;
#30882=ORIENTED_EDGE ( 'NONE', *, *, #91423, .T. ) ;
#30883=EDGE_CURVE ( 'NONE', #7334, #71477, #65916, .T. ) ;
#30891=PLANE ( 'NONE',  #7589 ) ;
#30892=VERTEX_POINT ( 'NONE', #44873 ) ;
#30898=CARTESIAN_POINT ( 'NONE',  ( 41.37327796571899796, 124.7191351846657028, 10.00000000000000000 ) ) ;
#30899=VERTEX_POINT ( 'NONE', #7377 ) ;
#30911=CARTESIAN_POINT ( 'NONE',  ( -47.47812815766307182, 47.92838303172833037, 59.99999999999999289 ) ) ;
#30916=CARTESIAN_POINT ( 'NONE',  ( 32.30839531297598910, 123.0650415295850593, 203.6502102582797420 ) ) ;
#30918=AXIS2_PLACEMENT_3D ( 'NONE', #95441, #63970, #94913 ) ;
#30943=DIRECTION ( 'NONE',  ( -0.000000000000000000, -0.000000000000000000, -1.000000000000000000 ) ) ;
#30944=DIRECTION ( 'NONE',  ( -0.000000000000000000, 0.000000000000000000, -1.000000000000000000 ) ) ;
#30947=DIRECTION ( 'NONE',  ( -0.3402761906661169178, -0.9403255362191097477, 0.000000000000000000 ) ) ;
#30949=CARTESIAN_POINT ( 'NONE',  ( 44.28334795397206847, 122.1950543691075808, 10.00000000000000000 ) ) ;
#30956=ORIENTED_EDGE ( 'NONE', *, *, #39468, .T. ) ;
#30962=EDGE_CURVE ( 'NONE', #33084, #47394, #70168, .T. ) ;
#30963=VERTEX_POINT ( 'NONE', #282 ) ;
#30965=DIRECTION ( 'NONE',  ( -0.9879014915521923124, 0.1550826972584425645, 0.000000000000000000 ) ) ;
#30966=VERTEX_POINT ( 'NONE', #62058 ) ;
#30968=DIRECTION ( 'NONE',  ( -0.6681572590663601430, 0.7440200784635646603, 0.000000000000000000 ) ) ;
#30970=CARTESIAN_POINT ( 'NONE',  ( 44.85937643310610667, 116.8208962945185050, -10.00000000000000000 ) ) ;
#30971=EDGE_LOOP ( 'NONE', ( #6031, #70977, #85231, #76588 ) ) ;
#30978=ORIENTED_EDGE ( 'NONE', *, *, #1583, .F. ) ;
#30982=ORIENTED_EDGE ( 'NONE', *, *, #66201, .F. ) ;
#30984=CARTESIAN_POINT ( 'NONE',  ( -9.237615305844807168, 72.36688712545108615, 14.94757194756781793 ) ) ;
#30986=CARTESIAN_POINT ( 'NONE',  ( 30.05588850504797449, 78.74034736131613954, 59.99999999999999289 ) ) ;
#30988=ORIENTED_EDGE ( 'NONE', *, *, #77016, .F. ) ;
#30989=AXIS2_PLACEMENT_3D ( 'NONE', #61825, #83692, #22841 ) ;
#30993=CARTESIAN_POINT ( 'NONE',  ( 37.13585574571499848, 81.55128318896728956, 59.99999999999999289 ) ) ;
#31000=DIRECTION ( 'NONE',  ( 0.000000000000000000, 0.000000000000000000, 1.000000000000000000 ) ) ;
#31008=DIRECTION ( 'NONE',  ( 0.000000000000000000, 0.000000000000000000, 1.000000000000000000 ) ) ;
#31013=ORIENTED_EDGE ( 'NONE', *, *, #95052, .T. ) ;
#31018=DIRECTION ( 'NONE',  ( -0.6139877827364832452, 0.7893155279419866721, 0.000000000000000000 ) ) ;
#31021=DIRECTION ( 'NONE',  ( -1.000000000000000000, 0.000000000000000000, 0.000000000000000000 ) ) ;
#31023=EDGE_CURVE ( 'NONE', #57165, #30262, #95041, .T. ) ;
#31027=CARTESIAN_POINT ( 'NONE',  ( -19.53030666862117215, 93.13595298606905715, 59.99999999999999289 ) ) ;
#31028=LINE ( 'NONE', #23420, #7502 ) ;
#31052=ORIENTED_EDGE ( 'NONE', *, *, #10699, .T. ) ;
#31064=CARTESIAN_POINT ( 'NONE',  ( -19.65312891409030271, 93.06504152958497400, -10.00000000000000888 ) ) ;
#31073=DIRECTION ( 'NONE',  ( 1.000000000000000000, 0.000000000000000000, 0.000000000000000000 ) ) ;
#31074=CARTESIAN_POINT ( 'NONE',  ( 48.92549481379852949, 97.87922363803308201, 10.00000000000000000 ) ) ;
#31076=FACE_BOUND ( 'NONE', #34143, .T. ) ;
#31078=CARTESIAN_POINT ( 'NONE',  ( -42.72532191160158987, 28.29708160126036987, -10.00000000000000000 ) ) ;
#31080=ORIENTED_EDGE ( 'NONE', *, *, #77029, .F. ) ;
#31086=EDGE_CURVE ( 'NONE', #8862, #25798, #69001, .T. ) ;
#31098=ORIENTED_EDGE ( 'NONE', *, *, #13163, .T. ) ;
#31102=ORIENTED_EDGE ( 'NONE', *, *, #95793, .T. ) ;
#31125=LINE ( 'NONE', #52943, #51596 ) ;
#31136=ORIENTED_EDGE ( 'NONE', *, *, #36694, .F. ) ;
#31151=LINE ( 'NONE', #92995, #32379 ) ;
#31152=AXIS2_PLACEMENT_3D ( 'NONE', #66076, #81321, #3788 ) ;
#31160=CIRCLE ( 'NONE', #21498, 70.00000000000001421 ) ;
#31168=EDGE_CURVE ( 'NONE', #42726, #28514, #44580, .T. ) ;
#31175=CARTESIAN_POINT ( 'NONE',  ( -58.02784037451009880, 34.21088073648085981, -10.00000000000000000 ) ) ;
#31176=AXIS2_PLACEMENT_3D ( 'NONE', #86899, #94472, #17434 ) ;
#31181=PLANE ( 'NONE',  #86645 ) ;
#31190=EDGE_CURVE ( 'NONE', #91064, #91993, #5604, .T. ) ;
#31191=ORIENTED_EDGE ( 'NONE', *, *, #55279, .F. ) ;
#31193=LINE ( 'NONE', #2703, #24328 ) ;
#31203=ORIENTED_EDGE ( 'NONE', *, *, #3295, .T. ) ;
#31206=DIRECTION ( 'NONE',  ( -0.5000000000000013323, 0.8660254037844380415, 0.000000000000000000 ) ) ;
#31207=ADVANCED_FACE ( 'NONE', ( #60767 ), #74534, .F. ) ;
#31212=PLANE ( 'NONE',  #75283 ) ;
#31216=EDGE_CURVE ( 'NONE', #6854, #36578, #90759, .T. ) ;
#31232=CARTESIAN_POINT ( 'NONE',  ( 24.69086998626515594, 38.90223361192551010, 177.5919119679930134 ) ) ;
#31242=VECTOR ( 'NONE', #1935, 1000.000000000000114 ) ;
#31260=CARTESIAN_POINT ( 'NONE',  ( -46.74660806181546491, 29.87360136034011049, -10.00000000000000000 ) ) ;
#31269=CARTESIAN_POINT ( 'NONE',  ( -28.04097607764120781, 24.82386083235214969, -10.00000000000000000 ) ) ;
#31270=CARTESIAN_POINT ( 'NONE',  ( 12.89700858264996164, 45.12712377379325801, 59.99999999999999289 ) ) ;
#31280=CARTESIAN_POINT ( 'NONE',  ( 7.454216751344177716, 28.24511763804003195, -10.00000000000000000 ) ) ;
#31284=CARTESIAN_POINT ( 'NONE',  ( -16.14350997085658790, 56.98620320469874656, 0.000000000000000000 ) ) ;
#31293=DIRECTION ( 'NONE',  ( -0.2165469281463391349, 0.9762722099447388446, 0.000000000000000000 ) ) ;
#31295=LINE ( 'NONE', #55579, #33537 ) ;
#31314=AXIS2_PLACEMENT_3D ( 'NONE', #6275, #37170, #68068 ) ;
#31320=ORIENTED_EDGE ( 'NONE', *, *, #61576, .T. ) ;
#31321=VECTOR ( 'NONE', #100120, 1000.000000000000000 ) ;
#31330=VECTOR ( 'NONE', #44618, 1000.000000000000227 ) ;
#31331=ORIENTED_EDGE ( 'NONE', *, *, #8357, .T. ) ;
#31332=DIRECTION ( 'NONE',  ( -0.3766285016932175989, 0.9263643838751153270, 0.000000000000000000 ) ) ;
#31336=CARTESIAN_POINT ( 'NONE',  ( -44.74834796241764678, 29.05375577536864995, -10.00000000000000000 ) ) ;
#31363=EDGE_LOOP ( 'NONE', ( #33776, #10562, #44793, #33425 ) ) ;
#31364=VERTEX_POINT ( 'NONE', #22181 ) ;
#31366=CARTESIAN_POINT ( 'NONE',  ( 7.864685750751951865, 30.05722773587472219, -10.00000000000000000 ) ) ;
#31375=ORIENTED_EDGE ( 'NONE', *, *, #12355, .F. ) ;
#31388=CARTESIAN_POINT ( 'NONE',  ( 43.25185672232382217, 62.35734246106904521, -10.00000000000000000 ) ) ;
#31394=CARTESIAN_POINT ( 'NONE',  ( -75.57215499213535281, 50.95729256953105590, -10.00000000000000000 ) ) ;
#31397=PLANE ( 'NONE',  #73712 ) ;
#31398=ORIENTED_EDGE ( 'NONE', *, *, #80226, .F. ) ;
#31401=CARTESIAN_POINT ( 'NONE',  ( -30.62386769735030256, 61.69365454717127051, -10.00000000000000000 ) ) ;
#31402=DIRECTION ( 'NONE',  ( -0.3473448497826262527, 0.9377374661009790779, 0.000000000000000000 ) ) ;
#31408=CYLINDRICAL_SURFACE ( 'NONE', #87005, 70.00000000000002842 ) ;
#31411=EDGE_CURVE ( 'NONE', #52271, #53961, #35641, .T. ) ;
#31413=DIRECTION ( 'NONE',  ( -0.8903844177683323258, -0.4552093898365321412, 0.000000000000000000 ) ) ;
#31414=ORIENTED_EDGE ( 'NONE', *, *, #33215, .F. ) ;
#31437=FACE_OUTER_BOUND ( 'NONE', #49250, .T. ) ;
#31440=DIRECTION ( 'NONE',  ( -0.9414334852479518956, -0.3371987438498165734, 0.000000000000000000 ) ) ;
#31443=ORIENTED_EDGE ( 'NONE', *, *, #16098, .F. ) ;
#31449=VERTEX_POINT ( 'NONE', #43225 ) ;
#31465=AXIS2_PLACEMENT_3D ( 'NONE', #11832, #4206, #66012 ) ;
#31467=ORIENTED_EDGE ( 'NONE', *, *, #83687, .T. ) ;
#31480=ORIENTED_EDGE ( 'NONE', *, *, #25860, .T. ) ;
#31501=FACE_OUTER_BOUND ( 'NONE', #99416, .T. ) ;
#31513=DIRECTION ( 'NONE',  ( -0.5078630399532131356, -0.8614378286617561109, 0.000000000000000000 ) ) ;
#31517=EDGE_LOOP ( 'NONE', ( #8826, #14343, #40836, #52800 ) ) ;
#31518=DIRECTION ( 'NONE',  ( 0.000000000000000000, -0.000000000000000000, -1.000000000000000000 ) ) ;
#31520=EDGE_CURVE ( 'NONE', #92543, #18551, #78894, .T. ) ;
#31524=CIRCLE ( 'NONE', #39539, 0.1418229129680897982 ) ;
#31526=EDGE_CURVE ( 'NONE', #3615, #92554, #53805, .T. ) ;
#31534=EDGE_CURVE ( 'NONE', #62259, #72718, #48059, .T. ) ;
#31540=FACE_OUTER_BOUND ( 'NONE', #88751, .T. ) ;
#31541=DIRECTION ( 'NONE',  ( 0.000000000000000000, -0.000000000000000000, -1.000000000000000000 ) ) ;
#31569=FACE_OUTER_BOUND ( 'NONE', #8298, .T. ) ;
#31576=VERTEX_POINT ( 'NONE', #85271 ) ;
#31577=PLANE ( 'NONE',  #41841 ) ;
#31583=EDGE_CURVE ( 'NONE', #5590, #39677, #36621, .T. ) ;
#31589=ORIENTED_EDGE ( 'NONE', *, *, #78353, .F. ) ;
#31595=CARTESIAN_POINT ( 'NONE',  ( -10.54235908185773418, 24.92402704602492847, -10.00000000000000000 ) ) ;
#31596=ORIENTED_EDGE ( 'NONE', *, *, #83747, .T. ) ;
#31605=VERTEX_POINT ( 'NONE', #83775 ) ;
#31611=VERTEX_POINT ( 'NONE', #44220 ) ;
#31612=DIRECTION ( 'NONE',  ( -0.9689885751534038638, -0.2471055264905585858, 0.000000000000000000 ) ) ;
#31614=DIRECTION ( 'NONE',  ( 1.000000000000000000, 0.000000000000000000, 0.000000000000000000 ) ) ;
#31621=DIRECTION ( 'NONE',  ( -0.000000000000000000, -0.000000000000000000, -1.000000000000000000 ) ) ;
#31627=CARTESIAN_POINT ( 'NONE',  ( -67.91103796225580425, 44.10201266000169795, -10.00000000000000000 ) ) ;
#31632=ORIENTED_EDGE ( 'NONE', *, *, #73080, .F. ) ;
#31637=AXIS2_PLACEMENT_3D ( 'NONE', #53907, #47317, #85897 ) ;
#31652=AXIS2_PLACEMENT_3D ( 'NONE', #75163, #98958, #14342 ) ;
#31677=ORIENTED_EDGE ( 'NONE', *, *, #50555, .F. ) ;
#31682=CARTESIAN_POINT ( 'NONE',  ( -36.26652983198115976, 26.35523046909639078, -10.00000000000000000 ) ) ;
#31683=LINE ( 'NONE', #14996, #16103 ) ;
#31684=VERTEX_POINT ( 'NONE', #14336 ) ;
#31687=ORIENTED_EDGE ( 'NONE', *, *, #82290, .F. ) ;
#31696=VECTOR ( 'NONE', #37356, 1000.000000000000114 ) ;
#31697=EDGE_CURVE ( 'NONE', #87618, #55881, #46204, .T. ) ;
#31703=LINE ( 'NONE', #8929, #93445 ) ;
#31704=CIRCLE ( 'NONE', #88424, 0.1418229129681557177 ) ;
#31710=ORIENTED_EDGE ( 'NONE', *, *, #80937, .T. ) ;
#31716=DIRECTION ( 'NONE',  ( -0.8098206029991054100, 0.5866775868892259993, 0.000000000000000000 ) ) ;
#31723=VERTEX_POINT ( 'NONE', #22430 ) ;
#31725=EDGE_LOOP ( 'NONE', ( #55884, #16132, #41195, #68854 ) ) ;
#31726=VECTOR ( 'NONE', #74148, 1000.000000000000114 ) ;
#31728=DIRECTION ( 'NONE',  ( -0.3473448497826262527, 0.9377374661009790779, 0.000000000000000000 ) ) ;
#31735=VECTOR ( 'NONE', #84657, 1000.000000000000000 ) ;
#31738=ORIENTED_EDGE ( 'NONE', *, *, #100054, .F. ) ;
#31740=DIRECTION ( 'NONE',  ( -0.8600446134263897147, -0.5102188382608503492, 0.000000000000000000 ) ) ;
#31741=ORIENTED_EDGE ( 'NONE', *, *, #26473, .F. ) ;
#31760=DIRECTION ( 'NONE',  ( -0.3766285016932175433, 0.9263643838751153270, 0.000000000000000000 ) ) ;
#31768=DIRECTION ( 'NONE',  ( 0.000000000000000000, 0.000000000000000000, 1.000000000000000000 ) ) ;
#31775=CARTESIAN_POINT ( 'NONE',  ( -19.65312891409030271, 93.06504152958497400, -10.00000000000000888 ) ) ;
#31782=AXIS2_PLACEMENT_3D ( 'NONE', #18060, #3375, #4345 ) ;
#31783=PLANE ( 'NONE',  #2636 ) ;
#31805=VECTOR ( 'NONE', #10763, 1000.000000000000000 ) ;
#31813=VERTEX_POINT ( 'NONE', #72043 ) ;
#31842=ADVANCED_FACE ( 'NONE', ( #41614 ), #19361, .F. ) ;
#31849=CARTESIAN_POINT ( 'NONE',  ( -77.74869931532474254, 54.01501336371526918, 10.00000000000000000 ) ) ;
#31850=AXIS2_PLACEMENT_3D ( 'NONE', #73795, #18606, #27704 ) ;
#31851=VERTEX_POINT ( 'NONE', #49723 ) ;
#31858=DIRECTION ( 'NONE',  ( -0.000000000000000000, 0.000000000000000000, -1.000000000000000000 ) ) ;
#31865=VERTEX_POINT ( 'NONE', #49239 ) ;
#31870=LINE ( 'NONE', #26169, #75860 ) ;
#31875=ORIENTED_EDGE ( 'NONE', *, *, #46857, .F. ) ;
#31879=PLANE ( 'NONE',  #70705 ) ;
#31899=CARTESIAN_POINT ( 'NONE',  ( -23.29562891409031522, 78.77562236714182120, 59.97499999999998721 ) ) ;
#31903=DIRECTION ( 'NONE',  ( 1.000000000000000000, 0.000000000000000000, 0.000000000000000000 ) ) ;
#31908=ORIENTED_EDGE ( 'NONE', *, *, #92720, .T. ) ;
#31914=VECTOR ( 'NONE', #57587, 1000.000000000000000 ) ;
#31919=AXIS2_PLACEMENT_3D ( 'NONE', #64761, #3473, #32843 ) ;
#31923=VECTOR ( 'NONE', #44722, 1000.000000000000000 ) ;
#31926=CARTESIAN_POINT ( 'NONE',  ( -46.35039662390601478, 28.35603213498495023, 10.00000000000000000 ) ) ;
#31930=CARTESIAN_POINT ( 'NONE',  ( 34.97213163436671124, 51.32435524152969464, -10.00000000000000000 ) ) ;
#31933=PLANE ( 'NONE',  #51530 ) ;
#31941=EDGE_LOOP ( 'NONE', ( #41941, #32863, #97688, #49840 ) ) ;
#31954=ORIENTED_EDGE ( 'NONE', *, *, #21506, .T. ) ;
#31955=AXIS2_PLACEMENT_3D ( 'NONE', #89418, #33160, #72698 ) ;
#31964=EDGE_CURVE ( 'NONE', #26501, #934, #75040, .T. ) ;
#31967=ORIENTED_EDGE ( 'NONE', *, *, #63685, .F. ) ;
#31968=DIRECTION ( 'NONE',  ( -0.000000000000000000, -0.000000000000000000, -1.000000000000000000 ) ) ;
#31969=CARTESIAN_POINT ( 'NONE',  ( -44.30466402961319972, 27.54938068083718861, 10.00000000000000000 ) ) ;
#31970=ORIENTED_EDGE ( 'NONE', *, *, #52881, .F. ) ;
#31976=ADVANCED_FACE ( 'NONE', ( #67411 ), #13719, .T. ) ;
#31979=DIRECTION ( 'NONE',  ( -0.5951734788405994570, 0.8035972437015812542, 0.000000000000000000 ) ) ;
#31984=DIRECTION ( 'NONE',  ( -0.9879014915521923124, 0.1550826972584426755, 0.000000000000000000 ) ) ;
#31998=ORIENTED_EDGE ( 'NONE', *, *, #73932, .F. ) ;
#32016=CARTESIAN_POINT ( 'NONE',  ( 47.32807415326523426, 108.5480133836684900, -10.00000000000000000 ) ) ;
#32020=DIRECTION ( 'NONE',  ( 0.9186857246103528052, -0.3949892902309516951, 0.000000000000000000 ) ) ;
#32035=DIRECTION ( 'NONE',  ( 0.000000000000000000, 0.000000000000000000, 1.000000000000000000 ) ) ;
#32049=AXIS2_PLACEMENT_3D ( 'NONE', #10653, #42520, #34926 ) ;
#32060=EDGE_LOOP ( 'NONE', ( #42901, #59728, #45060, #48022 ) ) ;
#32062=VECTOR ( 'NONE', #77652, 1000.000000000000000 ) ;
#32078=DIRECTION ( 'NONE',  ( -1.000000000000000000, 0.000000000000000000, 0.000000000000000000 ) ) ;
#32081=DIRECTION ( 'NONE',  ( -0.8770933717188679202, -0.4803199113995043623, 0.000000000000000000 ) ) ;
#32083=ORIENTED_EDGE ( 'NONE', *, *, #97182, .F. ) ;
#32086=VECTOR ( 'NONE', #13622, 1000.000000000000000 ) ;
#32091=CARTESIAN_POINT ( 'NONE',  ( 21.51366908625220731, 51.25433263228030967, 59.99999999999999289 ) ) ;
#32095=ORIENTED_EDGE ( 'NONE', *, *, #77797, .T. ) ;
#32096=EDGE_CURVE ( 'NONE', #3586, #55387, #78976, .T. ) ;
#32107=DIRECTION ( 'NONE',  ( -1.000000000000000000, 0.000000000000000000, 0.000000000000000000 ) ) ;
#32118=ORIENTED_EDGE ( 'NONE', *, *, #39399, .T. ) ;
#32122=LINE ( 'NONE', #71665, #87897 ) ;
#32130=FACE_OUTER_BOUND ( 'NONE', #38453, .T. ) ;
#32131=VECTOR ( 'NONE', #37629, 1000.000000000000000 ) ;
#32136=VECTOR ( 'NONE', #13162, 1000.000000000000000 ) ;
#32144=VECTOR ( 'NONE', #48419, 1000.000000000000000 ) ;
#32146=EDGE_LOOP ( 'NONE', ( #73389, #39348, #10914, #43412 ) ) ;
#32152=VECTOR ( 'NONE', #22872, 1000.000000000000000 ) ;
#32158=ORIENTED_EDGE ( 'NONE', *, *, #95638, .T. ) ;
#32162=AXIS2_PLACEMENT_3D ( 'NONE', #9242, #41117, #16337 ) ;
#32174=ORIENTED_EDGE ( 'NONE', *, *, #52940, .T. ) ;
#32203=AXIS2_PLACEMENT_3D ( 'NONE', #10989, #41351, #34754 ) ;
#32206=VERTEX_POINT ( 'NONE', #58680 ) ;
#32209=CARTESIAN_POINT ( 'NONE',  ( -62.46655456400515050, 61.78343361634738073, 59.99999999999999289 ) ) ;
#32211=CIRCLE ( 'NONE', #35398, 70.00000000000001421 ) ;
#32213=CARTESIAN_POINT ( 'NONE',  ( -8.669243101527598583, 25.19333184544593252, 10.00000000000000000 ) ) ;
#32217=CARTESIAN_POINT ( 'NONE',  ( 32.24342178309110096, 47.97677246190462341, -10.00000000000000000 ) ) ;
#32228=VECTOR ( 'NONE', #29775, 1000.000000000000000 ) ;
#32230=ORIENTED_EDGE ( 'NONE', *, *, #55194, .F. ) ;
#32238=LINE ( 'NONE', #62118, #79274 ) ;
#32242=ORIENTED_EDGE ( 'NONE', *, *, #63926, .T. ) ;
#32243=AXIS2_PLACEMENT_3D ( 'NONE', #84924, #55464, #86451 ) ;
#32255=CARTESIAN_POINT ( 'NONE',  ( 33.63407072503001416, 49.62913085183823370, -10.00000000000000000 ) ) ;
#32258=CARTESIAN_POINT ( 'NONE',  ( -6.281727404287059890, 25.63055774385195917, 10.00000000000000000 ) ) ;
#32268=EDGE_LOOP ( 'NONE', ( #80278, #96818, #46591, #33153 ) ) ;
#32287=AXIS2_PLACEMENT_3D ( 'NONE', #42016, #87700, #25318 ) ;
#32299=CIRCLE ( 'NONE', #87348, 70.00000000000001421 ) ;
#32303=DIRECTION ( 'NONE',  ( -0.000000000000000000, -0.000000000000000000, -1.000000000000000000 ) ) ;
#32309=VECTOR ( 'NONE', #19152, 1000.000000000000000 ) ;
#32320=AXIS2_PLACEMENT_3D ( 'NONE', #78030, #79054, #31903 ) ;
#32335=VERTEX_POINT ( 'NONE', #13121 ) ;
#32346=EDGE_CURVE ( 'NONE', #89501, #45207, #14603, .T. ) ;
#32348=PLANE ( 'NONE',  #40027 ) ;
#32354=CARTESIAN_POINT ( 'NONE',  ( -11.40312891409031693, 78.77562236714182120, 59.99999999999999289 ) ) ;
#32359=VECTOR ( 'NONE', #65889, 1000.000000000000000 ) ;
#32362=CARTESIAN_POINT ( 'NONE',  ( -19.65312891409030271, 93.06504152958497400, 20.00000000000000355 ) ) ;
#32364=ORIENTED_EDGE ( 'NONE', *, *, #50394, .T. ) ;
#32367=ORIENTED_EDGE ( 'NONE', *, *, #73883, .F. ) ;
#32369=ORIENTED_EDGE ( 'NONE', *, *, #55279, .T. ) ;
#32379=VECTOR ( 'NONE', #23548, 1000.000000000000000 ) ;
#32389=PLANE ( 'NONE',  #67255 ) ;
#32399=VERTEX_POINT ( 'NONE', #3006 ) ;
#32420=DIRECTION ( 'NONE',  ( -0.000000000000000000, -0.000000000000000000, -1.000000000000000000 ) ) ;
#32421=CARTESIAN_POINT ( 'NONE',  ( 47.03029105687465261, 114.3563895605556269, -10.00000000000000000 ) ) ;
#32429=DIRECTION ( 'NONE',  ( 0.000000000000000000, 0.000000000000000000, -1.000000000000000000 ) ) ;
#32442=VECTOR ( 'NONE', #22312, 1000.000000000000114 ) ;
#32445=DIRECTION ( 'NONE',  ( 0.000000000000000000, 0.000000000000000000, 1.000000000000000000 ) ) ;
#32449=CARTESIAN_POINT ( 'NONE',  ( -4.824821883096095831, 80.30437515058552833, 13.53724619112298022 ) ) ;
#32451=DIRECTION ( 'NONE',  ( -0.000000000000000000, 0.000000000000000000, -1.000000000000000000 ) ) ;
#32453=PLANE ( 'NONE',  #32974 ) ;
#32461=ORIENTED_EDGE ( 'NONE', *, *, #19961, .T. ) ;
#32467=VERTEX_POINT ( 'NONE', #76848 ) ;
#32473=ORIENTED_EDGE ( 'NONE', *, *, #72364, .T. ) ;
#32474=ORIENTED_EDGE ( 'NONE', *, *, #13923, .T. ) ;
#32488=ADVANCED_FACE ( 'NONE', ( #7964 ), #7445, .F. ) ;
#32493=EDGE_CURVE ( 'NONE', #51511, #87203, #54522, .T. ) ;
#32507=DIRECTION ( 'NONE',  ( 0.4458072818673421978, 0.8951289669282590511, 0.000000000000000000 ) ) ;
#32508=EDGE_LOOP ( 'NONE', ( #13643, #24887, #30153, #74157 ) ) ;
#32511=CARTESIAN_POINT ( 'NONE',  ( 43.53831125515428369, 65.97156238185917232, -10.00000000000000000 ) ) ;
#32520=ORIENTED_EDGE ( 'NONE', *, *, #90858, .T. ) ;
#32526=AXIS2_PLACEMENT_3D ( 'NONE', #85916, #30656, #61539 ) ;
#32538=CARTESIAN_POINT ( 'NONE',  ( 43.63646518856938172, 66.22046553916848666, -10.00000000000000000 ) ) ;
#32545=CARTESIAN_POINT ( 'NONE',  ( -19.65312891409030271, 93.06504152958497400, -10.00000000000000888 ) ) ;
#32550=EDGE_CURVE ( 'NONE', #28252, #70323, #55526, .T. ) ;
#32558=DIRECTION ( 'NONE',  ( 0.000000000000000000, 0.000000000000000000, 1.000000000000000000 ) ) ;
#32568=DIRECTION ( 'NONE',  ( -0.5104483989331149996, -0.8599083858334093389, 0.000000000000000000 ) ) ;
#32575=CARTESIAN_POINT ( 'NONE',  ( -19.65312891409030271, 93.06504152958497400, -10.00000000000000888 ) ) ;
#32584=DIRECTION ( 'NONE',  ( -0.09248003802712849442, 0.9957145386939476595, 0.000000000000000000 ) ) ;
#32590=AXIS2_PLACEMENT_3D ( 'NONE', #15132, #83596, #60233 ) ;
#32592=VERTEX_POINT ( 'NONE', #41336 ) ;
#32593=EDGE_CURVE ( 'NONE', #53210, #80145, #95611, .T. ) ;
#32596=ORIENTED_EDGE ( 'NONE', *, *, #36819, .T. ) ;
#32599=EDGE_LOOP ( 'NONE', ( #79993, #37667, #2214, #61738 ) ) ;
#32609=ORIENTED_EDGE ( 'NONE', *, *, #54968, .F. ) ;
#32610=EDGE_CURVE ( 'NONE', #76706, #66378, #42336, .T. ) ;
#32611=DIRECTION ( 'NONE',  ( -0.09573633691163400961, -0.9954067278227238802, 0.000000000000000000 ) ) ;
#32616=VERTEX_POINT ( 'NONE', #58051 ) ;
#32621=LINE ( 'NONE', #16415, #69522 ) ;
#32623=LINE ( 'NONE', #70616, #57984 ) ;
#32630=ORIENTED_EDGE ( 'NONE', *, *, #99553, .T. ) ;
#32632=CARTESIAN_POINT ( 'NONE',  ( 48.83428215874786815, 87.09189275153327969, -10.00000000000000000 ) ) ;
#32634=FACE_OUTER_BOUND ( 'NONE', #55753, .T. ) ;
#32635=EDGE_CURVE ( 'NONE', #93745, #14058, #99921, .T. ) ;
#32642=EDGE_CURVE ( 'NONE', #6303, #50548, #89509, .T. ) ;
#32646=LINE ( 'NONE', #16442, #45452 ) ;
#32652=VERTEX_POINT ( 'NONE', #3381 ) ;
#32663=ORIENTED_EDGE ( 'NONE', *, *, #72268, .F. ) ;
#32667=CARTESIAN_POINT ( 'NONE',  ( 46.60452734134891273, 70.48356709729733893, 177.5919119679930134 ) ) ;
#32693=EDGE_LOOP ( 'NONE', ( #78081, #53798, #95063, #95949 ) ) ;
#32695=AXIS2_PLACEMENT_3D ( 'NONE', #12167, #73970, #80609 ) ;
#32717=CARTESIAN_POINT ( 'NONE',  ( 6.626006335531184455, 41.42259438955097295, 59.99999999999999289 ) ) ;
#32722=ORIENTED_EDGE ( 'NONE', *, *, #83749, .F. ) ;
#32757=EDGE_LOOP ( 'NONE', ( #98795, #69607 ) ) ;
#32765=VECTOR ( 'NONE', #46255, 1000.000000000000000 ) ;
#32774=CARTESIAN_POINT ( 'NONE',  ( 42.87860686303044844, 124.5258428655388911, -10.00000000000000000 ) ) ;
#32776=CARTESIAN_POINT ( 'NONE',  ( 25.88271472100439041, 39.90032630942972247, 10.00000000000000000 ) ) ;
#32795=CARTESIAN_POINT ( 'NONE',  ( 40.82928596147627331, 60.38352576601455723, 10.00000000000000000 ) ) ;
#32798=EDGE_CURVE ( 'NONE', #95045, #79982, #15167, .T. ) ;
#32807=DIRECTION ( 'NONE',  ( -0.000000000000000000, 0.000000000000000000, -1.000000000000000000 ) ) ;
#32808=CARTESIAN_POINT ( 'NONE',  ( -54.21831688459418785, 33.63902229265146104, 10.00000000000000000 ) ) ;
#32818=FACE_OUTER_BOUND ( 'NONE', #81582, .T. ) ;
#32823=VERTEX_POINT ( 'NONE', #2503 ) ;
#32826=VERTEX_POINT ( 'NONE', #39961 ) ;
#32830=DIRECTION ( 'NONE',  ( 0.000000000000000000, 0.000000000000000000, 1.000000000000000000 ) ) ;
#32831=ORIENTED_EDGE ( 'NONE', *, *, #30962, .T. ) ;
#32843=DIRECTION ( 'NONE',  ( -0.6911977992267216431, 0.7226656227773233798, 0.000000000000000000 ) ) ;
#32862=EDGE_CURVE ( 'NONE', #2950, #84918, #91925, .T. ) ;
#32863=ORIENTED_EDGE ( 'NONE', *, *, #34860, .F. ) ;
#32877=ORIENTED_EDGE ( 'NONE', *, *, #69523, .F. ) ;
#32899=VERTEX_POINT ( 'NONE', #10094 ) ;
#32906=CARTESIAN_POINT ( 'NONE',  ( -11.40312891409031693, 78.77562236714182120, 52.49999999999999289 ) ) ;
#32909=LINE ( 'NONE', #23808, #9715 ) ;
#32913=PLANE ( 'NONE',  #48501 ) ;
#32914=ORIENTED_EDGE ( 'NONE', *, *, #54833, .T. ) ;
#32919=LINE ( 'NONE', #63823, #88873 ) ;
#32922=CYLINDRICAL_SURFACE ( 'NONE', #45840, 11.89249999999999652 ) ;
#32928=CARTESIAN_POINT ( 'NONE',  ( 0.005075371086064872639, 27.18819441265828019, -10.00000000000000000 ) ) ;
#32934=CARTESIAN_POINT ( 'NONE',  ( -63.30067564770008914, 39.94154026010144065, 10.00000000000000000 ) ) ;
#32941=ORIENTED_EDGE ( 'NONE', *, *, #20929, .T. ) ;
#32942=LINE ( 'NONE', #8650, #7082 ) ;
#32943=CARTESIAN_POINT ( 'NONE',  ( 48.05801951159152452, 75.31115804243518141, -10.00000000000000000 ) ) ;
#32944=DIRECTION ( 'NONE',  ( -0.03277852384266333879, 0.9994626398093607866, 0.000000000000000000 ) ) ;
#32954=PLANE ( 'NONE',  #87807 ) ;
#32958=DIRECTION ( 'NONE',  ( 1.000000000000000000, 0.000000000000000000, 0.000000000000000000 ) ) ;
#32961=ORIENTED_EDGE ( 'NONE', *, *, #1513, .T. ) ;
#32974=AXIS2_PLACEMENT_3D ( 'NONE', #23837, #2062, #17241 ) ;
#32976=ORIENTED_EDGE ( 'NONE', *, *, #98535, .F. ) ;
#32977=DIRECTION ( 'NONE',  ( -0.4554470513245730823, -0.8902628732232696906, 0.000000000000000000 ) ) ;
#32982=EDGE_CURVE ( 'NONE', #52414, #28862, #27180, .T. ) ;
#32988=VERTEX_POINT ( 'NONE', #44459 ) ;
#32989=VECTOR ( 'NONE', #22867, 1000.000000000000000 ) ;
#33000=CIRCLE ( 'NONE', #29751, 70.00000000000001421 ) ;
#33018=FACE_OUTER_BOUND ( 'NONE', #13907, .T. ) ;
#33026=CARTESIAN_POINT ( 'NONE',  ( -17.81126293257621995, 23.08927765589694303, 177.5919119679930134 ) ) ;
#33034=CARTESIAN_POINT ( 'NONE',  ( -75.14068524134967220, 52.46521621197197760, -10.00000000000000000 ) ) ;
#33041=ORIENTED_EDGE ( 'NONE', *, *, #86968, .T. ) ;
#33051=EDGE_CURVE ( 'NONE', #91537, #11685, #1277, .T. ) ;
#33054=EDGE_CURVE ( 'NONE', #34850, #6051, #28161, .T. ) ;
#33058=CARTESIAN_POINT ( 'NONE',  ( 13.18854085237251184, 31.24736827225017066, 177.5919119679930134 ) ) ;
#33059=ORIENTED_EDGE ( 'NONE', *, *, #63291, .F. ) ;
#33060=VECTOR ( 'NONE', #26819, 1000.000000000000227 ) ;
#33071=CARTESIAN_POINT ( 'NONE',  ( -72.81784413424504976, 47.52919789448971244, 10.00000000000000000 ) ) ;
#33072=CIRCLE ( 'NONE', #31465, 0.1418229129684228651 ) ;
#33076=FACE_OUTER_BOUND ( 'NONE', #20448, .T. ) ;
#33084=VERTEX_POINT ( 'NONE', #36251 ) ;
#33088=CARTESIAN_POINT ( 'NONE',  ( -12.68721568607400485, 24.67147432707382748, -10.00000000000000000 ) ) ;
#33092=ORIENTED_EDGE ( 'NONE', *, *, #76401, .F. ) ;
#33098=ORIENTED_EDGE ( 'NONE', *, *, #73337, .T. ) ;
#33102=CARTESIAN_POINT ( 'NONE',  ( -66.21217304253431735, 40.79406095866392690, 10.00000000000000000 ) ) ;
#33103=VERTEX_POINT ( 'NONE', #4365 ) ;
#33106=FACE_OUTER_BOUND ( 'NONE', #14725, .T. ) ;
#33107=DIRECTION ( 'NONE',  ( 0.000000000000000000, 0.000000000000000000, 1.000000000000000000 ) ) ;
#33115=CARTESIAN_POINT ( 'NONE',  ( -17.81126293257622706, 23.08927765589692527, -10.00000000000000000 ) ) ;
#33118=CARTESIAN_POINT ( 'NONE',  ( 17.60357497223980516, 35.28838536716092023, 10.00000000000000000 ) ) ;
#33121=EDGE_CURVE ( 'NONE', #11929, #63370, #5368, .T. ) ;
#33123=CARTESIAN_POINT ( 'NONE',  ( -19.78867382312482803, 93.10677061150157385, 59.99999999999999289 ) ) ;
#33125=CARTESIAN_POINT ( 'NONE',  ( -61.60412911085353471, 37.02832515102500111, 10.00000000000000000 ) ) ;
#33131=ORIENTED_EDGE ( 'NONE', *, *, #27020, .F. ) ;
#33134=EDGE_CURVE ( 'NONE', #27844, #74106, #58551, .T. ) ;
#33135=DIRECTION ( 'NONE',  ( -0.8916269620120450545, 0.4527707594502665689, 0.000000000000000000 ) ) ;
#33136=ADVANCED_FACE ( 'NONE', ( #34270 ), #50459, .F. ) ;
#33137=AXIS2_PLACEMENT_3D ( 'NONE', #66521, #89863, #97448 ) ;
#33140=EDGE_LOOP ( 'NONE', ( #23224, #13788, #13221, #33906 ) ) ;
#33143=CARTESIAN_POINT ( 'NONE',  ( -15.09704997274537597, 40.23729735856676371, 59.99999999999999289 ) ) ;
#33147=AXIS2_PLACEMENT_3D ( 'NONE', #94291, #32944, #3570 ) ;
#33153=ORIENTED_EDGE ( 'NONE', *, *, #54078, .T. ) ;
#33160=DIRECTION ( 'NONE',  ( -0.000000000000000000, -0.000000000000000000, 1.000000000000000000 ) ) ;
#33166=ORIENTED_EDGE ( 'NONE', *, *, #41313, .T. ) ;
#33168=ADVANCED_FACE ( 'NONE', ( #89522 ), #35261, .F. ) ;
#33171=AXIS2_PLACEMENT_3D ( 'NONE', #24229, #84080, #46505 ) ;
#33178=EDGE_CURVE ( 'NONE', #63052, #28914, #98075, .T. ) ;
#33180=CARTESIAN_POINT ( 'NONE',  ( -48.47243291925848752, 30.64988553008148031, 10.00000000000000000 ) ) ;
#33204=CIRCLE ( 'NONE', #99535, 70.00000000000001421 ) ;
#33215=EDGE_CURVE ( 'NONE', #24657, #13582, #23529, .T. ) ;
#33218=ORIENTED_EDGE ( 'NONE', *, *, #54019, .T. ) ;
#33221=DIRECTION ( 'NONE',  ( 0.000000000000000000, 0.000000000000000000, 1.000000000000000000 ) ) ;
#33226=LINE ( 'NONE', #65127, #12505 ) ;
#33235=LINE ( 'NONE', #92581, #73897 ) ;
#33238=CARTESIAN_POINT ( 'NONE',  ( -25.62627769214124740, 24.57763045674671432, -10.00000000000000000 ) ) ;
#33243=ORIENTED_EDGE ( 'NONE', *, *, #57359, .T. ) ;
#33255=ADVANCED_FACE ( 'NONE', ( #71171 ), #54940, .F. ) ;
#33268=CARTESIAN_POINT ( 'NONE',  ( -59.87889494062799400, 37.30571521936384016, -10.00000000000000000 ) ) ;
#33280=DIRECTION ( 'NONE',  ( -0.000000000000000000, -0.000000000000000000, -1.000000000000000000 ) ) ;
#33287=CARTESIAN_POINT ( 'NONE',  ( 47.78135487164288264, 106.4364430393875267, -10.00000000000000000 ) ) ;
#33295=DIRECTION ( 'NONE',  ( -0.9682419296822714072, -0.2500151307524235422, 0.000000000000000000 ) ) ;
#33298=CARTESIAN_POINT ( 'NONE',  ( -19.65312891409030271, 93.06504152958497400, 10.00000000000000888 ) ) ;
#33310=LINE ( 'NONE', #95161, #10516 ) ;
#33311=VECTOR ( 'NONE', #3979, 1000.000000000000114 ) ;
#33320=DIRECTION ( 'NONE',  ( 0.000000000000000000, 0.000000000000000000, 1.000000000000000000 ) ) ;
#33322=ORIENTED_EDGE ( 'NONE', *, *, #30542, .T. ) ;
#33331=EDGE_LOOP ( 'NONE', ( #20526, #97120, #63604, #34699 ) ) ;
#33333=VERTEX_POINT ( 'NONE', #43227 ) ;
#33335=DIRECTION ( 'NONE',  ( -0.9997524133706772176, 0.02225111142182466945, 0.000000000000000000 ) ) ;
#33337=VERTEX_POINT ( 'NONE', #74169 ) ;
#33338=FACE_OUTER_BOUND ( 'NONE', #66485, .T. ) ;
#33340=LINE ( 'NONE', #15621, #78142 ) ;
#33342=CARTESIAN_POINT ( 'NONE',  ( 17.38248943320504836, 35.13769309531819829, -10.00000000000000000 ) ) ;
#33345=VECTOR ( 'NONE', #67034, 1000.000000000000114 ) ;
#33350=AXIS2_PLACEMENT_3D ( 'NONE', #32545, #93886, #71060 ) ;
#33351=VERTEX_POINT ( 'NONE', #58913 ) ;
#33356=CARTESIAN_POINT ( 'NONE',  ( -19.65312891409030271, 93.06504152958497400, 177.5919119679930134 ) ) ;
#33362=DIRECTION ( 'NONE',  ( 1.000000000000000000, 0.000000000000000000, 0.000000000000000000 ) ) ;
#33375=EDGE_CURVE ( 'NONE', #17718, #62885, #90394, .T. ) ;
#33379=EDGE_CURVE ( 'NONE', #33103, #14328, #62799, .T. ) ;
#33383=VERTEX_POINT ( 'NONE', #53807 ) ;
#33397=AXIS2_PLACEMENT_3D ( 'NONE', #28982, #36058, #67463 ) ;
#33399=CARTESIAN_POINT ( 'NONE',  ( -25.62627769214124740, 24.57763045674671432, 10.00000000000000000 ) ) ;
#33409=AXIS2_PLACEMENT_3D ( 'NONE', #12624, #5506, #68292 ) ;
#33410=VECTOR ( 'NONE', #68253, 1000.000000000000000 ) ;
#33425=ORIENTED_EDGE ( 'NONE', *, *, #86609, .T. ) ;
#33426=ADVANCED_FACE ( 'NONE', ( #70523 ), #1653, .F. ) ;
#33447=EDGE_CURVE ( 'NONE', #54743, #56966, #47711, .T. ) ;
#33449=CARTESIAN_POINT ( 'NONE',  ( -8.055044619196017663, 84.65328059711238495, 13.81882856671667525 ) ) ;
#33450=CARTESIAN_POINT ( 'NONE',  ( -8.406493707509316238, 25.24382671950691304, -10.00000000000000000 ) ) ;
#33452=ORIENTED_EDGE ( 'NONE', *, *, #64630, .T. ) ;
#33453=PLANE ( 'NONE',  #16774 ) ;
#33455=PLANE ( 'NONE',  #33147 ) ;
#33461=LINE ( 'NONE', #96292, #37071 ) ;
#33462=ORIENTED_EDGE ( 'NONE', *, *, #87671, .T. ) ;
#33474=ORIENTED_EDGE ( 'NONE', *, *, #31526, .F. ) ;
#33475=EDGE_LOOP ( 'NONE', ( #3755, #84725, #20898, #35867 ) ) ;
#33476=LINE ( 'NONE', #55247, #47112 ) ;
#33478=ORIENTED_EDGE ( 'NONE', *, *, #57691, .T. ) ;
#33480=DIRECTION ( 'NONE',  ( -0.000000000000000000, -0.000000000000000000, -1.000000000000000000 ) ) ;
#33490=VECTOR ( 'NONE', #7, 1000.000000000000000 ) ;
#33502=ORIENTED_EDGE ( 'NONE', *, *, #69842, .F. ) ;
#33506=DIRECTION ( 'NONE',  ( -0.8951289669282590511, 0.4458072818673421978, 0.000000000000000000 ) ) ;
#33508=CARTESIAN_POINT ( 'NONE',  ( -19.65312891409030271, 93.06504152958497400, 10.00000000000000888 ) ) ;
#33511=EDGE_CURVE ( 'NONE', #77610, #18050, #87312, .T. ) ;
#33517=CARTESIAN_POINT ( 'NONE',  ( 30.80155721116056711, 46.36891074996812279, -10.00000000000000000 ) ) ;
#33522=FACE_OUTER_BOUND ( 'NONE', #27508, .T. ) ;
#33523=DIRECTION ( 'NONE',  ( -1.000000000000000000, 0.000000000000000000, 0.000000000000000000 ) ) ;
#33535=LINE ( 'NONE', #34527, #74115 ) ;
#33537=VECTOR ( 'NONE', #46485, 1000.000000000000000 ) ;
#33548=CARTESIAN_POINT ( 'NONE',  ( 48.77433535142598231, 99.76555324011610537, -10.00000000000000000 ) ) ;
#33549=VECTOR ( 'NONE', #2380, 1000.000000000000000 ) ;
#33553=DIRECTION ( 'NONE',  ( -0.6835488936653838499, -0.7299047266382303611, 0.000000000000000000 ) ) ;
#33570=EDGE_CURVE ( 'NONE', #97892, #38977, #92861, .T. ) ;
#33578=DIRECTION ( 'NONE',  ( 0.000000000000000000, 0.000000000000000000, 1.000000000000000000 ) ) ;
#33579=EDGE_CURVE ( 'NONE', #2846, #68611, #35335, .T. ) ;
#33580=DIRECTION ( 'NONE',  ( -0.9292718480896766664, -0.3693965786901617920, 0.000000000000000000 ) ) ;
#33582=DIRECTION ( 'NONE',  ( -0.9514785060800255989, 0.3077152132536228324, 0.000000000000000000 ) ) ;
#33585=PLANE ( 'NONE',  #43862 ) ;
#33594=VERTEX_POINT ( 'NONE', #32016 ) ;
#33604=ORIENTED_EDGE ( 'NONE', *, *, #11780, .T. ) ;
#33608=EDGE_LOOP ( 'NONE', ( #89467, #93813, #80670, #42183 ) ) ;
#33616=VECTOR ( 'NONE', #91285, 1000.000000000000114 ) ;
#33618=ORIENTED_EDGE ( 'NONE', *, *, #99360, .T. ) ;
#33619=EDGE_CURVE ( 'NONE', #28770, #4321, #54305, .T. ) ;
#33622=ORIENTED_EDGE ( 'NONE', *, *, #26204, .F. ) ;
#33628=AXIS2_PLACEMENT_3D ( 'NONE', #84287, #15315, #77133 ) ;
#33636=EDGE_CURVE ( 'NONE', #71153, #4561, #70018, .T. ) ;
#33649=EDGE_CURVE ( 'NONE', #96111, #55260, #64409, .T. ) ;
#33658=CARTESIAN_POINT ( 'NONE',  ( -37.20311282697427657, 64.84237164687553445, -10.00000000000000000 ) ) ;
#33660=LINE ( 'NONE', #10358, #92070 ) ;
#33667=DIRECTION ( 'NONE',  ( 0.000000000000000000, 0.000000000000000000, 1.000000000000000000 ) ) ;
#33680=ORIENTED_EDGE ( 'NONE', *, *, #30542, .F. ) ;
#33685=AXIS2_PLACEMENT_3D ( 'NONE', #10324, #48317, #10821 ) ;
#33704=LINE ( 'NONE', #64597, #88161 ) ;
#33706=LINE ( 'NONE', #81333, #45177 ) ;
#33712=CARTESIAN_POINT ( 'NONE',  ( -19.65312891409030271, 93.06504152958497400, -10.00000000000000888 ) ) ;
#33713=DIRECTION ( 'NONE',  ( 0.000000000000000000, 0.000000000000000000, 1.000000000000000000 ) ) ;
#33716=ORIENTED_EDGE ( 'NONE', *, *, #9515, .F. ) ;
#33721=ADVANCED_FACE ( 'NONE', ( #40615 ), #71549, .F. ) ;
#33722=EDGE_CURVE ( 'NONE', #85517, #41680, #72560, .T. ) ;
#33728=ORIENTED_EDGE ( 'NONE', *, *, #2526, .T. ) ;
#33731=DIRECTION ( 'NONE',  ( -0.8660254037844379305, -0.5000000000000011102, -0.000000000000000000 ) ) ;
#33732=VERTEX_POINT ( 'NONE', #12748 ) ;
#33736=VERTEX_POINT ( 'NONE', #64938 ) ;
#33742=DIRECTION ( 'NONE',  ( 0.7694697644498921241, -0.6386832404231594928, 0.000000000000000000 ) ) ;
#33746=ORIENTED_EDGE ( 'NONE', *, *, #7196, .T. ) ;
#33747=EDGE_CURVE ( 'NONE', #45184, #74753, #10740, .T. ) ;
#33755=ORIENTED_EDGE ( 'NONE', *, *, #51100, .F. ) ;
#33756=EDGE_CURVE ( 'NONE', #566, #95472, #95394, .T. ) ;
#33763=CARTESIAN_POINT ( 'NONE',  ( 42.33744422746375591, 122.7866300363639169, -10.00000000000000000 ) ) ;
#33764=ADVANCED_FACE ( 'NONE', ( #74551 ), #42606, .T. ) ;
#33765=VECTOR ( 'NONE', #17129, 1000.000000000000227 ) ;
#33767=EDGE_CURVE ( 'NONE', #60917, #46791, #33535, .T. ) ;
#33771=CIRCLE ( 'NONE', #46673, 70.00000000000001421 ) ;
#33773=CIRCLE ( 'NONE', #54768, 0.1418229129680828593 ) ;
#33776=ORIENTED_EDGE ( 'NONE', *, *, #41947, .T. ) ;
#33781=CARTESIAN_POINT ( 'NONE',  ( -24.40473831032599961, 23.22649767201583515, 10.00000000000000000 ) ) ;
#33784=DIRECTION ( 'NONE',  ( 0.000000000000000000, 0.000000000000000000, 1.000000000000000000 ) ) ;
#33788=VECTOR ( 'NONE', #95561, 1000.000000000000000 ) ;
#33794=CARTESIAN_POINT ( 'NONE',  ( 47.39496755818312579, 108.2889530649357681, 10.00000000000000000 ) ) ;
#33798=CARTESIAN_POINT ( 'NONE',  ( -50.41871976035449165, 31.58591985673633928, -10.00000000000000000 ) ) ;
#33800=AXIS2_PLACEMENT_3D ( 'NONE', #48639, #79573, #95284 ) ;
#33812=DIRECTION ( 'NONE',  ( -0.000000000000000000, -0.000000000000000000, -1.000000000000000000 ) ) ;
#33829=EDGE_CURVE ( 'NONE', #1860, #26784, #49868, .T. ) ;
#33833=CARTESIAN_POINT ( 'NONE',  ( 37.34220537994157496, 54.61056725541210710, -10.00000000000000000 ) ) ;
#33838=DIRECTION ( 'NONE',  ( -0.000000000000000000, -0.000000000000000000, -1.000000000000000000 ) ) ;
#33843=VECTOR ( 'NONE', #57429, 1000.000000000000114 ) ;
#33850=CARTESIAN_POINT ( 'NONE',  ( 48.58805178314242568, 84.67719436603331928, -10.00000000000000000 ) ) ;
#33863=CARTESIAN_POINT ( 'NONE',  ( 48.21858077004885246, 104.0489273421469818, 10.00000000000000000 ) ) ;
#33866=ORIENTED_EDGE ( 'NONE', *, *, #89149, .F. ) ;
#33867=CARTESIAN_POINT ( 'NONE',  ( -54.45295541630240166, 33.76759809053437067, -10.00000000000000000 ) ) ;
#33870=AXIS2_PLACEMENT_3D ( 'NONE', #95553, #95034, #79833 ) ;
#33878=LINE ( 'NONE', #11073, #62185 ) ;
#33884=LINE ( 'NONE', #92102, #47977 ) ;
#33891=ORIENTED_EDGE ( 'NONE', *, *, #67961, .T. ) ;
#33896=ORIENTED_EDGE ( 'NONE', *, *, #93357, .F. ) ;
#33899=CARTESIAN_POINT ( 'NONE',  ( -59.65739779450132829, 37.15562860896454112, -10.00000000000000000 ) ) ;
#33900=DIRECTION ( 'NONE',  ( -1.000000000000000000, 0.000000000000000000, 0.000000000000000000 ) ) ;
#33906=ORIENTED_EDGE ( 'NONE', *, *, #68021, .F. ) ;
#33909=LINE ( 'NONE', #47208, #1064 ) ;
#33917=CARTESIAN_POINT ( 'NONE',  ( -34.16292631813981728, 25.86630820016799248, 10.00000000000000000 ) ) ;
#33918=CARTESIAN_POINT ( 'NONE',  ( 48.21858077004885246, 104.0489273421469818, -10.00000000000000000 ) ) ;
#33930=ADVANCED_FACE ( 'NONE', ( #64008 ), #17407, .F. ) ;
#33947=DIRECTION ( 'NONE',  ( 0.3956464567955564338, -0.9184028970038813355, 0.000000000000000000 ) ) ;
#33960=EDGE_CURVE ( 'NONE', #41197, #39035, #19171, .T. ) ;
#33969=ORIENTED_EDGE ( 'NONE', *, *, #53279, .T. ) ;
#33986=DIRECTION ( 'NONE',  ( -0.8916269620120498285, 0.4527707594502571875, 0.000000000000000000 ) ) ;
#33991=DIRECTION ( 'NONE',  ( -0.6911977992267138715, 0.7226656227773308183, 0.000000000000000000 ) ) ;
#33992=EDGE_LOOP ( 'NONE', ( #90228, #68969, #69146, #46149 ) ) ;
#33993=VECTOR ( 'NONE', #33553, 1000.000000000000000 ) ;
#33994=ORIENTED_EDGE ( 'NONE', *, *, #95050, .F. ) ;
#34007=ORIENTED_EDGE ( 'NONE', *, *, #38335, .T. ) ;
#34019=CARTESIAN_POINT ( 'NONE',  ( 43.35468487962021555, 120.5828561944265687, 10.00000000000000000 ) ) ;
#34033=VERTEX_POINT ( 'NONE', #98912 ) ;
#34035=CARTESIAN_POINT ( 'NONE',  ( -35.25453232515824453, 42.38837410636706693, 59.99999999999999289 ) ) ;
#34057=VECTOR ( 'NONE', #49353, 999.9999999999998863 ) ;
#34070=CARTESIAN_POINT ( 'NONE',  ( 47.92671612011951510, 80.40884667711614497, -10.00000000000000000 ) ) ;
#34078=DIRECTION ( 'NONE',  ( 1.000000000000000000, 0.000000000000000000, 0.000000000000000000 ) ) ;
#34087=ADVANCED_FACE ( 'NONE', ( #60369 ), #84727, .F. ) ;
#34107=ORIENTED_EDGE ( 'NONE', *, *, #29040, .T. ) ;
#34114=ORIENTED_EDGE ( 'NONE', *, *, #66263, .T. ) ;
#34118=ORIENTED_EDGE ( 'NONE', *, *, #36828, .F. ) ;
#34121=FACE_OUTER_BOUND ( 'NONE', #31725, .T. ) ;
#34137=DIRECTION ( 'NONE',  ( -0.6855440362341480576, 0.7280311630581436377, 0.000000000000000000 ) ) ;
#34139=EDGE_CURVE ( 'NONE', #31364, #15864, #8689, .T. ) ;
#34141=CARTESIAN_POINT ( 'NONE',  ( -8.669243101527598583, 25.19333184544593252, -10.00000000000000000 ) ) ;
#34143=EDGE_LOOP ( 'NONE', ( #98910, #30220 ) ) ;
#34151=ORIENTED_EDGE ( 'NONE', *, *, #6573, .F. ) ;
#34154=CARTESIAN_POINT ( 'NONE',  ( -19.67426652243475615, 92.92480266137719980, 59.99999999999999289 ) ) ;
#34155=EDGE_CURVE ( 'NONE', #59347, #30332, #92819, .T. ) ;
#34159=DIRECTION ( 'NONE',  ( -1.000000000000000000, 0.000000000000000000, 0.000000000000000000 ) ) ;
#34176=CARTESIAN_POINT ( 'NONE',  ( -42.23460334637722013, 26.80738527414552053, 177.5919119679930134 ) ) ;
#34182=EDGE_CURVE ( 'NONE', #57311, #57629, #28823, .T. ) ;
#34183=DIRECTION ( 'NONE',  ( -0.000000000000000000, -0.000000000000000000, 1.000000000000000000 ) ) ;
#34188=VECTOR ( 'NONE', #9175, 999.9999999999998863 ) ;
#34190=CARTESIAN_POINT ( 'NONE',  ( 38.21438390411638153, 96.04939573986766277, 59.99999999999999289 ) ) ;
#34198=CARTESIAN_POINT ( 'NONE',  ( 25.95381284194209215, 117.4816347750370369, 59.99999999999999289 ) ) ;
#34204=CARTESIAN_POINT ( 'NONE',  ( -75.14068524134968641, 52.46521621197197760, -10.00000000000000000 ) ) ;
#34212=CARTESIAN_POINT ( 'NONE',  ( 21.15788363470973366, 37.74176219324819215, -10.00000000000000000 ) ) ;
#34218=ORIENTED_EDGE ( 'NONE', *, *, #77158, .F. ) ;
#34233=ORIENTED_EDGE ( 'NONE', *, *, #56574, .T. ) ;
#34235=ORIENTED_EDGE ( 'NONE', *, *, #26893, .F. ) ;
#34236=DIRECTION ( 'NONE',  ( 0.000000000000000000, 0.000000000000000000, 1.000000000000000000 ) ) ;
#34237=DIRECTION ( 'NONE',  ( -1.000000000000000000, 9.785293164094327883E-14, 0.000000000000000000 ) ) ;
#34258=CARTESIAN_POINT ( 'NONE',  ( 21.61448739737248559, 51.35407934543722774, 59.99999999999999289 ) ) ;
#34261=DIRECTION ( 'NONE',  ( -0.000000000000000000, -0.000000000000000000, -1.000000000000000000 ) ) ;
#34270=FACE_OUTER_BOUND ( 'NONE', #27571, .T. ) ;
#34273=DIRECTION ( 'NONE',  ( -0.9182972510888841589, 0.3958915996110536906, 0.000000000000000000 ) ) ;
#34280=LINE ( 'NONE', #11992, #62943 ) ;
#34281=EDGE_CURVE ( 'NONE', #47682, #10473, #27880, .T. ) ;
#34284=DIRECTION ( 'NONE',  ( -1.000000000000000000, 0.000000000000000000, 0.000000000000000000 ) ) ;
#34289=DIRECTION ( 'NONE',  ( -0.04218457335174585071, -0.9991098346884246251, 0.000000000000000000 ) ) ;
#34291=LINE ( 'NONE', #65188, #96634 ) ;
#34295=PLANE ( 'NONE',  #75926 ) ;
#34297=EDGE_CURVE ( 'NONE', #33351, #49306, #79044, .T. ) ;
#34298=DIRECTION ( 'NONE',  ( 1.000000000000000000, 0.000000000000000000, 0.000000000000000000 ) ) ;
#34302=EDGE_CURVE ( 'NONE', #20754, #74292, #43575, .T. ) ;
#34307=EDGE_CURVE ( 'NONE', #1103, #4020, #82248, .T. ) ;
#34309=CARTESIAN_POINT ( 'NONE',  ( -68.29659580619643577, 42.72804590294295224, -10.00000000000000000 ) ) ;
#34323=VERTEX_POINT ( 'NONE', #36469 ) ;
#34338=CARTESIAN_POINT ( 'NONE',  ( -19.65312891409030271, 93.06504152958497400, 177.5919119679930134 ) ) ;
#34356=DIRECTION ( 'NONE',  ( -0.000000000000000000, -0.000000000000000000, -1.000000000000000000 ) ) ;
#34364=ORIENTED_EDGE ( 'NONE', *, *, #39691, .T. ) ;
#34369=VERTEX_POINT ( 'NONE', #20799 ) ;
#34374=CARTESIAN_POINT ( 'NONE',  ( 42.33744422746375591, 122.7866300363639169, 10.00000000000000000 ) ) ;
#34377=ORIENTED_EDGE ( 'NONE', *, *, #46009, .F. ) ;
#34378=VERTEX_POINT ( 'NONE', #19803 ) ;
#34379=CARTESIAN_POINT ( 'NONE',  ( 24.69086998626516305, 38.90223361192549589, 10.00000000000000000 ) ) ;
#34380=ORIENTED_EDGE ( 'NONE', *, *, #94976, .F. ) ;
#34382=AXIS2_PLACEMENT_3D ( 'NONE', #12735, #87792, #65413 ) ;
#34388=DIRECTION ( 'NONE',  ( -0.1032265479692960342, 0.9946578707245736783, 0.000000000000000000 ) ) ;
#34389=FACE_OUTER_BOUND ( 'NONE', #73134, .T. ) ;
#34398=EDGE_CURVE ( 'NONE', #90851, #45207, #13685, .T. ) ;
#34399=CARTESIAN_POINT ( 'NONE',  ( 40.70814378237798081, 60.14496435084704018, -10.00000000000000000 ) ) ;
#34412=CARTESIAN_POINT ( 'NONE',  ( 27.76992210170819675, 43.29297894285233639, -10.00000000000000000 ) ) ;
#34414=PLANE ( 'NONE',  #25462 ) ;
#34415=CYLINDRICAL_SURFACE ( 'NONE', #22634, 70.00000000000002842 ) ;
#34436=VECTOR ( 'NONE', #91425, 1000.000000000000000 ) ;
#34440=PLANE ( 'NONE',  #96025 ) ;
#34443=VERTEX_POINT ( 'NONE', #17671 ) ;
#34444=CARTESIAN_POINT ( 'NONE',  ( 30.62489312496363425, 46.16797101519271962, 10.00000000000000000 ) ) ;
#34447=ORIENTED_EDGE ( 'NONE', *, *, #45572, .T. ) ;
#34448=CIRCLE ( 'NONE', #40936, 70.00000000000001421 ) ;
#34467=ORIENTED_EDGE ( 'NONE', *, *, #77413, .F. ) ;
#34470=EDGE_LOOP ( 'NONE', ( #79875, #88633 ) ) ;
#34472=LINE ( 'NONE', #27869, #82030 ) ;
#34478=DIRECTION ( 'NONE',  ( 0.000000000000000000, 0.000000000000000000, 1.000000000000000000 ) ) ;
#34479=ORIENTED_EDGE ( 'NONE', *, *, #34139, .T. ) ;
#34481=EDGE_LOOP ( 'NONE', ( #34364, #32083, #27297, #96451 ) ) ;
#34490=VERTEX_POINT ( 'NONE', #88129 ) ;
#34499=EDGE_CURVE ( 'NONE', #69721, #52564, #63764, .T. ) ;
#34500=DIRECTION ( 'NONE',  ( 1.000000000000000000, 0.000000000000000000, 0.000000000000000000 ) ) ;
#34503=DIRECTION ( 'NONE',  ( -0.000000000000000000, 0.000000000000000000, 1.000000000000000000 ) ) ;
#34505=ORIENTED_EDGE ( 'NONE', *, *, #25170, .F. ) ;
#34510=PLANE ( 'NONE',  #30298 ) ;
#34515=ADVANCED_FACE ( 'NONE', ( #18170 ), #18675, .F. ) ;
#34517=CARTESIAN_POINT ( 'NONE',  ( 49.17298586869600285, 105.8308522718264584, 177.5919119679930134 ) ) ;
#34520=ADVANCED_FACE ( 'NONE', ( #49072 ), #56141, .F. ) ;
#34521=DIRECTION ( 'NONE',  ( 0.1548189829846108034, -0.9879428538673736826, 0.000000000000000000 ) ) ;
#34522=CARTESIAN_POINT ( 'NONE',  ( 42.65610334793077385, 64.00004027534475881, -10.00000000000000000 ) ) ;
#34525=AXIS2_PLACEMENT_3D ( 'NONE', #15888, #30605, #47779 ) ;
#34527=CARTESIAN_POINT ( 'NONE',  ( 13.75631770279070842, 31.55236904046465440, 177.5919119679930134 ) ) ;
#34531=PLANE ( 'NONE',  #93619 ) ;
#34570=EDGE_CURVE ( 'NONE', #81007, #72976, #85569, .T. ) ;
#34576=ORIENTED_EDGE ( 'NONE', *, *, #10692, .T. ) ;
#34579=EDGE_LOOP ( 'NONE', ( #26031, #6327, #78343, #70844 ) ) ;
#34588=VECTOR ( 'NONE', #4268, 1000.000000000000227 ) ;
#34590=ORIENTED_EDGE ( 'NONE', *, *, #36828, .T. ) ;
#34593=EDGE_LOOP ( 'NONE', ( #83458, #96676, #24165, #72659 ) ) ;
#34598=ORIENTED_EDGE ( 'NONE', *, *, #80546, .F. ) ;
#34605=DIRECTION ( 'NONE',  ( 0.000000000000000000, 0.000000000000000000, 1.000000000000000000 ) ) ;
#34608=EDGE_LOOP ( 'NONE', ( #48573, #45785, #20387, #62580 ) ) ;
#34615=CARTESIAN_POINT ( 'NONE',  ( -44.67997007436067491, 47.78987728549608960, 59.99999999999999289 ) ) ;
#34632=EDGE_CURVE ( 'NONE', #98268, #91064, #69310, .T. ) ;
#34634=ORIENTED_EDGE ( 'NONE', *, *, #97626, .F. ) ;
#34635=DIRECTION ( 'NONE',  ( -0.9413434404457865501, 0.3374500364938337049, 0.000000000000000000 ) ) ;
#34636=DIRECTION ( 'NONE',  ( -0.9263643838751194348, -0.3766285016932073293, 0.000000000000000000 ) ) ;
#34637=EDGE_CURVE ( 'NONE', #17528, #9585, #4456, .T. ) ;
#34639=EDGE_CURVE ( 'NONE', #20627, #7148, #50545, .T. ) ;
#34644=CARTESIAN_POINT ( 'NONE',  ( 17.60357497223980516, 35.28838536716092023, -10.00000000000000000 ) ) ;
#34647=DIRECTION ( 'NONE',  ( 0.7490285521785712275, -0.6625377181876315191, 0.000000000000000000 ) ) ;
#34656=CARTESIAN_POINT ( 'NONE',  ( 22.66956910419568061, 38.88013629349136835, -10.00000000000000000 ) ) ;
#34660=VERTEX_POINT ( 'NONE', #50062 ) ;
#34669=LINE ( 'NONE', #33180, #10136 ) ;
#34673=VERTEX_POINT ( 'NONE', #27270 ) ;
#34676=CARTESIAN_POINT ( 'NONE',  ( -40.42249077443059235, 27.53003111760058630, -10.00000000000000000 ) ) ;
#34680=CARTESIAN_POINT ( 'NONE',  ( 48.98007068238331385, 88.97864505566217019, -10.00000000000000000 ) ) ;
#34684=ORIENTED_EDGE ( 'NONE', *, *, #95076, .T. ) ;
#34697=DIRECTION ( 'NONE',  ( -0.8660254037844378194, -0.5000000000000013323, 0.000000000000000000 ) ) ;
#34699=ORIENTED_EDGE ( 'NONE', *, *, #98556, .F. ) ;
#34702=DIRECTION ( 'NONE',  ( -1.000000000000000000, 0.000000000000000000, 0.000000000000000000 ) ) ;
#34707=DIRECTION ( 'NONE',  ( -0.9999986627203611977, 0.001635407438350361181, 0.000000000000000000 ) ) ;
#34723=DIRECTION ( 'NONE',  ( -0.7492053821869066876, -0.6623377501714446947, 0.000000000000000000 ) ) ;
#34724=AXIS2_PLACEMENT_3D ( 'NONE', #87905, #58892, #42704 ) ;
#34728=ORIENTED_EDGE ( 'NONE', *, *, #1377, .T. ) ;
#34754=DIRECTION ( 'NONE',  ( -1.000000000000000000, 0.000000000000000000, 0.000000000000000000 ) ) ;
#34762=AXIS2_PLACEMENT_3D ( 'NONE', #26504, #43163, #11323 ) ;
#34771=DIRECTION ( 'NONE',  ( -0.7253665389804496710, -0.6883628288392130701, 0.000000000000000000 ) ) ;
#34775=FACE_OUTER_BOUND ( 'NONE', #7466, .T. ) ;
#34781=CARTESIAN_POINT ( 'NONE',  ( -4.170157060006060235, 26.08383846222962887, -10.00000000000000000 ) ) ;
#34790=VECTOR ( 'NONE', #82477, 1000.000000000000000 ) ;
#34808=LINE ( 'NONE', #50511, #32309 ) ;
#34819=ORIENTED_EDGE ( 'NONE', *, *, #30860, .F. ) ;
#34820=CARTESIAN_POINT ( 'NONE',  ( -19.51954277429316065, 93.11267011235696600, 59.99999999999999289 ) ) ;
#34821=ORIENTED_EDGE ( 'NONE', *, *, #76722, .F. ) ;
#34824=PLANE ( 'NONE',  #86638 ) ;
#34840=LINE ( 'NONE', #88619, #27042 ) ;
#34850=VERTEX_POINT ( 'NONE', #74272 ) ;
#34851=EDGE_CURVE ( 'NONE', #46284, #3544, #97565, .T. ) ;
#34856=DIRECTION ( 'NONE',  ( 0.1162373735601320568, 0.9932214622066130039, 0.000000000000000000 ) ) ;
#34860=EDGE_CURVE ( 'NONE', #15908, #67111, #65635, .T. ) ;
#34863=VERTEX_POINT ( 'NONE', #81879 ) ;
#34864=EDGE_CURVE ( 'NONE', #89739, #84849, #42817, .T. ) ;
#34865=CIRCLE ( 'NONE', #91526, 70.00000000000001421 ) ;
#34868=DIRECTION ( 'NONE',  ( 0.6116140086401538056, -0.7911563084720502070, 0.000000000000000000 ) ) ;
#34873=DIRECTION ( 'NONE',  ( -0.9514785060800255989, 0.3077152132536228879, 0.000000000000000000 ) ) ;
#34874=ORIENTED_EDGE ( 'NONE', *, *, #42302, .F. ) ;
#34880=FACE_OUTER_BOUND ( 'NONE', #72702, .T. ) ;
#34882=CARTESIAN_POINT ( 'NONE',  ( -19.65312891409030271, 93.06504152958497400, -10.00000000000000888 ) ) ;
#34884=PLANE ( 'NONE',  #85126 ) ;
#34892=CIRCLE ( 'NONE', #60762, 70.00000000000001421 ) ;
#34897=LINE ( 'NONE', #81068, #7232 ) ;
#34899=CIRCLE ( 'NONE', #99576, 0.1418229129680897982 ) ;
#34916=VECTOR ( 'NONE', #13840, 1000.000000000000000 ) ;
#34921=ADVANCED_FACE ( 'NONE', ( #1228 ), #93965, .T. ) ;
#34922=PLANE ( 'NONE',  #82317 ) ;
#34923=AXIS2_PLACEMENT_3D ( 'NONE', #38892, #24695, #39872 ) ;
#34926=DIRECTION ( 'NONE',  ( -0.9762143704923794685, 0.2168075248790211351, 0.000000000000000000 ) ) ;
#34927=ORIENTED_EDGE ( 'NONE', *, *, #29524, .F. ) ;
#34929=ORIENTED_EDGE ( 'NONE', *, *, #73759, .F. ) ;
#34930=CARTESIAN_POINT ( 'NONE',  ( -13.14524566621093626, 85.30073937114704563, 14.89871103469313951 ) ) ;
#34932=EDGE_CURVE ( 'NONE', #39677, #65525, #86382, .T. ) ;
#34934=VERTEX_POINT ( 'NONE', #9326 ) ;
#34936=CARTESIAN_POINT ( 'NONE',  ( -10.54235908185773418, 24.92402704602492847, 10.00000000000000000 ) ) ;
#34944=DIRECTION ( 'NONE',  ( 0.000000000000000000, 0.000000000000000000, 1.000000000000000000 ) ) ;
#34945=DIRECTION ( 'NONE',  ( -0.000000000000000000, -0.000000000000000000, 1.000000000000000000 ) ) ;
#34946=EDGE_CURVE ( 'NONE', #7407, #34378, #48328, .T. ) ;
#34947=ORIENTED_EDGE ( 'NONE', *, *, #75650, .T. ) ;
#34949=DIRECTION ( 'NONE',  ( 0.000000000000000000, 0.000000000000000000, 1.000000000000000000 ) ) ;
#34953=ORIENTED_EDGE ( 'NONE', *, *, #48500, .T. ) ;
#34962=CARTESIAN_POINT ( 'NONE',  ( 32.06973406193871057, 92.10133962881208447, 59.99999999999999289 ) ) ;
#34967=VERTEX_POINT ( 'NONE', #65028 ) ;
#34970=ORIENTED_EDGE ( 'NONE', *, *, #82290, .T. ) ;
#34973=CARTESIAN_POINT ( 'NONE',  ( -19.65312891409030271, 93.06504152958497400, -10.00000000000000888 ) ) ;
#34978=CIRCLE ( 'NONE', #77058, 70.00000000000001421 ) ;
#34983=CARTESIAN_POINT ( 'NONE',  ( -32.57204513736933649, 62.44441720109064420, -10.00000000000000000 ) ) ;
#34986=CARTESIAN_POINT ( 'NONE',  ( -19.74036418170400609, 92.95322137609242930, 59.99999999999999289 ) ) ;
#34999=CIRCLE ( 'NONE', #98159, 70.00000000000001421 ) ;
#35001=DIRECTION ( 'NONE',  ( 0.8902628732232650277, -0.4554470513245822971, 0.000000000000000000 ) ) ;
#35002=LINE ( 'NONE', #64419, #42460 ) ;
#35005=CARTESIAN_POINT ( 'NONE',  ( -26.59607535340071394, 23.41021043553328695, 177.5919119679930134 ) ) ;
#35006=DIRECTION ( 'NONE',  ( -0.000000000000000000, -0.000000000000000000, -1.000000000000000000 ) ) ;
#35009=DIRECTION ( 'NONE',  ( 0.000000000000000000, -0.000000000000000000, -1.000000000000000000 ) ) ;
#35026=ORIENTED_EDGE ( 'NONE', *, *, #57373, .T. ) ;
#35027=ADVANCED_FACE ( 'NONE', ( #35110 ), #96466, .T. ) ;
#35046=VECTOR ( 'NONE', #29465, 1000.000000000000114 ) ;
#35055=EDGE_CURVE ( 'NONE', #5025, #98414, #82269, .T. ) ;
#35065=VECTOR ( 'NONE', #7737, 1000.000000000000000 ) ;
#35070=CARTESIAN_POINT ( 'NONE',  ( -19.65312891409030271, 93.06504152958497400, -10.00000000000000888 ) ) ;
#35071=EDGE_CURVE ( 'NONE', #30332, #16059, #43703, .T. ) ;
#35075=VECTOR ( 'NONE', #42304, 1000.000000000000227 ) ;
#35079=ORIENTED_EDGE ( 'NONE', *, *, #46640, .T. ) ;
#35091=CARTESIAN_POINT ( 'NONE',  ( 27.53018959221258655, 41.35687530090521591, 10.00000000000000000 ) ) ;
#35092=ORIENTED_EDGE ( 'NONE', *, *, #91935, .T. ) ;
#35096=ORIENTED_EDGE ( 'NONE', *, *, #96548, .F. ) ;
#35098=ORIENTED_EDGE ( 'NONE', *, *, #81431, .T. ) ;
#35104=CARTESIAN_POINT ( 'NONE',  ( 48.21858077004886667, 104.0489273421469818, -10.00000000000000000 ) ) ;
#35110=FACE_OUTER_BOUND ( 'NONE', #8683, .T. ) ;
#35112=ORIENTED_EDGE ( 'NONE', *, *, #46783, .F. ) ;
#35120=ORIENTED_EDGE ( 'NONE', *, *, #46920, .F. ) ;
#35123=ADVANCED_FACE ( 'NONE', ( #62380 ), #23891, .F. ) ;
#35125=CARTESIAN_POINT ( 'NONE',  ( 46.30674614090290220, 112.4688969640381231, -10.00000000000000000 ) ) ;
#35128=VERTEX_POINT ( 'NONE', #93337 ) ;
#35131=DIRECTION ( 'NONE',  ( 1.000000000000000000, 0.000000000000000000, 0.000000000000000000 ) ) ;
#35142=ORIENTED_EDGE ( 'NONE', *, *, #17605, .T. ) ;
#35143=VECTOR ( 'NONE', #16195, 1000.000000000000000 ) ;
#35145=EDGE_LOOP ( 'NONE', ( #30371, #55936, #23034, #46145 ) ) ;
#35146=CARTESIAN_POINT ( 'NONE',  ( -46.35039662390602899, 28.35603213498495023, 177.5919119679930134 ) ) ;
#35148=CARTESIAN_POINT ( 'NONE',  ( -35.27139336136212933, 24.82964151130202879, -10.00000000000000000 ) ) ;
#35152=FACE_OUTER_BOUND ( 'NONE', #22101, .T. ) ;
#35158=EDGE_CURVE ( 'NONE', #8078, #97948, #8208, .T. ) ;
#35164=LINE ( 'NONE', #74694, #82397 ) ;
#35170=ORIENTED_EDGE ( 'NONE', *, *, #55441, .F. ) ;
#35173=FACE_OUTER_BOUND ( 'NONE', #68124, .T. ) ;
#35178=DIRECTION ( 'NONE',  ( -0.6681572590663601430, 0.7440200784635646603, 0.000000000000000000 ) ) ;
#35185=AXIS2_PLACEMENT_3D ( 'NONE', #53322, #91366, #84769 ) ;
#35201=ORIENTED_EDGE ( 'NONE', *, *, #41154, .F. ) ;
#35203=EDGE_CURVE ( 'NONE', #22789, #95233, #97324, .T. ) ;
#35206=EDGE_LOOP ( 'NONE', ( #16827, #63009, #90470, #35933 ) ) ;
#35216=ORIENTED_EDGE ( 'NONE', *, *, #92683, .T. ) ;
#35219=VECTOR ( 'NONE', #28375, 1000.000000000000000 ) ;
#35227=ORIENTED_EDGE ( 'NONE', *, *, #91067, .F. ) ;
#35230=EDGE_LOOP ( 'NONE', ( #73782, #50165, #30706, #96332 ) ) ;
#35232=AXIS2_PLACEMENT_3D ( 'NONE', #5897, #28701, #29695 ) ;
#35235=FACE_OUTER_BOUND ( 'NONE', #30868, .T. ) ;
#35236=DIRECTION ( 'NONE',  ( 0.000000000000000000, -0.000000000000000000, -1.000000000000000000 ) ) ;
#35242=ORIENTED_EDGE ( 'NONE', *, *, #62968, .T. ) ;
#35248=FACE_OUTER_BOUND ( 'NONE', #37631, .T. ) ;
#35254=ORIENTED_EDGE ( 'NONE', *, *, #14414, .T. ) ;
#35261=PLANE ( 'NONE',  #98411 ) ;
#35265=DIRECTION ( 'NONE',  ( 0.3595896960900473172, 0.9331105242498700658, 0.000000000000000000 ) ) ;
#35269=ORIENTED_EDGE ( 'NONE', *, *, #42370, .F. ) ;
#35272=CARTESIAN_POINT ( 'NONE',  ( -14.83894680564148238, 24.48641780169620219, -10.00000000000000000 ) ) ;
#35275=CARTESIAN_POINT ( 'NONE',  ( -19.65312891409030271, 93.06504152958497400, -10.00000000000000888 ) ) ;
#35277=AXIS2_PLACEMENT_3D ( 'NONE', #27322, #48109, #72443 ) ;
#35285=VECTOR ( 'NONE', #28401, 1000.000000000000000 ) ;
#35293=AXIS2_PLACEMENT_3D ( 'NONE', #89239, #65370, #57759 ) ;
#35294=CARTESIAN_POINT ( 'NONE',  ( -19.59289307225702714, 92.93664611688882360, 59.99999999999999289 ) ) ;
#35305=DIRECTION ( 'NONE',  ( -1.000000000000000000, 0.000000000000000000, 0.000000000000000000 ) ) ;
#35309=CARTESIAN_POINT ( 'NONE',  ( -19.65312891409030271, 93.06504152958497400, -10.00000000000000888 ) ) ;
#35313=CARTESIAN_POINT ( 'NONE',  ( -61.78156952962572035, 53.28125210322373562, 59.99999999999999289 ) ) ;
#35320=CIRCLE ( 'NONE', #4596, 70.00000000000001421 ) ;
#35322=ORIENTED_EDGE ( 'NONE', *, *, #86050, .T. ) ;
#35326=ORIENTED_EDGE ( 'NONE', *, *, #38266, .T. ) ;
#35327=LINE ( 'NONE', #88103, #85578 ) ;
#35334=DIRECTION ( 'NONE',  ( 1.000000000000000000, 0.000000000000000000, 0.000000000000000000 ) ) ;
#35335=CIRCLE ( 'NONE', #25579, 60.00000000000002132 ) ;
#35336=CIRCLE ( 'NONE', #77357, 70.00000000000001421 ) ;
#35338=LINE ( 'NONE', #12056, #55883 ) ;
#35339=DIRECTION ( 'NONE',  ( -0.9994538543569189137, 0.03304531753666254540, 0.000000000000000000 ) ) ;
#35341=LINE ( 'NONE', #90084, #17327 ) ;
#35345=AXIS2_PLACEMENT_3D ( 'NONE', #75123, #40815, #95090 ) ;
#35351=LINE ( 'NONE', #41445, #24207 ) ;
#35353=CARTESIAN_POINT ( 'NONE',  ( -8.240413327673026700, 41.28378578775782159, 59.99999999999999289 ) ) ;
#35360=ORIENTED_EDGE ( 'NONE', *, *, #78472, .T. ) ;
#35367=ORIENTED_EDGE ( 'NONE', *, *, #40469, .T. ) ;
#35368=DIRECTION ( 'NONE',  ( -0.9662637919863231728, -0.2575544297740022248, 0.000000000000000000 ) ) ;
#35379=ORIENTED_EDGE ( 'NONE', *, *, #74590, .F. ) ;
#35386=FACE_OUTER_BOUND ( 'NONE', #98082, .T. ) ;
#35387=EDGE_CURVE ( 'NONE', #68897, #24506, #988, .T. ) ;
#35397=EDGE_CURVE ( 'NONE', #87650, #76499, #31870, .T. ) ;
#35398=AXIS2_PLACEMENT_3D ( 'NONE', #61563, #68667, #83926 ) ;
#35400=VECTOR ( 'NONE', #66748, 1000.000000000000000 ) ;
#35409=VECTOR ( 'NONE', #70996, 1000.000000000000000 ) ;
#35425=CARTESIAN_POINT ( 'NONE',  ( -70.89022602266993545, 47.22876919346843749, -10.00000000000000000 ) ) ;
#35426=LINE ( 'NONE', #82079, #99113 ) ;
#35433=CARTESIAN_POINT ( 'NONE',  ( 44.18794977381974576, 118.5901545549086791, 10.00000000000000000 ) ) ;
#35438=LINE ( 'NONE', #80593, #10955 ) ;
#35441=ADVANCED_FACE ( 'NONE', ( #10468 ), #72287, .T. ) ;
#35442=ORIENTED_EDGE ( 'NONE', *, *, #65746, .T. ) ;
#35443=FACE_OUTER_BOUND ( 'NONE', #89216, .T. ) ;
#35448=LINE ( 'NONE', #51655, #19843 ) ;
#35457=CARTESIAN_POINT ( 'NONE',  ( -48.47243291925849462, 30.64988553008148031, -10.00000000000000000 ) ) ;
#35458=LINE ( 'NONE', #72499, #94974 ) ;
#35461=CARTESIAN_POINT ( 'NONE',  ( -58.10760318826260118, 36.06970723555269842, 10.00000000000000000 ) ) ;
#35463=ORIENTED_EDGE ( 'NONE', *, *, #71672, .T. ) ;
#35465=VECTOR ( 'NONE', #33578, 1000.000000000000000 ) ;
#35467=CARTESIAN_POINT ( 'NONE',  ( 6.147400554087897540, 72.11620600556240390, -10.00000000000000000 ) ) ;
#35470=AXIS2_PLACEMENT_3D ( 'NONE', #25990, #26132, #33742 ) ;
#35483=DIRECTION ( 'NONE',  ( 0.9086904199442095154, -0.4174706225611763410, 0.000000000000000000 ) ) ;
#35486=ORIENTED_EDGE ( 'NONE', *, *, #1379, .F. ) ;
#35497=CIRCLE ( 'NONE', #97017, 0.1418229129680845801 ) ;
#35501=ORIENTED_EDGE ( 'NONE', *, *, #78238, .F. ) ;
#35504=ORIENTED_EDGE ( 'NONE', *, *, #22277, .T. ) ;
#35509=LINE ( 'NONE', #3634, #54837 ) ;
#35511=CARTESIAN_POINT ( 'NONE',  ( -41.08971556016342674, 38.44550953485882872, 59.99999999999999289 ) ) ;
#35515=CARTESIAN_POINT ( 'NONE',  ( 35.03822396736671152, 49.37458582131906581, 177.5919119679930134 ) ) ;
#35522=DIRECTION ( 'NONE',  ( -0.8660254037844379305, -0.5000000000000011102, -0.000000000000000000 ) ) ;
#35525=EDGE_CURVE ( 'NONE', #34934, #65613, #33771, .T. ) ;
#35534=ORIENTED_EDGE ( 'NONE', *, *, #97146, .F. ) ;
#35535=VECTOR ( 'NONE', #38828, 1000.000000000000000 ) ;
#35536=DIRECTION ( 'NONE',  ( -1.000000000000000000, 0.000000000000000000, 0.000000000000000000 ) ) ;
#35551=AXIS2_PLACEMENT_3D ( 'NONE', #69161, #67680, #22573 ) ;
#35552=EDGE_CURVE ( 'NONE', #98479, #1989, #77758, .T. ) ;
#35570=CIRCLE ( 'NONE', #1603, 60.00000000000002132 ) ;
#35577=CARTESIAN_POINT ( 'NONE',  ( -66.34925969370661392, 42.61035540433362456, -10.00000000000000000 ) ) ;
#35578=LINE ( 'NONE', #20392, #95004 ) ;
#35579=AXIS2_PLACEMENT_3D ( 'NONE', #39993, #15705, #62296 ) ;
#35585=EDGE_LOOP ( 'NONE', ( #34929, #9977, #93689, #43403 ) ) ;
#35586=ORIENTED_EDGE ( 'NONE', *, *, #54717, .F. ) ;
#35590=VERTEX_POINT ( 'NONE', #24530 ) ;
#35594=LINE ( 'NONE', #74624, #79911 ) ;
#35605=CARTESIAN_POINT ( 'NONE',  ( 7.454216751344177716, 28.24511763804003195, 10.00000000000000000 ) ) ;
#35613=CARTESIAN_POINT ( 'NONE',  ( -54.21831688459419496, 33.63902229265145394, -10.00000000000000000 ) ) ;
#35615=DIRECTION ( 'NONE',  ( 0.02977611660965746518, -0.9995565931350001154, 0.000000000000000000 ) ) ;
#35616=ORIENTED_EDGE ( 'NONE', *, *, #10119, .F. ) ;
#35617=CARTESIAN_POINT ( 'NONE',  ( -7.136131074307646927, 62.27793715567937483, -10.00000000000000000 ) ) ;
#35632=ORIENTED_EDGE ( 'NONE', *, *, #95995, .T. ) ;
#35634=LINE ( 'NONE', #29532, #19316 ) ;
#35641=LINE ( 'NONE', #59412, #67506 ) ;
#35653=LINE ( 'NONE', #88935, #27335 ) ;
#35669=CARTESIAN_POINT ( 'NONE',  ( 37.48526053816526371, 54.83666944042808922, -10.00000000000000000 ) ) ;
#35671=CARTESIAN_POINT ( 'NONE',  ( 49.74924850768368145, 83.93760989710258968, 10.00000000000000000 ) ) ;
#35676=CARTESIAN_POINT ( 'NONE',  ( 47.96820964746023463, 80.67316705762479501, -10.00000000000000000 ) ) ;
#35678=CARTESIAN_POINT ( 'NONE',  ( 24.46206622376873696, 38.38158625946101665, 10.00000000000000000 ) ) ;
#35685=CARTESIAN_POINT ( 'NONE',  ( -50.34886203176066033, 29.86533669878861375, -10.00000000000000000 ) ) ;
#35700=DIRECTION ( 'NONE',  ( -0.4621356007560455392, 0.8868092729070039537, 0.000000000000000000 ) ) ;
#35703=AXIS2_PLACEMENT_3D ( 'NONE', #29601, #91432, #56881 ) ;
#35708=VERTEX_POINT ( 'NONE', #45699 ) ;
#35709=CARTESIAN_POINT ( 'NONE',  ( -59.84120265028303010, 60.49048082395207615, 59.99999999999999289 ) ) ;
#35716=EDGE_LOOP ( 'NONE', ( #56426, #81490, #33041, #89503 ) ) ;
#35722=VERTEX_POINT ( 'NONE', #13824 ) ;
#35725=VERTEX_POINT ( 'NONE', #60399 ) ;
#35729=ORIENTED_EDGE ( 'NONE', *, *, #65876, .T. ) ;
#35732=VERTEX_POINT ( 'NONE', #87793 ) ;
#35741=ORIENTED_EDGE ( 'NONE', *, *, #50984, .F. ) ;
#35744=ORIENTED_EDGE ( 'NONE', *, *, #53336, .T. ) ;
#35745=DIRECTION ( 'NONE',  ( -0.9825427565607363078, 0.1860369090530955005, 0.000000000000000000 ) ) ;
#35748=DIRECTION ( 'NONE',  ( 1.000000000000000000, 0.000000000000000000, 0.000000000000000000 ) ) ;
#35753=CARTESIAN_POINT ( 'NONE',  ( 41.50249547274756168, 124.4848494355456836, -10.00000000000000000 ) ) ;
#35754=DIRECTION ( 'NONE',  ( 1.000000000000000000, 0.000000000000000000, 0.000000000000000000 ) ) ;
#35766=LINE ( 'NONE', #79917, #89014 ) ;
#35768=CYLINDRICAL_SURFACE ( 'NONE', #96448, 70.00000000000002842 ) ;
#35770=ORIENTED_EDGE ( 'NONE', *, *, #73409, .F. ) ;
#35771=LINE ( 'NONE', #43857, #100147 ) ;
#35773=EDGE_CURVE ( 'NONE', #8702, #29478, #93863, .T. ) ;
#35778=AXIS2_PLACEMENT_3D ( 'NONE', #46050, #60252, #6586 ) ;
#35783=DIRECTION ( 'NONE',  ( -0.4272584830711198545, -0.9041295198387040433, 0.000000000000000000 ) ) ;
#35794=CARTESIAN_POINT ( 'NONE',  ( -51.75017079496729622, 30.85748650210271293, 10.00000000000000000 ) ) ;
#35795=EDGE_CURVE ( 'NONE', #15777, #23431, #82161, .T. ) ;
#35796=DIRECTION ( 'NONE',  ( -1.000000000000000000, 0.000000000000000000, 0.000000000000000000 ) ) ;
#35805=DIRECTION ( 'NONE',  ( -0.5078630399532132467, -0.8614378286617561109, 0.000000000000000000 ) ) ;
#35809=VERTEX_POINT ( 'NONE', #66901 ) ;
#35811=CARTESIAN_POINT ( 'NONE',  ( -76.49344163160110099, 52.20945622995200353, -10.00000000000000000 ) ) ;
#35814=ORIENTED_EDGE ( 'NONE', *, *, #27330, .F. ) ;
#35816=CARTESIAN_POINT ( 'NONE',  ( -79.43448886220070904, 56.15136215343108717, 10.00000000000000000 ) ) ;
#35818=DIRECTION ( 'NONE',  ( 1.000000000000000000, 0.000000000000000000, 0.000000000000000000 ) ) ;
#35836=EDGE_CURVE ( 'NONE', #72480, #22609, #35509, .T. ) ;
#35842=ORIENTED_EDGE ( 'NONE', *, *, #88198, .T. ) ;
#35867=ORIENTED_EDGE ( 'NONE', *, *, #20698, .F. ) ;
#35869=VERTEX_POINT ( 'NONE', #57802 ) ;
#35873=LINE ( 'NONE', #5483, #24123 ) ;
#35876=FACE_OUTER_BOUND ( 'NONE', #35230, .T. ) ;
#35887=DIRECTION ( 'NONE',  ( -0.7490285521785782219, 0.6625377181876236365, 0.000000000000000000 ) ) ;
#35895=EDGE_CURVE ( 'NONE', #72875, #49563, #37976, .T. ) ;
#35896=CARTESIAN_POINT ( 'NONE',  ( 46.22371820283660782, 112.7232458147606451, -10.00000000000000000 ) ) ;
#35906=VERTEX_POINT ( 'NONE', #6103 ) ;
#35917=CARTESIAN_POINT ( 'NONE',  ( -6.175261138941928962, 62.68629713672868320, -10.00000000000000000 ) ) ;
#35929=ORIENTED_EDGE ( 'NONE', *, *, #53379, .F. ) ;
#35933=ORIENTED_EDGE ( 'NONE', *, *, #42865, .F. ) ;
#35936=CYLINDRICAL_SURFACE ( 'NONE', #23295, 70.00000000000002842 ) ;
#35945=DIRECTION ( 'NONE',  ( -1.000000000000000000, 0.000000000000000000, 0.000000000000000000 ) ) ;
#35947=CARTESIAN_POINT ( 'NONE',  ( -19.65312891409030271, 93.06504152958497400, 60.00000000000000000 ) ) ;
#35950=CARTESIAN_POINT ( 'NONE',  ( 24.94106359012611307, 66.84403333601011354, 59.99999999999999289 ) ) ;
#35952=ORIENTED_EDGE ( 'NONE', *, *, #80742, .F. ) ;
#35955=CARTESIAN_POINT ( 'NONE',  ( 47.46694519036043403, 73.19305994210745325, 10.00000000000000000 ) ) ;
#35956=VERTEX_POINT ( 'NONE', #31388 ) ;
#35965=DIRECTION ( 'NONE',  ( -0.8492021815265757834, 0.5280678506503729830, 0.000000000000000000 ) ) ;
#35967=EDGE_LOOP ( 'NONE', ( #15127, #81972, #84813, #34819 ) ) ;
#35981=ORIENTED_EDGE ( 'NONE', *, *, #72576, .F. ) ;
#35982=FACE_OUTER_BOUND ( 'NONE', #92992, .T. ) ;
#35985=DIRECTION ( 'NONE',  ( -0.2197389712097134185, -0.9755587037855265597, 0.000000000000000000 ) ) ;
#35989=EDGE_LOOP ( 'NONE', ( #84137, #11550, #51942, #75272 ) ) ;
#36000=ORIENTED_EDGE ( 'NONE', *, *, #66927, .F. ) ;
#36007=ADVANCED_FACE ( 'NONE', ( #16198 ), #8602, .F. ) ;
#36023=AXIS2_PLACEMENT_3D ( 'NONE', #43210, #3264, #49836 ) ;
#36045=CARTESIAN_POINT ( 'NONE',  ( -56.29836151245349640, 34.88994676555962116, -10.00000000000000000 ) ) ;
#36054=DIRECTION ( 'NONE',  ( 1.000000000000000000, 0.000000000000000000, 0.000000000000000000 ) ) ;
#36058=DIRECTION ( 'NONE',  ( -0.000000000000000000, -0.000000000000000000, -1.000000000000000000 ) ) ;
#36078=ORIENTED_EDGE ( 'NONE', *, *, #60759, .F. ) ;
#36083=CARTESIAN_POINT ( 'NONE',  ( 30.83629047462941486, 109.2621690313456924, 59.99999999999999289 ) ) ;
#36088=ORIENTED_EDGE ( 'NONE', *, *, #98481, .T. ) ;
#36089=EDGE_CURVE ( 'NONE', #41047, #90969, #96739, .T. ) ;
#36094=ORIENTED_EDGE ( 'NONE', *, *, #56933, .T. ) ;
#36098=DIRECTION ( 'NONE',  ( 0.000000000000000000, 0.000000000000000000, 1.000000000000000000 ) ) ;
#36111=ADVANCED_FACE ( 'NONE', ( #35386 ), #26306, .T. ) ;
#36116=DIRECTION ( 'NONE',  ( -0.000000000000000000, 0.000000000000000000, -1.000000000000000000 ) ) ;
#36126=ADVANCED_FACE ( 'NONE', ( #41480 ), #50096, .F. ) ;
#36131=DIRECTION ( 'NONE',  ( -0.9522021074858073586, -0.3054687324417786343, 0.000000000000000000 ) ) ;
#36132=ORIENTED_EDGE ( 'NONE', *, *, #32635, .T. ) ;
#36133=DIRECTION ( 'NONE',  ( 0.000000000000000000, 0.000000000000000000, 1.000000000000000000 ) ) ;
#36134=EDGE_CURVE ( 'NONE', #67607, #87878, #77506, .T. ) ;
#36145=VERTEX_POINT ( 'NONE', #80544 ) ;
#36162=DIRECTION ( 'NONE',  ( -0.000000000000000000, -0.000000000000000000, -1.000000000000000000 ) ) ;
#36173=ORIENTED_EDGE ( 'NONE', *, *, #70539, .T. ) ;
#36179=ORIENTED_EDGE ( 'NONE', *, *, #62011, .T. ) ;
#36190=DIRECTION ( 'NONE',  ( -0.4621356007560455392, 0.8868092729070038427, 0.000000000000000000 ) ) ;
#36208=VERTEX_POINT ( 'NONE', #19717 ) ;
#36210=ORIENTED_EDGE ( 'NONE', *, *, #93638, .F. ) ;
#36213=EDGE_CURVE ( 'NONE', #4429, #23644, #96237, .T. ) ;
#36226=ORIENTED_EDGE ( 'NONE', *, *, #14543, .F. ) ;
#36242=ORIENTED_EDGE ( 'NONE', *, *, #85069, .F. ) ;
#36251=CARTESIAN_POINT ( 'NONE',  ( 32.30839531297598910, 123.0650415295850593, -40.00000000000000000 ) ) ;
#36258=EDGE_CURVE ( 'NONE', #47682, #17413, #87675, .T. ) ;
#36261=ORIENTED_EDGE ( 'NONE', *, *, #71633, .F. ) ;
#36262=LINE ( 'NONE', #92015, #53257 ) ;
#36276=DIRECTION ( 'NONE',  ( -0.000000000000000000, -0.000000000000000000, -1.000000000000000000 ) ) ;
#36278=DIRECTION ( 'NONE',  ( 0.000000000000000000, 0.000000000000000000, 1.000000000000000000 ) ) ;
#36281=FACE_OUTER_BOUND ( 'NONE', #54374, .T. ) ;
#36296=CARTESIAN_POINT ( 'NONE',  ( -55.59287931351116896, 32.99562883703961802, 177.5919119679930134 ) ) ;
#36301=CARTESIAN_POINT ( 'NONE',  ( 44.47956695515382108, 64.36960560548604349, 10.00000000000000000 ) ) ;
#36304=ORIENTED_EDGE ( 'NONE', *, *, #28127, .T. ) ;
#36314=VERTEX_POINT ( 'NONE', #13598 ) ;
#36317=VERTEX_POINT ( 'NONE', #5987 ) ;
#36319=AXIS2_PLACEMENT_3D ( 'NONE', #4031, #58223, #12140 ) ;
#36320=ORIENTED_EDGE ( 'NONE', *, *, #96297, .F. ) ;
#36321=EDGE_CURVE ( 'NONE', #28659, #98547, #99199, .T. ) ;
#36327=DIRECTION ( 'NONE',  ( 0.8806841296921896767, -0.4737039832092512226, 0.000000000000000000 ) ) ;
#36330=FACE_OUTER_BOUND ( 'NONE', #66983, .T. ) ;
#36348=FACE_OUTER_BOUND ( 'NONE', #97045, .T. ) ;
#36357=LINE ( 'NONE', #67262, #72275 ) ;
#36359=EDGE_LOOP ( 'NONE', ( #27517, #82606, #8270, #58657 ) ) ;
#36362=ORIENTED_EDGE ( 'NONE', *, *, #70999, .F. ) ;
#36369=VERTEX_POINT ( 'NONE', #43970 ) ;
#36375=CARTESIAN_POINT ( 'NONE',  ( 48.48788556946983874, 102.1758113618167982, -10.00000000000000000 ) ) ;
#36377=VECTOR ( 'NONE', #79656, 1000.000000000000227 ) ;
#36378=FACE_OUTER_BOUND ( 'NONE', #79743, .T. ) ;
#36386=CIRCLE ( 'NONE', #94645, 0.1418229129681557177 ) ;
#36393=DIRECTION ( 'NONE',  ( 1.000000000000000000, 0.000000000000000000, -0.000000000000000000 ) ) ;
#36394=DIRECTION ( 'NONE',  ( 1.000000000000000000, 7.137148015447434001E-15, 0.000000000000000000 ) ) ;
#36405=AXIS2_PLACEMENT_3D ( 'NONE', #62461, #93427, #23979 ) ;
#36408=DIRECTION ( 'NONE',  ( 0.000000000000000000, -0.000000000000000000, 1.000000000000000000 ) ) ;
#36421=ORIENTED_EDGE ( 'NONE', *, *, #53266, .F. ) ;
#36429=DIRECTION ( 'NONE',  ( -0.000000000000000000, -0.000000000000000000, -1.000000000000000000 ) ) ;
#36431=CARTESIAN_POINT ( 'NONE',  ( 39.77289032284285497, 58.49985355908045648, 10.00000000000000000 ) ) ;
#36445=CIRCLE ( 'NONE', #93106, 0.1418229129681522482 ) ;
#36454=DIRECTION ( 'NONE',  ( -0.7278481391575704063, 0.6857383512133925496, 0.000000000000000000 ) ) ;
#36464=ORIENTED_EDGE ( 'NONE', *, *, #43884, .F. ) ;
#36465=DIRECTION ( 'NONE',  ( -0.000000000000000000, 0.000000000000000000, -1.000000000000000000 ) ) ;
#36466=VERTEX_POINT ( 'NONE', #63679 ) ;
#36467=ORIENTED_EDGE ( 'NONE', *, *, #61621, .F. ) ;
#36469=CARTESIAN_POINT ( 'NONE',  ( -59.29375005653867703, 35.37083770076973366, 10.00000000000000000 ) ) ;
#36472=FACE_OUTER_BOUND ( 'NONE', #80606, .T. ) ;
#36480=ORIENTED_EDGE ( 'NONE', *, *, #77420, .F. ) ;
#36488=VECTOR ( 'NONE', #49841, 1000.000000000000000 ) ;
#36491=ORIENTED_EDGE ( 'NONE', *, *, #6397, .T. ) ;
#36498=AXIS2_PLACEMENT_3D ( 'NONE', #97822, #19819, #51712 ) ;
#36500=CARTESIAN_POINT ( 'NONE',  ( 6.752405126987250483, 41.48691455871444589, 59.99999999999999289 ) ) ;
#36501=VERTEX_POINT ( 'NONE', #8977 ) ;
#36507=DIRECTION ( 'NONE',  ( -0.000000000000000000, -0.000000000000000000, -1.000000000000000000 ) ) ;
#36515=CARTESIAN_POINT ( 'NONE',  ( -68.37628875030422648, 42.44405361048389125, 10.00000000000000000 ) ) ;
#36521=ORIENTED_EDGE ( 'NONE', *, *, #25003, .T. ) ;
#36528=CARTESIAN_POINT ( 'NONE',  ( -58.10760318826260118, 36.06970723555269842, -10.00000000000000000 ) ) ;
#36530=CARTESIAN_POINT ( 'NONE',  ( 24.55112987542764458, 40.41347472807389352, -10.00000000000000000 ) ) ;
#36558=DIRECTION ( 'NONE',  ( -0.000000000000000000, -0.000000000000000000, -1.000000000000000000 ) ) ;
#36559=ORIENTED_EDGE ( 'NONE', *, *, #87110, .T. ) ;
#36576=EDGE_CURVE ( 'NONE', #79632, #21527, #89058, .T. ) ;
#36578=VERTEX_POINT ( 'NONE', #57566 ) ;
#36580=AXIS2_PLACEMENT_3D ( 'NONE', #90739, #22278, #14685 ) ;
#36589=VECTOR ( 'NONE', #71923, 1000.000000000000114 ) ;
#36602=LINE ( 'NONE', #66025, #97988 ) ;
#36607=ORIENTED_EDGE ( 'NONE', *, *, #18318, .F. ) ;
#36621=LINE ( 'NONE', #21929, #17326 ) ;
#36625=VECTOR ( 'NONE', #82373, 1000.000000000000114 ) ;
#36626=ADVANCED_FACE ( 'NONE', ( #97125 ), #57066, .F. ) ;
#36627=PLANE ( 'NONE',  #31652 ) ;
#36628=AXIS2_PLACEMENT_3D ( 'NONE', #26162, #18570, #89511 ) ;
#36636=EDGE_CURVE ( 'NONE', #39677, #14660, #41364, .T. ) ;
#36647=VECTOR ( 'NONE', #93080, 1000.000000000000114 ) ;
#36657=VECTOR ( 'NONE', #65263, 1000.000000000000227 ) ;
#36674=ORIENTED_EDGE ( 'NONE', *, *, #72032, .F. ) ;
#36677=EDGE_CURVE ( 'NONE', #30899, #11943, #34280, .T. ) ;
#36689=CARTESIAN_POINT ( 'NONE',  ( 42.76202708541288899, 64.24573752441608576, 10.00000000000000000 ) ) ;
#36694=EDGE_CURVE ( 'NONE', #27723, #87428, #90013, .T. ) ;
#36698=ORIENTED_EDGE ( 'NONE', *, *, #393, .T. ) ;
#36704=CARTESIAN_POINT ( 'NONE',  ( -19.65312891409030271, 93.06504152958497400, -10.00000000000000888 ) ) ;
#36708=ORIENTED_EDGE ( 'NONE', *, *, #62706, .F. ) ;
#36715=ORIENTED_EDGE ( 'NONE', *, *, #49270, .F. ) ;
#36718=CARTESIAN_POINT ( 'NONE',  ( 49.10122569834316408, 93.29622288527660601, 10.00000000000000000 ) ) ;
#36719=CARTESIAN_POINT ( 'NONE',  ( 45.19716250472275476, 70.24742367233086782, -10.00000000000000000 ) ) ;
#36729=ORIENTED_EDGE ( 'NONE', *, *, #62706, .T. ) ;
#36730=AXIS2_PLACEMENT_3D ( 'NONE', #17307, #86771, #79658 ) ;
#36742=VERTEX_POINT ( 'NONE', #98088 ) ;
#36746=LINE ( 'NONE', #22551, #72968 ) ;
#36752=EDGE_CURVE ( 'NONE', #1290, #76499, #97605, .T. ) ;
#36757=CARTESIAN_POINT ( 'NONE',  ( -19.65312891409030271, 93.06504152958497400, 10.00000000000000888 ) ) ;
#36771=VECTOR ( 'NONE', #69676, 1000.000000000000000 ) ;
#36773=VECTOR ( 'NONE', #70859, 1000.000000000000114 ) ;
#36799=CIRCLE ( 'NONE', #28711, 0.1418229129680828593 ) ;
#36800=DIRECTION ( 'NONE',  ( -1.000000000000000000, 1.957058632818291033E-13, 0.000000000000000000 ) ) ;
#36811=VECTOR ( 'NONE', #72091, 1000.000000000000000 ) ;
#36812=ORIENTED_EDGE ( 'NONE', *, *, #88511, .T. ) ;
#36815=DIRECTION ( 'NONE',  ( -0.5078630399532131356, -0.8614378286617561109, 0.000000000000000000 ) ) ;
#36819=EDGE_CURVE ( 'NONE', #76358, #10367, #43489, .T. ) ;
#36828=EDGE_CURVE ( 'NONE', #51434, #76991, #72451, .T. ) ;
#36836=VERTEX_POINT ( 'NONE', #7625 ) ;
#36841=CARTESIAN_POINT ( 'NONE',  ( -19.65312891409030271, 93.06504152958497400, 10.00000000000000888 ) ) ;
#36853=VECTOR ( 'NONE', #53188, 1000.000000000000114 ) ;
#36855=AXIS2_PLACEMENT_3D ( 'NONE', #55224, #30943, #8648 ) ;
#36862=VERTEX_POINT ( 'NONE', #94642 ) ;
#36863=AXIS2_PLACEMENT_3D ( 'NONE', #99458, #76171, #70025 ) ;
#36866=LINE ( 'NONE', #59655, #12363 ) ;
#36868=VECTOR ( 'NONE', #86722, 1000.000000000000000 ) ;
#36890=LINE ( 'NONE', #85545, #59194 ) ;
#36904=DIRECTION ( 'NONE',  ( -0.000000000000000000, 0.000000000000000000, -1.000000000000000000 ) ) ;
#36911=DIRECTION ( 'NONE',  ( 0.2803049773603250028, -0.9599109957006575211, 0.000000000000000000 ) ) ;
#36924=EDGE_CURVE ( 'NONE', #89008, #47179, #85411, .T. ) ;
#36930=CARTESIAN_POINT ( 'NONE',  ( 17.00529913897481293, 33.43149683636511327, 10.00000000000000000 ) ) ;
#36933=VECTOR ( 'NONE', #52318, 1000.000000000000114 ) ;
#36935=LINE ( 'NONE', #13165, #37810 ) ;
#36937=EDGE_CURVE ( 'NONE', #84233, #94567, #65689, .T. ) ;
#36938=LINE ( 'NONE', #5546, #52444 ) ;
#36964=CARTESIAN_POINT ( 'NONE',  ( -19.34860767484687116, 59.83210158341513818, -10.00000000000000000 ) ) ;
#36966=ORIENTED_EDGE ( 'NONE', *, *, #97182, .T. ) ;
#36969=VERTEX_POINT ( 'NONE', #98111 ) ;
#36971=DIRECTION ( 'NONE',  ( 1.000000000000000000, 0.000000000000000000, 0.000000000000000000 ) ) ;
#36982=CIRCLE ( 'NONE', #30473, 70.00000000000001421 ) ;
#36984=LINE ( 'NONE', #34986, #32359 ) ;
#36985=EDGE_CURVE ( 'NONE', #24595, #45905, #28694, .T. ) ;
#36994=EDGE_LOOP ( 'NONE', ( #41042, #98761, #67235, #64032 ) ) ;
#37000=ORIENTED_EDGE ( 'NONE', *, *, #83628, .T. ) ;
#37001=PLANE ( 'NONE',  #8948 ) ;
#37006=CARTESIAN_POINT ( 'NONE',  ( 49.19475937879462890, 79.05079877653317055, 10.00000000000000000 ) ) ;
#37010=VECTOR ( 'NONE', #41000, 1000.000000000000114 ) ;
#37015=DIRECTION ( 'NONE',  ( 1.000000000000000000, 0.000000000000000000, 0.000000000000000000 ) ) ;
#37019=ADVANCED_FACE ( 'NONE', ( #57588 ), #88567, .T. ) ;
#37033=DIRECTION ( 'NONE',  ( -0.000000000000000000, -0.000000000000000000, 1.000000000000000000 ) ) ;
#37042=AXIS2_PLACEMENT_3D ( 'NONE', #79793, #80803, #9869 ) ;
#37060=VECTOR ( 'NONE', #23031, 1000.000000000000114 ) ;
#37062=CARTESIAN_POINT ( 'NONE',  ( 41.37327796571899796, 124.7191351846657028, -10.00000000000000000 ) ) ;
#37068=CARTESIAN_POINT ( 'NONE',  ( 10.06845959268932411, 31.07446838803122446, -10.00000000000000000 ) ) ;
#37071=VECTOR ( 'NONE', #48672, 1000.000000000000114 ) ;
#37072=VERTEX_POINT ( 'NONE', #7898 ) ;
#37083=VERTEX_POINT ( 'NONE', #84428 ) ;
#37089=EDGE_LOOP ( 'NONE', ( #10339, #95178, #76860, #3392 ) ) ;
#37090=CARTESIAN_POINT ( 'NONE',  ( -14.16662337007866057, 72.61341060738401154, 13.96608703042485011 ) ) ;
#37093=DIRECTION ( 'NONE',  ( 0.000000000000000000, -0.000000000000000000, 1.000000000000000000 ) ) ;
#37094=ORIENTED_EDGE ( 'NONE', *, *, #85187, .F. ) ;
#37095=EDGE_LOOP ( 'NONE', ( #50077, #3748, #90836, #92733 ) ) ;
#37104=CARTESIAN_POINT ( 'NONE',  ( 45.57373283677818421, 114.7827874512443032, -10.00000000000000000 ) ) ;
#37106=CARTESIAN_POINT ( 'NONE',  ( -19.55550329252533004, 92.96216793405713474, 59.99999999999999289 ) ) ;
#37108=FACE_OUTER_BOUND ( 'NONE', #9553, .T. ) ;
#37109=LINE ( 'NONE', #41849, #31726 ) ;
#37124=DIRECTION ( 'NONE',  ( -1.000000000000000000, 0.000000000000000000, 0.000000000000000000 ) ) ;
#37125=AXIS2_PLACEMENT_3D ( 'NONE', #55960, #95554, #79340 ) ;
#37131=VECTOR ( 'NONE', #11147, 1000.000000000000000 ) ;
#37135=ADVANCED_FACE ( 'NONE', ( #22087 ), #85434, .F. ) ;
#37141=CIRCLE ( 'NONE', #41995, 0.1418229129680863287 ) ;
#37149=ADVANCED_FACE ( 'NONE', ( #41774, #47863 ), #56969, .F. ) ;
#37152=VECTOR ( 'NONE', #38554, 1000.000000000000000 ) ;
#37165=EDGE_LOOP ( 'NONE', ( #61586, #96612, #2614, #90050 ) ) ;
#37170=DIRECTION ( 'NONE',  ( 0.8035972437015812542, 0.5951734788405995680, 0.000000000000000000 ) ) ;
#37177=CARTESIAN_POINT ( 'NONE',  ( -75.69529296620470404, 50.68926341652933587, 10.00000000000000000 ) ) ;
#37178=SHAPE_REPRESENTATION_RELATIONSHIP ( 'NONE' , 'NONE' ,  #78010, #484 ) ;
#37179=DIRECTION ( 'NONE',  ( -0.6835488936653838499, -0.7299047266382303611, 0.000000000000000000 ) ) ;
#37194=VERTEX_POINT ( 'NONE', #25593 ) ;
#37215=EDGE_CURVE ( 'NONE', #76961, #46907, #41265, .T. ) ;
#37217=VECTOR ( 'NONE', #75791, 1000.000000000000227 ) ;
#37218=ORIENTED_EDGE ( 'NONE', *, *, #36321, .F. ) ;
#37226=ORIENTED_EDGE ( 'NONE', *, *, #33570, .F. ) ;
#37229=ORIENTED_EDGE ( 'NONE', *, *, #80178, .T. ) ;
#37256=CYLINDRICAL_SURFACE ( 'NONE', #71151, 70.00000000000002842 ) ;
#37258=EDGE_CURVE ( 'NONE', #15783, #2857, #16972, .T. ) ;
#37262=DIRECTION ( 'NONE',  ( 0.000000000000000000, 0.000000000000000000, 1.000000000000000000 ) ) ;
#37263=LINE ( 'NONE', #69654, #41831 ) ;
#37272=CYLINDRICAL_SURFACE ( 'NONE', #8091, 70.00000000000002842 ) ;
#37280=DIRECTION ( 'NONE',  ( 0.000000000000000000, 0.000000000000000000, 1.000000000000000000 ) ) ;
#37282=LINE ( 'NONE', #13510, #19022 ) ;
#37292=CARTESIAN_POINT ( 'NONE',  ( 32.06670334149083601, 91.95954910241374591, 59.99999999999999289 ) ) ;
#37295=DIRECTION ( 'NONE',  ( -0.9689225787001356505, 0.2473641778533816060, 0.000000000000000000 ) ) ;
#37307=ORIENTED_EDGE ( 'NONE', *, *, #60113, .F. ) ;
#37322=EDGE_CURVE ( 'NONE', #5467, #46146, #72720, .T. ) ;
#37323=FACE_OUTER_BOUND ( 'NONE', #77447, .T. ) ;
#37326=ORIENTED_EDGE ( 'NONE', *, *, #53502, .T. ) ;
#37329=DIRECTION ( 'NONE',  ( -0.1266907948509198856, 0.9919422576440839467, 0.000000000000000000 ) ) ;
#37331=LINE ( 'NONE', #53034, #57837 ) ;
#37336=EDGE_CURVE ( 'NONE', #39956, #76681, #66579, .T. ) ;
#37341=DIRECTION ( 'NONE',  ( -1.000000000000000000, 0.000000000000000000, 0.000000000000000000 ) ) ;
#37356=DIRECTION ( 'NONE',  ( -0.7561390817803280706, 0.6544109481086042290, 0.000000000000000000 ) ) ;
#37360=CYLINDRICAL_SURFACE ( 'NONE', #18728, 70.00000000000002842 ) ;
#37363=DIRECTION ( 'NONE',  ( -0.000000000000000000, -0.000000000000000000, -1.000000000000000000 ) ) ;
#37367=DIRECTION ( 'NONE',  ( 0.9909246428798906825, 0.1344185706417126980, 0.000000000000000000 ) ) ;
#37369=DIRECTION ( 'NONE',  ( 0.000000000000000000, -0.000000000000000000, 1.000000000000000000 ) ) ;
#37373=CARTESIAN_POINT ( 'NONE',  ( -19.62009469743497547, 92.92711952563814748, 59.99999999999999289 ) ) ;
#37386=CARTESIAN_POINT ( 'NONE',  ( -48.36978223816941380, 29.22654356899180428, -10.00000000000000000 ) ) ;
#37387=EDGE_CURVE ( 'NONE', #7863, #67877, #42758, .T. ) ;
#37389=EDGE_CURVE ( 'NONE', #94453, #13198, #44993, .T. ) ;
#37395=CARTESIAN_POINT ( 'NONE',  ( 41.82599275875796252, 62.29945068332010294, -10.00000000000000000 ) ) ;
#37415=VERTEX_POINT ( 'NONE', #90430 ) ;
#37421=VERTEX_POINT ( 'NONE', #34190 ) ;
#37427=ORIENTED_EDGE ( 'NONE', *, *, #49998, .T. ) ;
#37435=ORIENTED_EDGE ( 'NONE', *, *, #91802, .F. ) ;
#37446=ADVANCED_FACE ( 'NONE', ( #96032 ), #21002, .F. ) ;
#37453=ORIENTED_EDGE ( 'NONE', *, *, #32642, .F. ) ;
#37455=VERTEX_POINT ( 'NONE', #82824 ) ;
#37457=FACE_BOUND ( 'NONE', #99669, .T. ) ;
#37460=ADVANCED_FACE ( 'NONE', ( #35173 ), #73690, .T. ) ;
#37469=CARTESIAN_POINT ( 'NONE',  ( -42.23460334637721303, 26.80738527414552408, -10.00000000000000000 ) ) ;
#37490=PLANE ( 'NONE',  #49517 ) ;
#37495=ORIENTED_EDGE ( 'NONE', *, *, #38725, .T. ) ;
#37497=EDGE_CURVE ( 'NONE', #36578, #33337, #55345, .T. ) ;
#37505=FACE_OUTER_BOUND ( 'NONE', #98565, .T. ) ;
#37511=LINE ( 'NONE', #7619, #75774 ) ;
#37512=ORIENTED_EDGE ( 'NONE', *, *, #33121, .F. ) ;
#37529=VECTOR ( 'NONE', #94397, 1000.000000000000000 ) ;
#37540=DIRECTION ( 'NONE',  ( -1.000000000000000000, 0.000000000000000000, 0.000000000000000000 ) ) ;
#37545=ORIENTED_EDGE ( 'NONE', *, *, #3970, .F. ) ;
#37547=DIRECTION ( 'NONE',  ( -0.9171038997749370036, 0.3986482622784180418, 0.000000000000000000 ) ) ;
#37560=CARTESIAN_POINT ( 'NONE',  ( -44.38014153532155603, 70.85927927110010671, -10.00000000000000000 ) ) ;
#37562=DIRECTION ( 'NONE',  ( -0.9662637919863231728, -0.2575544297740022248, 0.000000000000000000 ) ) ;
#37565=EDGE_CURVE ( 'NONE', #75006, #30838, #82241, .T. ) ;
#37567=VERTEX_POINT ( 'NONE', #49763 ) ;
#37570=EDGE_LOOP ( 'NONE', ( #54832, #33728, #95801, #62341 ) ) ;
#37572=DIRECTION ( 'NONE',  ( -0.5076330711061851630, 0.8615733660689046669, 0.000000000000000000 ) ) ;
#37575=CARTESIAN_POINT ( 'NONE',  ( -11.85091256637315205, 72.02634106223788990, 14.52565316431220133 ) ) ;
#37578=CARTESIAN_POINT ( 'NONE',  ( -38.02969130575858259, 25.52022711230254970, -10.00000000000000000 ) ) ;
#37579=ORIENTED_EDGE ( 'NONE', *, *, #40345, .T. ) ;
#37591=LINE ( 'NONE', #70499, #10629 ) ;
#37592=VECTOR ( 'NONE', #97519, 1000.000000000000000 ) ;
#37594=DIRECTION ( 'NONE',  ( -0.9999580202055560196, -0.009162850352621043637, 0.000000000000000000 ) ) ;
#37599=ORIENTED_EDGE ( 'NONE', *, *, #72286, .T. ) ;
#37607=ORIENTED_EDGE ( 'NONE', *, *, #75240, .F. ) ;
#37614=DIRECTION ( 'NONE',  ( -0.000000000000000000, 0.000000000000000000, 1.000000000000000000 ) ) ;
#37620=CARTESIAN_POINT ( 'NONE',  ( -36.52772323645827868, 26.41323893245353105, -10.00000000000000000 ) ) ;
#37624=EDGE_CURVE ( 'NONE', #9798, #1235, #12272, .T. ) ;
#37626=CARTESIAN_POINT ( 'NONE',  ( -78.94662368502557115, 55.85910816071122298, 177.5919119679930134 ) ) ;
#37629=DIRECTION ( 'NONE',  ( 0.000000000000000000, 0.000000000000000000, 1.000000000000000000 ) ) ;
#37631=EDGE_LOOP ( 'NONE', ( #86985, #36362, #95544, #48450 ) ) ;
#37655=LINE ( 'NONE', #68565, #93755 ) ;
#37656=CARTESIAN_POINT ( 'NONE',  ( -10.08900441837308470, 61.23661786014601205, -10.00000000000000000 ) ) ;
#37667=ORIENTED_EDGE ( 'NONE', *, *, #9039, .F. ) ;
#37670=AXIS2_PLACEMENT_3D ( 'NONE', #25706, #55076, #24687 ) ;
#37684=EDGE_LOOP ( 'NONE', ( #28302, #13730, #36210, #67331 ) ) ;
#37685=FACE_OUTER_BOUND ( 'NONE', #97545, .T. ) ;
#37691=ORIENTED_EDGE ( 'NONE', *, *, #44686, .T. ) ;
#37699=EDGE_CURVE ( 'NONE', #3834, #61894, #69437, .T. ) ;
#37701=DIRECTION ( 'NONE',  ( -0.000000000000000000, -0.000000000000000000, -1.000000000000000000 ) ) ;
#37703=EDGE_CURVE ( 'NONE', #19444, #56880, #43347, .T. ) ;
#37712=ORIENTED_EDGE ( 'NONE', *, *, #6598, .F. ) ;
#37715=DIRECTION ( 'NONE',  ( -0.9414334852479518956, -0.3371987438498165734, 0.000000000000000000 ) ) ;
#37716=CARTESIAN_POINT ( 'NONE',  ( -12.68721568607400485, 24.67147432707382038, -10.00000000000000000 ) ) ;
#37717=VERTEX_POINT ( 'NONE', #31926 ) ;
#37726=ORIENTED_EDGE ( 'NONE', *, *, #73488, .T. ) ;
#37729=FACE_OUTER_BOUND ( 'NONE', #12095, .T. ) ;
#37739=CIRCLE ( 'NONE', #11886, 70.00000000000001421 ) ;
#37743=CARTESIAN_POINT ( 'NONE',  ( 45.16679497745494132, 120.1723871950187714, 10.00000000000000000 ) ) ;
#37745=VECTOR ( 'NONE', #57226, 1000.000000000000000 ) ;
#37758=AXIS2_PLACEMENT_3D ( 'NONE', #51875, #64712, #87073 ) ;
#37759=FACE_OUTER_BOUND ( 'NONE', #90884, .T. ) ;
#37766=CARTESIAN_POINT ( 'NONE',  ( -14.83894680564148238, 24.48641780169620219, 10.00000000000000000 ) ) ;
#37769=DIRECTION ( 'NONE',  ( 0.2433040867433105825, 0.9699500612784163200, 0.000000000000000000 ) ) ;
#37774=EDGE_CURVE ( 'NONE', #18010, #12449, #27175, .T. ) ;
#37783=DIRECTION ( 'NONE',  ( 1.000000000000000000, 0.000000000000000000, 0.000000000000000000 ) ) ;
#37787=VERTEX_POINT ( 'NONE', #78559 ) ;
#37801=ORIENTED_EDGE ( 'NONE', *, *, #64611, .T. ) ;
#37804=ORIENTED_EDGE ( 'NONE', *, *, #26693, .T. ) ;
#37810=VECTOR ( 'NONE', #82599, 1000.000000000000114 ) ;
#37813=EDGE_CURVE ( 'NONE', #66505, #79746, #53038, .T. ) ;
#37814=CYLINDRICAL_SURFACE ( 'NONE', #87139, 14.99999999999967493 ) ;
#37818=CIRCLE ( 'NONE', #73428, 70.00000000000001421 ) ;
#37832=CONICAL_SURFACE ( 'NONE', #58867, 11.91750000000000043, 0.7853981633974482790 ) ;
#37835=ORIENTED_EDGE ( 'NONE', *, *, #97583, .F. ) ;
#37836=DIRECTION ( 'NONE',  ( -0.000000000000000000, -0.000000000000000000, -1.000000000000000000 ) ) ;
#37841=LINE ( 'NONE', #54031, #75489 ) ;
#37845=VERTEX_POINT ( 'NONE', #25337 ) ;
#37848=CARTESIAN_POINT ( 'NONE',  ( -19.65312891409030271, 93.06504152958497400, 59.99999999999999289 ) ) ;
#37849=ORIENTED_EDGE ( 'NONE', *, *, #96152, .F. ) ;
#37852=DIRECTION ( 'NONE',  ( -0.8435938723211519052, -0.5369817302126803638, 0.000000000000000000 ) ) ;
#37865=DIRECTION ( 'NONE',  ( -1.000000000000000000, 0.000000000000000000, 0.000000000000000000 ) ) ;
#37872=FACE_OUTER_BOUND ( 'NONE', #12178, .T. ) ;
#37875=CARTESIAN_POINT ( 'NONE',  ( -19.65312891409030271, 93.06504152958497400, 177.5919119679930134 ) ) ;
#37888=VECTOR ( 'NONE', #710, 1000.000000000000114 ) ;
#37897=LINE ( 'NONE', #12268, #50486 ) ;
#37901=LINE ( 'NONE', #14129, #50568 ) ;
#37911=CARTESIAN_POINT ( 'NONE',  ( 46.54103524584390783, 115.8319611975524595, 10.00000000000000000 ) ) ;
#37914=EDGE_LOOP ( 'NONE', ( #80643, #82750, #71399, #1204 ) ) ;
#37923=EDGE_CURVE ( 'NONE', #18075, #54901, #67649, .T. ) ;
#37925=ORIENTED_EDGE ( 'NONE', *, *, #32798, .F. ) ;
#37935=FACE_OUTER_BOUND ( 'NONE', #83125, .T. ) ;
#37938=ADVANCED_FACE ( 'NONE', ( #43527 ), #73454, .F. ) ;
#37946=ORIENTED_EDGE ( 'NONE', *, *, #57621, .T. ) ;
#37948=ORIENTED_EDGE ( 'NONE', *, *, #34302, .T. ) ;
#37949=ORIENTED_EDGE ( 'NONE', *, *, #60812, .F. ) ;
#37950=EDGE_CURVE ( 'NONE', #97599, #21181, #89209, .T. ) ;
#37951=FACE_BOUND ( 'NONE', #55299, .T. ) ;
#37958=PLANE ( 'NONE',  #81982 ) ;
#37960=EDGE_LOOP ( 'NONE', ( #35112, #5786, #59039, #35360 ) ) ;
#37961=VECTOR ( 'NONE', #6602, 1000.000000000000227 ) ;
#37963=DIRECTION ( 'NONE',  ( 0.2091919045418403900, 0.9778746070300412541, 0.000000000000000000 ) ) ;
#37964=ORIENTED_EDGE ( 'NONE', *, *, #13412, .T. ) ;
#37966=VECTOR ( 'NONE', #71520, 1000.000000000000227 ) ;
#37972=CARTESIAN_POINT ( 'NONE',  ( -23.47208873469913115, 24.42380372261332155, -10.00000000000000000 ) ) ;
#37973=CARTESIAN_POINT ( 'NONE',  ( 17.55280445478281237, 33.77154675864930056, 177.5919119679930134 ) ) ;
#37976=LINE ( 'NONE', #45098, #75686 ) ;
#37981=FACE_OUTER_BOUND ( 'NONE', #54008, .T. ) ;
#37985=VERTEX_POINT ( 'NONE', #64851 ) ;
#37988=CIRCLE ( 'NONE', #26746, 70.00000000000001421 ) ;
#37989=EDGE_CURVE ( 'NONE', #60097, #100252, #12148, .T. ) ;
#37991=LINE ( 'NONE', #24316, #79124 ) ;
#37997=CARTESIAN_POINT ( 'NONE',  ( 48.81784752633560487, 86.82484054835779830, -10.00000000000000000 ) ) ;
#38005=CARTESIAN_POINT ( 'NONE',  ( -19.65312891409030271, 93.06504152958497400, 10.00000000000000888 ) ) ;
#38015=VECTOR ( 'NONE', #8806, 1000.000000000000000 ) ;
#38018=FACE_OUTER_BOUND ( 'NONE', #231, .T. ) ;
#38022=LINE ( 'NONE', #31930, #79232 ) ;
#38028=DIRECTION ( 'NONE',  ( 0.000000000000000000, -0.000000000000000000, -1.000000000000000000 ) ) ;
#38036=LINE ( 'NONE', #20894, #35046 ) ;
#38056=VERTEX_POINT ( 'NONE', #13602 ) ;
#38059=ORIENTED_EDGE ( 'NONE', *, *, #45133, .T. ) ;
#38061=EDGE_CURVE ( 'NONE', #17145, #58533, #99203, .T. ) ;
#38063=EDGE_LOOP ( 'NONE', ( #22249, #20002, #94834, #72260 ) ) ;
#38064=LINE ( 'NONE', #68978, #5042 ) ;
#38066=ORIENTED_EDGE ( 'NONE', *, *, #92641, .T. ) ;
#38067=CARTESIAN_POINT ( 'NONE',  ( -5.322652039529478962, 75.81237378679655592, 14.51925131820462944 ) ) ;
#38069=DIRECTION ( 'NONE',  ( -1.000000000000000000, 0.000000000000000000, 0.000000000000000000 ) ) ;
#38075=CARTESIAN_POINT ( 'NONE',  ( 3.330649899756923382, 26.67094063374350554, 10.00000000000000000 ) ) ;
#38087=ORIENTED_EDGE ( 'NONE', *, *, #94717, .F. ) ;
#38088=AXIS2_PLACEMENT_3D ( 'NONE', #78843, #94064, #9426 ) ;
#38093=CIRCLE ( 'NONE', #88381, 70.00000000000001421 ) ;
#38109=CARTESIAN_POINT ( 'NONE',  ( 50.06890205215324130, 99.29708757740752390, 177.5919119679930134 ) ) ;
#38113=CARTESIAN_POINT ( 'NONE',  ( 30.34687108590969373, 93.06504152958497400, 60.00000000000000000 ) ) ;
#38116=PLANE ( 'NONE',  #4203 ) ;
#38120=ORIENTED_EDGE ( 'NONE', *, *, #51194, .T. ) ;
#38135=PLANE ( 'NONE',  #24605 ) ;
#38137=VECTOR ( 'NONE', #60284, 1000.000000000000114 ) ;
#38138=ADVANCED_FACE ( 'NONE', ( #93618 ), #87565, .F. ) ;
#38148=DIRECTION ( 'NONE',  ( 0.000000000000000000, 0.000000000000000000, 1.000000000000000000 ) ) ;
#38157=LINE ( 'NONE', #53377, #32765 ) ;
#38159=AXIS2_PLACEMENT_3D ( 'NONE', #12094, #43963, #34873 ) ;
#38160=CARTESIAN_POINT ( 'NONE',  ( 49.04287251715432205, 95.72274150194785136, -10.00000000000000000 ) ) ;
#38170=EDGE_LOOP ( 'NONE', ( #78769, #82303, #9697, #71269 ) ) ;
#38181=VERTEX_POINT ( 'NONE', #48992 ) ;
#38187=ORIENTED_EDGE ( 'NONE', *, *, #4394, .F. ) ;
#38202=VECTOR ( 'NONE', #87171, 1000.000000000000114 ) ;
#38205=CARTESIAN_POINT ( 'NONE',  ( -41.47773752187638507, 44.74077244691897448, 59.99999999999999289 ) ) ;
#38206=EDGE_LOOP ( 'NONE', ( #52265, #74891, #78582, #35079 ) ) ;
#38207=CIRCLE ( 'NONE', #83613, 49.99999999999999289 ) ;
#38211=VECTOR ( 'NONE', #42442, 1000.000000000000114 ) ;
#38213=ADVANCED_FACE ( 'NONE', ( #74314 ), #49986, .F. ) ;
#38219=LINE ( 'NONE', #46840, #62937 ) ;
#38220=EDGE_CURVE ( 'NONE', #55654, #83576, #88544, .T. ) ;
#38230=ORIENTED_EDGE ( 'NONE', *, *, #98832, .T. ) ;
#38231=VECTOR ( 'NONE', #37093, 1000.000000000000000 ) ;
#38236=AXIS2_PLACEMENT_3D ( 'NONE', #33298, #72833, #89551 ) ;
#38247=FACE_OUTER_BOUND ( 'NONE', #81888, .T. ) ;
#38249=CARTESIAN_POINT ( 'NONE',  ( -19.65312891409030271, 93.06504152958497400, 10.00000000000000888 ) ) ;
#38253=CARTESIAN_POINT ( 'NONE',  ( 49.54000814145098275, 103.6626726051169669, 177.5919119679930134 ) ) ;
#38266=EDGE_CURVE ( 'NONE', #8436, #41607, #26683, .T. ) ;
#38267=ADVANCED_FACE ( 'NONE', ( #73790 ), #98092, .T. ) ;
#38276=FACE_OUTER_BOUND ( 'NONE', #25124, .T. ) ;
#38281=VERTEX_POINT ( 'NONE', #3409 ) ;
#38287=VERTEX_POINT ( 'NONE', #73297 ) ;
#38289=AXIS2_PLACEMENT_3D ( 'NONE', #56912, #34137, #71147 ) ;
#38299=ORIENTED_EDGE ( 'NONE', *, *, #92568, .T. ) ;
#38317=VECTOR ( 'NONE', #42467, 1000.000000000000000 ) ;
#38318=VERTEX_POINT ( 'NONE', #66673 ) ;
#38335=EDGE_CURVE ( 'NONE', #69980, #4020, #96627, .T. ) ;
#38336=ORIENTED_EDGE ( 'NONE', *, *, #82629, .F. ) ;
#38341=FACE_OUTER_BOUND ( 'NONE', #29521, .T. ) ;
#38344=LINE ( 'NONE', #53549, #15601 ) ;
#38346=ORIENTED_EDGE ( 'NONE', *, *, #88883, .F. ) ;
#38349=VERTEX_POINT ( 'NONE', #28176 ) ;
#38353=AXIS2_PLACEMENT_3D ( 'NONE', #18230, #86677, #40992 ) ;
#38354=LINE ( 'NONE', #39838, #25737 ) ;
#38358=ORIENTED_EDGE ( 'NONE', *, *, #74016, .F. ) ;
#38359=AXIS2_PLACEMENT_3D ( 'NONE', #64730, #78951, #4802 ) ;
#38368=VECTOR ( 'NONE', #40835, 1000.000000000000000 ) ;
#38372=CARTESIAN_POINT ( 'NONE',  ( -45.75347490765857117, 28.11296735934751112, -10.00000000000000000 ) ) ;
#38374=PLANE ( 'NONE',  #85151 ) ;
#38377=DIRECTION ( 'NONE',  ( -0.000000000000000000, -0.000000000000000000, -1.000000000000000000 ) ) ;
#38378=CIRCLE ( 'NONE', #7656, 45.00000000000000000 ) ;
#38383=CARTESIAN_POINT ( 'NONE',  ( -19.65312891409030271, 93.06504152958497400, 40.00000000000000000 ) ) ;
#38387=LINE ( 'NONE', #56077, #23638 ) ;
#38390=VECTOR ( 'NONE', #58718, 1000.000000000000114 ) ;
#38391=EDGE_CURVE ( 'NONE', #93052, #69710, #90019, .T. ) ;
#38398=LINE ( 'NONE', #16113, #71993 ) ;
#38413=ORIENTED_EDGE ( 'NONE', *, *, #30771, .T. ) ;
#38416=VERTEX_POINT ( 'NONE', #96129 ) ;
#38424=LINE ( 'NONE', #14146, #15910 ) ;
#38427=AXIS2_PLACEMENT_3D ( 'NONE', #44632, #13278, #44140 ) ;
#38432=ORIENTED_EDGE ( 'NONE', *, *, #57118, .T. ) ;
#38433=FACE_OUTER_BOUND ( 'NONE', #17003, .T. ) ;
#38452=EDGE_CURVE ( 'NONE', #47670, #48810, #7848, .T. ) ;
#38453=EDGE_LOOP ( 'NONE', ( #83632, #97555, #78227, #73825 ) ) ;
#38460=DIRECTION ( 'NONE',  ( -0.8660254037844380415, -0.5000000000000011102, 0.000000000000000000 ) ) ;
#38462=CARTESIAN_POINT ( 'NONE',  ( -71.07364842061382149, 47.42355933771584375, -10.00000000000000000 ) ) ;
#38467=VERTEX_POINT ( 'NONE', #53453 ) ;
#38468=DIRECTION ( 'NONE',  ( -0.000000000000000000, -0.000000000000000000, -1.000000000000000000 ) ) ;
#38469=CARTESIAN_POINT ( 'NONE',  ( -44.74834796241764678, 29.05375577536863929, 10.00000000000000000 ) ) ;
#38472=DIRECTION ( 'NONE',  ( -0.7352104281592295454, 0.6778389383370672094, 0.000000000000000000 ) ) ;
#38476=DIRECTION ( 'NONE',  ( -1.000000000000000000, 0.000000000000000000, 0.000000000000000000 ) ) ;
#38478=ORIENTED_EDGE ( 'NONE', *, *, #97551, .T. ) ;
#38489=VECTOR ( 'NONE', #65956, 999.9999999999998863 ) ;
#38496=VECTOR ( 'NONE', #90893, 1000.000000000000114 ) ;
#38497=AXIS2_PLACEMENT_3D ( 'NONE', #84241, #89847, #54263 ) ;
#38502=DIRECTION ( 'NONE',  ( 1.000000000000000000, 0.000000000000000000, 0.000000000000000000 ) ) ;
#38504=LINE ( 'NONE', #85681, #79313 ) ;
#38506=CIRCLE ( 'NONE', #93595, 6.749999999999992006 ) ;
#38508=FACE_OUTER_BOUND ( 'NONE', #15432, .T. ) ;
#38510=EDGE_CURVE ( 'NONE', #30892, #38287, #14353, .T. ) ;
#38514=LINE ( 'NONE', #46104, #64003 ) ;
#38525=DIRECTION ( 'NONE',  ( 0.05364311403569549386, 0.9985601716053735810, 0.000000000000000000 ) ) ;
#38554=DIRECTION ( 'NONE',  ( -0.2877784213863818774, 0.9576970189910596343, 0.000000000000000000 ) ) ;
#38555=ORIENTED_EDGE ( 'NONE', *, *, #22731, .F. ) ;
#38556=ORIENTED_EDGE ( 'NONE', *, *, #94207, .F. ) ;
#38558=LINE ( 'NONE', #63373, #32989 ) ;
#38559=ORIENTED_EDGE ( 'NONE', *, *, #57745, .F. ) ;
#38568=VECTOR ( 'NONE', #84785, 1000.000000000000114 ) ;
#38569=VECTOR ( 'NONE', #74998, 1000.000000000000000 ) ;
#38573=VECTOR ( 'NONE', #68099, 1000.000000000000000 ) ;
#38578=EDGE_CURVE ( 'NONE', #98895, #70875, #37263, .T. ) ;
#38579=ORIENTED_EDGE ( 'NONE', *, *, #29834, .T. ) ;
#38580=CARTESIAN_POINT ( 'NONE',  ( -17.24452398764597305, 75.38583958956024844, 13.39357157112610608 ) ) ;
#38583=DIRECTION ( 'NONE',  ( -0.9957145386939475484, -0.09248003802712848054, 0.000000000000000000 ) ) ;
#38602=VERTEX_POINT ( 'NONE', #91504 ) ;
#38604=CARTESIAN_POINT ( 'NONE',  ( -66.21217304253430314, 40.79406095866393400, 177.5919119679930134 ) ) ;
#38622=VERTEX_POINT ( 'NONE', #78779 ) ;
#38628=LINE ( 'NONE', #15317, #3013 ) ;
#38633=AXIS2_PLACEMENT_3D ( 'NONE', #14930, #8347, #45820 ) ;
#38634=CARTESIAN_POINT ( 'NONE',  ( -19.65312891409030271, 93.06504152958497400, -10.00000000000000888 ) ) ;
#38641=VECTOR ( 'NONE', #88047, 1000.000000000000000 ) ;
#38656=VERTEX_POINT ( 'NONE', #56950 ) ;
#38657=AXIS2_PLACEMENT_3D ( 'NONE', #1203, #47777, #62995 ) ;
#38666=DIRECTION ( 'NONE',  ( -0.09274582908234026146, -0.9956898167541081701, 0.000000000000000000 ) ) ;
#38670=CARTESIAN_POINT ( 'NONE',  ( -19.65312891409030271, 93.06504152958497400, -10.00000000000000888 ) ) ;
#38680=EDGE_LOOP ( 'NONE', ( #73249, #45755, #14195, #47063 ) ) ;
#38681=VERTEX_POINT ( 'NONE', #81799 ) ;
#38684=VERTEX_POINT ( 'NONE', #20473 ) ;
#38689=ORIENTED_EDGE ( 'NONE', *, *, #85914, .T. ) ;
#38705=VERTEX_POINT ( 'NONE', #74183 ) ;
#38706=CARTESIAN_POINT ( 'NONE',  ( -63.08903959183645327, 39.77784189046417396, -10.00000000000000000 ) ) ;
#38717=CIRCLE ( 'NONE', #53328, 70.00000000000001421 ) ;
#38718=DIRECTION ( 'NONE',  ( 1.000000000000000000, 0.000000000000000000, 0.000000000000000000 ) ) ;
#38722=EDGE_CURVE ( 'NONE', #64867, #58503, #76175, .T. ) ;
#38725=EDGE_CURVE ( 'NONE', #12312, #55017, #99463, .T. ) ;
#38728=VECTOR ( 'NONE', #34944, 1000.000000000000000 ) ;
#38732=FACE_OUTER_BOUND ( 'NONE', #7948, .T. ) ;
#38743=ORIENTED_EDGE ( 'NONE', *, *, #36677, .F. ) ;
#38754=CARTESIAN_POINT ( 'NONE',  ( 24.48993338297023570, 63.68956773670547733, 59.99999999999999289 ) ) ;
#38757=EDGE_CURVE ( 'NONE', #16411, #51013, #98968, .T. ) ;
#38761=CARTESIAN_POINT ( 'NONE',  ( 48.58805178314242568, 84.67719436603331928, 10.00000000000000000 ) ) ;
#38792=VERTEX_POINT ( 'NONE', #7235 ) ;
#38793=DIRECTION ( 'NONE',  ( -0.000000000000000000, 0.000000000000000000, -1.000000000000000000 ) ) ;
#38796=DIRECTION ( 'NONE',  ( -0.000000000000000000, -0.000000000000000000, -1.000000000000000000 ) ) ;
#38797=VECTOR ( 'NONE', #5381, 1000.000000000000227 ) ;
#38801=ORIENTED_EDGE ( 'NONE', *, *, #35795, .F. ) ;
#38811=AXIS2_PLACEMENT_3D ( 'NONE', #98612, #61060, #22576 ) ;
#38816=CARTESIAN_POINT ( 'NONE',  ( -63.08903959183645327, 39.77784189046417396, 10.00000000000000000 ) ) ;
#38828=DIRECTION ( 'NONE',  ( -0.6363689690731114679, -0.7713848165480219343, 0.000000000000000000 ) ) ;
#38835=ORIENTED_EDGE ( 'NONE', *, *, #38972, .T. ) ;
#38837=CARTESIAN_POINT ( 'NONE',  ( -11.40312891409031693, 78.77562236714182120, 59.99999999999999289 ) ) ;
#38849=ORIENTED_EDGE ( 'NONE', *, *, #49315, .F. ) ;
#38852=ORIENTED_EDGE ( 'NONE', *, *, #16471, .T. ) ;
#38857=LINE ( 'NONE', #76392, #20325 ) ;
#38866=CARTESIAN_POINT ( 'NONE',  ( -19.65312891409030271, 93.06504152958497400, 10.00000000000000888 ) ) ;
#38871=VECTOR ( 'NONE', #99815, 1000.000000000000341 ) ;
#38887=LINE ( 'NONE', #69790, #88664 ) ;
#38892=CARTESIAN_POINT ( 'NONE',  ( -19.65312891409030271, 93.06504152958497400, 10.00000000000000888 ) ) ;
#38895=DIRECTION ( 'NONE',  ( -0.7005979833698863235, -0.7135562106085605594, 0.000000000000000000 ) ) ;
#38917=DIRECTION ( 'NONE',  ( 0.000000000000000000, -0.000000000000000000, 1.000000000000000000 ) ) ;
#38919=ORIENTED_EDGE ( 'NONE', *, *, #83623, .T. ) ;
#38925=EDGE_LOOP ( 'NONE', ( #41359, #74224, #78391, #39166 ) ) ;
#38926=LINE ( 'NONE', #70331, #26359 ) ;
#38929=VERTEX_POINT ( 'NONE', #73546 ) ;
#38939=CARTESIAN_POINT ( 'NONE',  ( -2.474071885612758148, 64.61506735976895754, -10.00000000000000000 ) ) ;
#38951=ORIENTED_EDGE ( 'NONE', *, *, #77903, .F. ) ;
#38953=DIRECTION ( 'NONE',  ( -0.7713848165480284846, 0.6363689690731033632, 0.000000000000000000 ) ) ;
#38954=ORIENTED_EDGE ( 'NONE', *, *, #73971, .F. ) ;
#38963=CYLINDRICAL_SURFACE ( 'NONE', #36580, 49.99999999999999289 ) ;
#38966=ADVANCED_FACE ( 'NONE', ( #10750 ), #48757, .F. ) ;
#38970=ORIENTED_EDGE ( 'NONE', *, *, #96554, .T. ) ;
#38972=EDGE_CURVE ( 'NONE', #10682, #1290, #72054, .T. ) ;
#38977=VERTEX_POINT ( 'NONE', #85554 ) ;
#38979=CARTESIAN_POINT ( 'NONE',  ( -14.81556294067986457, 35.32291336244301760, 59.99999999999999289 ) ) ;
#38985=EDGE_LOOP ( 'NONE', ( #43813, #43929, #59653, #31136 ) ) ;
#38988=DIRECTION ( 'NONE',  ( -0.9957145386939485476, -0.09248003802711830812, 0.000000000000000000 ) ) ;
#39027=DIRECTION ( 'NONE',  ( -0.09573633691163400961, -0.9954067278227237692, 0.000000000000000000 ) ) ;
#39034=CYLINDRICAL_SURFACE ( 'NONE', #54854, 70.00000000000002842 ) ;
#39035=VERTEX_POINT ( 'NONE', #6633 ) ;
#39040=ORIENTED_EDGE ( 'NONE', *, *, #5839, .T. ) ;
#39055=ORIENTED_EDGE ( 'NONE', *, *, #33619, .F. ) ;
#39068=ORIENTED_EDGE ( 'NONE', *, *, #49491, .F. ) ;
#39069=VECTOR ( 'NONE', #35700, 1000.000000000000114 ) ;
#39074=ORIENTED_EDGE ( 'NONE', *, *, #45604, .F. ) ;
#39087=ORIENTED_EDGE ( 'NONE', *, *, #41816, .F. ) ;
#39104=DIRECTION ( 'NONE',  ( -0.000000000000000000, -0.000000000000000000, 1.000000000000000000 ) ) ;
#39106=DIRECTION ( 'NONE',  ( 0.000000000000000000, -0.000000000000000000, 1.000000000000000000 ) ) ;
#39111=FACE_OUTER_BOUND ( 'NONE', #91120, .T. ) ;
#39113=CARTESIAN_POINT ( 'NONE',  ( 35.24274519906763459, 113.7842027444719406, 59.99999999999999289 ) ) ;
#39119=ORIENTED_EDGE ( 'NONE', *, *, #73954, .F. ) ;
#39125=CARTESIAN_POINT ( 'NONE',  ( 39.77289032284285497, 58.49985355908045648, -10.00000000000000000 ) ) ;
#39135=VERTEX_POINT ( 'NONE', #91740 ) ;
#39147=ORIENTED_EDGE ( 'NONE', *, *, #74300, .F. ) ;
#39163=ORIENTED_EDGE ( 'NONE', *, *, #2985, .T. ) ;
#39164=CARTESIAN_POINT ( 'NONE',  ( 42.45923888023187232, 122.5484010731363043, -10.00000000000000000 ) ) ;
#39166=ORIENTED_EDGE ( 'NONE', *, *, #75659, .F. ) ;
#39186=ORIENTED_EDGE ( 'NONE', *, *, #93127, .T. ) ;
#39192=EDGE_CURVE ( 'NONE', #70394, #77615, #36982, .T. ) ;
#39193=DIRECTION ( 'NONE',  ( -0.000000000000000000, -0.000000000000000000, -1.000000000000000000 ) ) ;
#39196=AXIS2_PLACEMENT_3D ( 'NONE', #64542, #33135, #2255 ) ;
#39203=EDGE_CURVE ( 'NONE', #83781, #26122, #93642, .T. ) ;
#39205=CARTESIAN_POINT ( 'NONE',  ( -64.94778771796556782, 41.33875607593970614, 10.00000000000000000 ) ) ;
#39208=PLANE ( 'NONE',  #39196 ) ;
#39211=DIRECTION ( 'NONE',  ( -0.000000000000000000, 0.000000000000000000, -1.000000000000000000 ) ) ;
#39212=CARTESIAN_POINT ( 'NONE',  ( -24.40473831032599605, 23.22649767201584581, 177.5919119679930134 ) ) ;
#39213=VERTEX_POINT ( 'NONE', #29414 ) ;
#39220=CARTESIAN_POINT ( 'NONE',  ( 33.92732256784238132, 47.61654385008751689, -10.00000000000000000 ) ) ;
#39229=ORIENTED_EDGE ( 'NONE', *, *, #59202, .T. ) ;
#39248=AXIS2_PLACEMENT_3D ( 'NONE', #76100, #6169, #53744 ) ;
#39250=CARTESIAN_POINT ( 'NONE',  ( 11.23059542939759936, 30.24628978557580794, -10.00000000000000000 ) ) ;
#39254=DIRECTION ( 'NONE',  ( -0.000000000000000000, -0.000000000000000000, 1.000000000000000000 ) ) ;
#39268=CARTESIAN_POINT ( 'NONE',  ( -70.89022602266993545, 47.22876919346843749, 10.00000000000000000 ) ) ;
#39273=ORIENTED_EDGE ( 'NONE', *, *, #37387, .T. ) ;
#39291=ORIENTED_EDGE ( 'NONE', *, *, #73450, .F. ) ;
#39293=DIRECTION ( 'NONE',  ( 0.3887219701523905169, 0.9213551052231946370, 0.000000000000000000 ) ) ;
#39295=CARTESIAN_POINT ( 'NONE',  ( -19.65312891409030271, 93.06504152958497400, 10.00000000000000888 ) ) ;
#39304=ORIENTED_EDGE ( 'NONE', *, *, #48621, .T. ) ;
#39316=EDGE_CURVE ( 'NONE', #73949, #82380, #35320, .T. ) ;
#39318=ADVANCED_FACE ( 'NONE', ( #47318 ), #3257, .F. ) ;
#39323=ORIENTED_EDGE ( 'NONE', *, *, #44251, .T. ) ;
#39343=LINE ( 'NONE', #93603, #13870 ) ;
#39348=ORIENTED_EDGE ( 'NONE', *, *, #53826, .T. ) ;
#39364=CARTESIAN_POINT ( 'NONE',  ( 50.32263495959776378, 94.90690751109829648, 10.00000000000000000 ) ) ;
#39376=CARTESIAN_POINT ( 'NONE',  ( -58.01722807680246774, 56.46252223527211811, 59.99999999999999289 ) ) ;
#39380=FACE_OUTER_BOUND ( 'NONE', #15880, .T. ) ;
#39387=FACE_OUTER_BOUND ( 'NONE', #41719, .T. ) ;
#39396=DIRECTION ( 'NONE',  ( -0.9979398670145497308, -0.06415622980648827411, 0.000000000000000000 ) ) ;
#39398=EDGE_CURVE ( 'NONE', #91230, #6477, #67010, .T. ) ;
#39399=EDGE_CURVE ( 'NONE', #43843, #75021, #74146, .T. ) ;
#39400=STYLED_ITEM('',(#100310),#42857);
#39403=CARTESIAN_POINT ( 'NONE',  ( -17.26249501324477720, 59.91680024587567033, -10.00000000000000000 ) ) ;
#39405=VERTEX_POINT ( 'NONE', #51829 ) ;
#39408=ORIENTED_EDGE ( 'NONE', *, *, #1153, .T. ) ;
#39415=CARTESIAN_POINT ( 'NONE',  ( 49.32130651720206771, 81.12656353050643077, 177.5919119679930134 ) ) ;
#39420=CARTESIAN_POINT ( 'NONE',  ( 49.87168060777529632, 103.2007005253944385, -10.00000000000000000 ) ) ;
#39422=ORIENTED_EDGE ( 'NONE', *, *, #84676, .F. ) ;
#39423=LINE ( 'NONE', #6560, #49824 ) ;
#39426=CARTESIAN_POINT ( 'NONE',  ( -19.65312891409030271, 93.06504152958497400, 10.00000000000000888 ) ) ;
#39427=EDGE_CURVE ( 'NONE', #68209, #10682, #73152, .T. ) ;
#39430=CARTESIAN_POINT ( 'NONE',  ( -38.94059804707394079, 66.00003524665416421, -10.00000000000000000 ) ) ;
#39438=ORIENTED_EDGE ( 'NONE', *, *, #7007, .T. ) ;
#39440=PLANE ( 'NONE',  #49646 ) ;
#39443=VERTEX_POINT ( 'NONE', #13336 ) ;
#39444=ORIENTED_EDGE ( 'NONE', *, *, #92424, .T. ) ;
#39449=CARTESIAN_POINT ( 'NONE',  ( 46.32860941106299890, 116.4404604047837779, 10.00000000000000000 ) ) ;
#39455=ORIENTED_EDGE ( 'NONE', *, *, #45322, .T. ) ;
#39458=EDGE_CURVE ( 'NONE', #17175, #49794, #19463, .T. ) ;
#39460=DIRECTION ( 'NONE',  ( -0.000000000000000000, -0.000000000000000000, -1.000000000000000000 ) ) ;
#39465=LINE ( 'NONE', #70390, #2838 ) ;
#39468=EDGE_CURVE ( 'NONE', #36836, #36314, #60391, .T. ) ;
#39469=DIRECTION ( 'NONE',  ( 1.000000000000000000, 0.000000000000000000, 0.000000000000000000 ) ) ;
#39476=EDGE_CURVE ( 'NONE', #8628, #28346, #53785, .T. ) ;
#39478=ORIENTED_EDGE ( 'NONE', *, *, #38220, .T. ) ;
#39479=VECTOR ( 'NONE', #52898, 1000.000000000000000 ) ;
#39482=LINE ( 'NONE', #31401, #32442 ) ;
#39487=CARTESIAN_POINT ( 'NONE',  ( -19.65312891409030271, 93.06504152958497400, 177.5919119679930134 ) ) ;
#39497=DIRECTION ( 'NONE',  ( -0.000000000000000000, -0.000000000000000000, -1.000000000000000000 ) ) ;
#39498=DIRECTION ( 'NONE',  ( 0.000000000000000000, 0.000000000000000000, 1.000000000000000000 ) ) ;
#39507=EDGE_CURVE ( 'NONE', #3834, #66626, #62863, .T. ) ;
#39512=DIRECTION ( 'NONE',  ( 1.000000000000000000, 0.000000000000000000, 0.000000000000000000 ) ) ;
#39515=CARTESIAN_POINT ( 'NONE',  ( 50.27371054362190961, 89.86549102125590593, 10.00000000000000000 ) ) ;
#39516=EDGE_CURVE ( 'NONE', #3474, #82113, #92350, .T. ) ;
#39520=DIRECTION ( 'NONE',  ( -1.000000000000000000, 0.000000000000000000, 0.000000000000000000 ) ) ;
#39523=DIRECTION ( 'NONE',  ( -1.000000000000000000, 0.000000000000000000, 0.000000000000000000 ) ) ;
#39539=AXIS2_PLACEMENT_3D ( 'NONE', #73518, #60271, #59270 ) ;
#39540=VERTEX_POINT ( 'NONE', #69502 ) ;
#39544=ORIENTED_EDGE ( 'NONE', *, *, #53947, .F. ) ;
#39549=AXIS2_PLACEMENT_3D ( 'NONE', #48322, #17932, #41706 ) ;
#39557=DIRECTION ( 'NONE',  ( 0.6600842437418872333, -0.7511915808658273797, 0.000000000000000000 ) ) ;
#39560=ORIENTED_EDGE ( 'NONE', *, *, #75925, .F. ) ;
#39565=VERTEX_POINT ( 'NONE', #76141 ) ;
#39578=VECTOR ( 'NONE', #84333, 1000.000000000000114 ) ;
#39580=CARTESIAN_POINT ( 'NONE',  ( 0.005075371086064872639, 27.18819441265828019, -10.00000000000000000 ) ) ;
#39585=ORIENTED_EDGE ( 'NONE', *, *, #28118, .F. ) ;
#39603=DIRECTION ( 'NONE',  ( 0.000000000000000000, -0.000000000000000000, 1.000000000000000000 ) ) ;
#39607=DIRECTION ( 'NONE',  ( -0.4999999999999999445, 0.8660254037844385966, 0.000000000000000000 ) ) ;
#39608=LINE ( 'NONE', #9238, #22130 ) ;
#39618=VECTOR ( 'NONE', #4934, 1000.000000000000000 ) ;
#39623=LINE ( 'NONE', #39125, #59754 ) ;
#39626=CARTESIAN_POINT ( 'NONE',  ( 44.10470679282202866, 121.9603419428074602, 10.00000000000000000 ) ) ;
#39633=ORIENTED_EDGE ( 'NONE', *, *, #62082, .T. ) ;
#39636=CARTESIAN_POINT ( 'NONE',  ( 25.98835327777827686, 41.64452202306098627, 10.00000000000000000 ) ) ;
#39643=CARTESIAN_POINT ( 'NONE',  ( -42.72532191160158987, 28.29708160126036987, 10.00000000000000000 ) ) ;
#39652=AXIS2_PLACEMENT_3D ( 'NONE', #18580, #80414, #48971 ) ;
#39659=ORIENTED_EDGE ( 'NONE', *, *, #65240, .T. ) ;
#39664=FACE_OUTER_BOUND ( 'NONE', #91679, .T. ) ;
#39666=VERTEX_POINT ( 'NONE', #83246 ) ;
#39667=PLANE ( 'NONE',  #63664 ) ;
#39671=EDGE_LOOP ( 'NONE', ( #12340, #84380, #66277, #26868 ) ) ;
#39673=LINE ( 'NONE', #92934, #10078 ) ;
#39676=VERTEX_POINT ( 'NONE', #75624 ) ;
#39677=VERTEX_POINT ( 'NONE', #13812 ) ;
#39691=EDGE_CURVE ( 'NONE', #97801, #49707, #53303, .T. ) ;
#39701=EDGE_CURVE ( 'NONE', #75907, #46284, #68505, .T. ) ;
#39704=ORIENTED_EDGE ( 'NONE', *, *, #46818, .T. ) ;
#39705=CARTESIAN_POINT ( 'NONE',  ( -58.00277386063315532, 34.50477571329874138, 10.00000000000000000 ) ) ;
#39707=DIRECTION ( 'NONE',  ( 0.000000000000000000, 0.000000000000000000, 1.000000000000000000 ) ) ;
#39708=DIRECTION ( 'NONE',  ( -0.6056412518070772855, -0.7957378174433814566, 0.000000000000000000 ) ) ;
#39748=AXIS2_PLACEMENT_3D ( 'NONE', #23425, #40120, #24933 ) ;
#39763=LINE ( 'NONE', #78313, #78206 ) ;
#39773=CARTESIAN_POINT ( 'NONE',  ( 9.830230629461709668, 30.95267373526312227, 10.00000000000000000 ) ) ;
#39779=ORIENTED_EDGE ( 'NONE', *, *, #95511, .F. ) ;
#39781=LINE ( 'NONE', #16511, #32144 ) ;
#39786=CARTESIAN_POINT ( 'NONE',  ( -62.95439910331221256, 68.06504152958493137, 60.00000000000000000 ) ) ;
#39788=VECTOR ( 'NONE', #32020, 1000.000000000000227 ) ;
#39795=AXIS2_PLACEMENT_3D ( 'NONE', #27653, #50926, #51430 ) ;
#39796=VERTEX_POINT ( 'NONE', #60149 ) ;
#39812=ORIENTED_EDGE ( 'NONE', *, *, #20917, .F. ) ;
#39821=DIRECTION ( 'NONE',  ( 0.000000000000000000, 0.000000000000000000, 1.000000000000000000 ) ) ;
#39826=VECTOR ( 'NONE', #86422, 1000.000000000000227 ) ;
#39827=LINE ( 'NONE', #69254, #25291 ) ;
#39838=CARTESIAN_POINT ( 'NONE',  ( -21.31413092498266693, 24.33771760303832465, -10.00000000000000000 ) ) ;
#39841=DIRECTION ( 'NONE',  ( 0.000000000000000000, 0.000000000000000000, 1.000000000000000000 ) ) ;
#39862=CIRCLE ( 'NONE', #96571, 70.00000000000001421 ) ;
#39871=AXIS2_PLACEMENT_3D ( 'NONE', #57650, #10576, #41451 ) ;
#39872=DIRECTION ( 'NONE',  ( 1.000000000000000000, 0.000000000000000000, 0.000000000000000000 ) ) ;
#39874=EDGE_CURVE ( 'NONE', #86151, #35869, #90486, .T. ) ;
#39892=CIRCLE ( 'NONE', #60940, 70.00000000000001421 ) ;
#39897=VECTOR ( 'NONE', #94221, 999.9999999999998863 ) ;
#39900=CARTESIAN_POINT ( 'NONE',  ( 33.47037235539275457, 49.41749479597460493, -10.00000000000000000 ) ) ;
#39902=ORIENTED_EDGE ( 'NONE', *, *, #12935, .T. ) ;
#39911=VERTEX_POINT ( 'NONE', #87547 ) ;
#39923=LINE ( 'NONE', #23734, #36773 ) ;
#39934=DIRECTION ( 'NONE',  ( -0.9819794923402673792, 0.1889875038809470387, 0.000000000000000000 ) ) ;
#39936=ORIENTED_EDGE ( 'NONE', *, *, #64941, .T. ) ;
#39940=DIRECTION ( 'NONE',  ( -0.000000000000000000, 0.000000000000000000, -1.000000000000000000 ) ) ;
#39944=VECTOR ( 'NONE', #94574, 1000.000000000000114 ) ;
#39947=CARTESIAN_POINT ( 'NONE',  ( -28.78056054657192320, 23.66266410781089391, -10.00000000000000000 ) ) ;
#39954=ORIENTED_EDGE ( 'NONE', *, *, #29657, .F. ) ;
#39955=CIRCLE ( 'NONE', #67439, 70.00000000000001421 ) ;
#39956=VERTEX_POINT ( 'NONE', #78889 ) ;
#39960=EDGE_CURVE ( 'NONE', #91080, #54771, #48974, .T. ) ;
#39961=CARTESIAN_POINT ( 'NONE',  ( 44.85937643310610667, 116.8208962945185050, 10.00000000000000000 ) ) ;
#39966=CIRCLE ( 'NONE', #48083, 0.1418229129680863287 ) ;
#39972=ADVANCED_FACE ( 'NONE', ( #9981 ), #3871, .F. ) ;
#39974=ADVANCED_FACE ( 'NONE', ( #96112 ), #56560, .F. ) ;
#39975=LINE ( 'NONE', #33399, #48589 ) ;
#39976=VERTEX_POINT ( 'NONE', #65655 ) ;
#39979=AXIS2_PLACEMENT_3D ( 'NONE', #57219, #59073, #71950 ) ;
#39993=CARTESIAN_POINT ( 'NONE',  ( -11.40312891409031693, 78.77562236714182120, 59.97499999999998721 ) ) ;
#39994=CARTESIAN_POINT ( 'NONE',  ( 8.106622824862185439, 30.17147933776455204, 10.00000000000000000 ) ) ;
#39996=EDGE_CURVE ( 'NONE', #9356, #96111, #64677, .T. ) ;
#39998=CARTESIAN_POINT ( 'NONE',  ( 41.85954357502990320, 126.4744881464662001, -10.00000000000000000 ) ) ;
#40005=AXIS2_PLACEMENT_3D ( 'NONE', #66898, #6606, #82662 ) ;
#40014=ADVANCED_FACE ( 'NONE', ( #87033 ), #1876, .F. ) ;
#40019=CARTESIAN_POINT ( 'NONE',  ( -19.65312891409030271, 93.06504152958497400, 10.00000000000000888 ) ) ;
#40023=CARTESIAN_POINT ( 'NONE',  ( -4.653128914090328472, 79.21777907560398546, 13.72050197239993707 ) ) ;
#40025=CARTESIAN_POINT ( 'NONE',  ( -19.65312891409030271, 93.06504152958497400, 59.99999999999999289 ) ) ;
#40026=ORIENTED_EDGE ( 'NONE', *, *, #61393, .T. ) ;
#40027=AXIS2_PLACEMENT_3D ( 'NONE', #48556, #87628, #41944 ) ;
#40041=ORIENTED_EDGE ( 'NONE', *, *, #68385, .T. ) ;
#40048=CIRCLE ( 'NONE', #7745, 70.00000000000001421 ) ;
#40053=CARTESIAN_POINT ( 'NONE',  ( -19.65312891409030271, 93.06504152958497400, 177.5919119679930134 ) ) ;
#40055=DIRECTION ( 'NONE',  ( 1.000000000000000000, 0.000000000000000000, 0.000000000000000000 ) ) ;
#40056=EDGE_CURVE ( 'NONE', #21527, #91318, #49461, .T. ) ;
#40061=EDGE_LOOP ( 'NONE', ( #15046, #56942, #10300, #73856 ) ) ;
#40063=VERTEX_POINT ( 'NONE', #25157 ) ;
#40089=VECTOR ( 'NONE', #72363, 1000.000000000000227 ) ;
#40097=ADVANCED_FACE ( 'NONE', ( #43348 ), #21085, .F. ) ;
#40112=DIRECTION ( 'NONE',  ( 1.000000000000000000, 0.000000000000000000, 0.000000000000000000 ) ) ;
#40118=CARTESIAN_POINT ( 'NONE',  ( 38.12092316966794669, 88.62496094012092840, 59.99999999999999289 ) ) ;
#40120=DIRECTION ( 'NONE',  ( 0.000000000000000000, 0.000000000000000000, 1.000000000000000000 ) ) ;
#40122=CIRCLE ( 'NONE', #51490, 70.00000000000001421 ) ;
#40125=DIRECTION ( 'NONE',  ( -0.3105719460338542404, -0.9505498757754611283, 0.000000000000000000 ) ) ;
#40126=ORIENTED_EDGE ( 'NONE', *, *, #90573, .F. ) ;
#40132=CARTESIAN_POINT ( 'NONE',  ( 30.68386671255119325, 44.42157463747831514, 177.5919119679930134 ) ) ;
#40133=CARTESIAN_POINT ( 'NONE',  ( 27.58098951138967436, 43.10352854649765675, 10.00000000000000000 ) ) ;
#40140=EDGE_LOOP ( 'NONE', ( #64659, #20984, #7063, #2318 ) ) ;
#40148=CARTESIAN_POINT ( 'NONE',  ( 45.88188149789386472, 72.29567966924398092, -10.00000000000000000 ) ) ;
#40153=VECTOR ( 'NONE', #50135, 1000.000000000000227 ) ;
#40155=ORIENTED_EDGE ( 'NONE', *, *, #11542, .F. ) ;
#40169=ORIENTED_EDGE ( 'NONE', *, *, #93761, .F. ) ;
#40170=CIRCLE ( 'NONE', #49965, 70.00000000000001421 ) ;
#40179=FACE_OUTER_BOUND ( 'NONE', #81970, .T. ) ;
#40181=ORIENTED_EDGE ( 'NONE', *, *, #45697, .T. ) ;
#40182=CARTESIAN_POINT ( 'NONE',  ( -19.65312891409030271, 93.06504152958497400, 10.00000000000000888 ) ) ;
#40183=DIRECTION ( 'NONE',  ( -0.000000000000000000, -0.000000000000000000, -1.000000000000000000 ) ) ;
#40185=CARTESIAN_POINT ( 'NONE',  ( -19.65312891409030271, 93.06504152958497400, 10.00000000000000888 ) ) ;
#40192=ORIENTED_EDGE ( 'NONE', *, *, #50199, .T. ) ;
#40194=ORIENTED_EDGE ( 'NONE', *, *, #32610, .F. ) ;
#40199=CARTESIAN_POINT ( 'NONE',  ( -72.48190909937208914, 49.06123820388767598, -10.00000000000000000 ) ) ;
#40201=DIRECTION ( 'NONE',  ( -0.7713848165480284846, 0.6363689690731033632, 0.000000000000000000 ) ) ;
#40208=FACE_OUTER_BOUND ( 'NONE', #17158, .T. ) ;
#40210=DIRECTION ( 'NONE',  ( 0.000000000000000000, 0.000000000000000000, 1.000000000000000000 ) ) ;
#40213=ADVANCED_FACE ( 'NONE', ( #37729 ), #61027, .F. ) ;
#40215=ORIENTED_EDGE ( 'NONE', *, *, #79460, .F. ) ;
#40219=ADVANCED_FACE ( 'NONE', ( #53433 ), #99559, .F. ) ;
#40220=VECTOR ( 'NONE', #37715, 1000.000000000000114 ) ;
#40225=DIRECTION ( 'NONE',  ( 0.2091919045418505763, 0.9778746070300391446, 0.000000000000000000 ) ) ;
#40234=VECTOR ( 'NONE', #42900, 1000.000000000000000 ) ;
#40236=DIRECTION ( 'NONE',  ( 0.000000000000000000, 0.000000000000000000, 1.000000000000000000 ) ) ;
#40240=LINE ( 'NONE', #71182, #39826 ) ;
#40241=VECTOR ( 'NONE', #9181, 1000.000000000000000 ) ;
#40242=LINE ( 'NONE', #100083, #91892 ) ;
#40251=AXIS2_PLACEMENT_3D ( 'NONE', #15828, #46733, #15316 ) ;
#40268=DIRECTION ( 'NONE',  ( -0.000000000000000000, -0.000000000000000000, -1.000000000000000000 ) ) ;
#40270=CARTESIAN_POINT ( 'NONE',  ( 6.117390533544191378, 29.33055864014942316, -10.00000000000000000 ) ) ;
#40273=EDGE_CURVE ( 'NONE', #76267, #16766, #31125, .T. ) ;
#40276=LINE ( 'NONE', #69691, #19993 ) ;
#40286=EDGE_LOOP ( 'NONE', ( #52439, #73382, #81370, #76506 ) ) ;
#40287=CARTESIAN_POINT ( 'NONE',  ( 32.24342178309110096, 47.97677246190463052, 10.00000000000000000 ) ) ;
#40288=VECTOR ( 'NONE', #94603, 1000.000000000000000 ) ;
#40293=EDGE_CURVE ( 'NONE', #26784, #64892, #43482, .T. ) ;
#40298=CARTESIAN_POINT ( 'NONE',  ( -59.65739779450132829, 37.15562860896454112, 10.00000000000000000 ) ) ;
#40302=AXIS2_PLACEMENT_3D ( 'NONE', #31260, #94111, #62651 ) ;
#40306=ORIENTED_EDGE ( 'NONE', *, *, #52129, .F. ) ;
#40307=ORIENTED_EDGE ( 'NONE', *, *, #68585, .T. ) ;
#40309=ORIENTED_EDGE ( 'NONE', *, *, #87890, .T. ) ;
#40312=DIRECTION ( 'NONE',  ( -1.000000000000000000, 0.000000000000000000, 0.000000000000000000 ) ) ;
#40315=ORIENTED_EDGE ( 'NONE', *, *, #89040, .T. ) ;
#40318=LINE ( 'NONE', #1851, #67432 ) ;
#40332=ADVANCED_FACE ( 'NONE', ( #38732 ), #14457, .F. ) ;
#40340=CARTESIAN_POINT ( 'NONE',  ( -48.47243291925848752, 30.64988553008148031, 10.00000000000000000 ) ) ;
#40345=EDGE_CURVE ( 'NONE', #79781, #66505, #77243, .T. ) ;
#40346=DIRECTION ( 'NONE',  ( -0.9762143704923770260, 0.2168075248790319320, 0.000000000000000000 ) ) ;
#40355=ORIENTED_EDGE ( 'NONE', *, *, #98341, .F. ) ;
#40362=CARTESIAN_POINT ( 'NONE',  ( -19.65312891409030271, 93.06504152958497400, -10.00000000000000888 ) ) ;
#40370=AXIS2_PLACEMENT_3D ( 'NONE', #29696, #7903, #100113 ) ;
#40372=AXIS2_PLACEMENT_3D ( 'NONE', #4033, #56219, #42031 ) ;
#40382=VECTOR ( 'NONE', #86684, 1000.000000000000227 ) ;
#40393=EDGE_CURVE ( 'NONE', #1103, #28901, #38219, .T. ) ;
#40397=ORIENTED_EDGE ( 'NONE', *, *, #81244, .F. ) ;
#40401=CARTESIAN_POINT ( 'NONE',  ( 11.76667899187106059, 31.90941714274742225, 10.00000000000000000 ) ) ;
#40403=CARTESIAN_POINT ( 'NONE',  ( 49.51900556837681222, 105.3795262313705763, 10.00000000000000000 ) ) ;
#40405=ADVANCED_FACE ( 'NONE', ( #68638 ), #15421, .F. ) ;
#40406=CIRCLE ( 'NONE', #14544, 70.00000000000001421 ) ;
#40426=ORIENTED_EDGE ( 'NONE', *, *, #99553, .F. ) ;
#40430=ORIENTED_EDGE ( 'NONE', *, *, #93462, .T. ) ;
#40432=EDGE_CURVE ( 'NONE', #37717, #70938, #92479, .T. ) ;
#40445=CIRCLE ( 'NONE', #53393, 0.1418229129684436818 ) ;
#40449=ORIENTED_EDGE ( 'NONE', *, *, #79059, .T. ) ;
#40454=ORIENTED_EDGE ( 'NONE', *, *, #57873, .T. ) ;
#40468=VERTEX_POINT ( 'NONE', #54934 ) ;
#40469=EDGE_CURVE ( 'NONE', #17797, #78693, #69134, .T. ) ;
#40470=EDGE_CURVE ( 'NONE', #74770, #73478, #25551, .T. ) ;
#40477=EDGE_CURVE ( 'NONE', #39976, #29044, #86907, .T. ) ;
#40496=LINE ( 'NONE', #24804, #81980 ) ;
#40502=DIRECTION ( 'NONE',  ( -0.000000000000000000, -0.000000000000000000, 1.000000000000000000 ) ) ;
#40522=CIRCLE ( 'NONE', #92362, 0.1418229129680863287 ) ;
#40526=CYLINDRICAL_SURFACE ( 'NONE', #73284, 70.00000000000002842 ) ;
#40530=CARTESIAN_POINT ( 'NONE',  ( -4.653128914090328472, 78.77562236714182120, 13.81405534229504717 ) ) ;
#40547=EDGE_CURVE ( 'NONE', #48375, #76464, #59676, .T. ) ;
#40559=PLANE ( 'NONE',  #44796 ) ;
#40565=EDGE_LOOP ( 'NONE', ( #88723, #12446, #66970, #88419 ) ) ;
#40567=ORIENTED_EDGE ( 'NONE', *, *, #88010, .T. ) ;
#40576=VERTEX_POINT ( 'NONE', #63040 ) ;
#40577=EDGE_CURVE ( 'NONE', #57230, #80767, #53184, .T. ) ;
#40581=ORIENTED_EDGE ( 'NONE', *, *, #13400, .T. ) ;
#40586=EDGE_CURVE ( 'NONE', #39956, #80413, #33660, .T. ) ;
#40598=CARTESIAN_POINT ( 'NONE',  ( -19.65312891409030271, 93.06504152958497400, -10.00000000000000888 ) ) ;
#40604=CIRCLE ( 'NONE', #32590, 0.1418229129681557177 ) ;
#40606=EDGE_LOOP ( 'NONE', ( #92715, #26510, #40426, #67481 ) ) ;
#40615=FACE_OUTER_BOUND ( 'NONE', #21620, .T. ) ;
#40618=CARTESIAN_POINT ( 'NONE',  ( -25.62627769214125451, 24.57763045674671076, -10.00000000000000000 ) ) ;
#40639=CARTESIAN_POINT ( 'NONE',  ( 46.80869107419874098, 110.6443039040113092, -10.00000000000000000 ) ) ;
#40656=ADVANCED_FACE ( 'NONE', ( #66043 ), #27054, .F. ) ;
#40677=VERTEX_POINT ( 'NONE', #41104 ) ;
#40681=CARTESIAN_POINT ( 'NONE',  ( 40.70814378237798081, 60.14496435084704018, -10.00000000000000000 ) ) ;
#40689=LINE ( 'NONE', #68724, #25530 ) ;
#40696=VERTEX_POINT ( 'NONE', #56817 ) ;
#40698=ORIENTED_EDGE ( 'NONE', *, *, #55203, .F. ) ;
#40717=ORIENTED_EDGE ( 'NONE', *, *, #72071, .T. ) ;
#40720=DIRECTION ( 'NONE',  ( -0.000000000000000000, -0.000000000000000000, 1.000000000000000000 ) ) ;
#40723=ORIENTED_EDGE ( 'NONE', *, *, #36321, .T. ) ;
#40732=EDGE_CURVE ( 'NONE', #94679, #23520, #24918, .T. ) ;
#40736=ORIENTED_EDGE ( 'NONE', *, *, #84876, .T. ) ;
#40747=ORIENTED_EDGE ( 'NONE', *, *, #8507, .F. ) ;
#40749=DIRECTION ( 'NONE',  ( -0.8660254037844380415, -0.5000000000000011102, 0.000000000000000000 ) ) ;
#40751=FACE_OUTER_BOUND ( 'NONE', #76015, .T. ) ;
#40755=CARTESIAN_POINT ( 'NONE',  ( -11.40312891409031693, 78.77562236714182120, 59.99999999999999289 ) ) ;
#40759=ORIENTED_EDGE ( 'NONE', *, *, #17732, .F. ) ;
#40761=DIRECTION ( 'NONE',  ( -0.5346708562974005208, -0.8450603975019800318, 0.000000000000000000 ) ) ;
#40764=FACE_OUTER_BOUND ( 'NONE', #23379, .T. ) ;
#40766=DIRECTION ( 'NONE',  ( -0.000000000000000000, -0.000000000000000000, -1.000000000000000000 ) ) ;
#40767=DIRECTION ( 'NONE',  ( -0.8035972437015875824, -0.5951734788405910193, 0.000000000000000000 ) ) ;
#40774=ORIENTED_EDGE ( 'NONE', *, *, #21881, .F. ) ;
#40775=CARTESIAN_POINT ( 'NONE',  ( 46.22371820283660782, 112.7232458147606451, -10.00000000000000000 ) ) ;
#40778=VERTEX_POINT ( 'NONE', #34522 ) ;
#40784=CARTESIAN_POINT ( 'NONE',  ( -64.74139798177010618, 41.16849083240310847, -10.00000000000000000 ) ) ;
#40794=EDGE_CURVE ( 'NONE', #43088, #62301, #61011, .T. ) ;
#40797=ORIENTED_EDGE ( 'NONE', *, *, #28353, .F. ) ;
#40800=LINE ( 'NONE', #86989, #30439 ) ;
#40806=ORIENTED_EDGE ( 'NONE', *, *, #89458, .F. ) ;
#40812=DIRECTION ( 'NONE',  ( 0.7490285521785712275, -0.6625377181876315191, 0.000000000000000000 ) ) ;
#40815=DIRECTION ( 'NONE',  ( -0.9404163354663446217, -0.3400251696390308442, 0.000000000000000000 ) ) ;
#40820=ORIENTED_EDGE ( 'NONE', *, *, #3660, .F. ) ;
#40822=PLANE ( 'NONE',  #31782 ) ;
#40832=LINE ( 'NONE', #62635, #93380 ) ;
#40835=DIRECTION ( 'NONE',  ( 0.000000000000000000, 0.000000000000000000, 1.000000000000000000 ) ) ;
#40836=ORIENTED_EDGE ( 'NONE', *, *, #77542, .T. ) ;
#40840=CARTESIAN_POINT ( 'NONE',  ( 47.05668214639808156, 76.45164061169337799, -10.00000000000000000 ) ) ;
#40848=AXIS2_PLACEMENT_3D ( 'NONE', #96923, #5175, #4167 ) ;
#40859=FACE_OUTER_BOUND ( 'NONE', #45181, .T. ) ;
#40870=DIRECTION ( 'NONE',  ( -0.7715546603183444097, -0.6361630342459738685, 0.000000000000000000 ) ) ;
#40895=CARTESIAN_POINT ( 'NONE',  ( -73.66720466879951346, 50.53642055324488780, -10.00000000000000000 ) ) ;
#40896=LINE ( 'NONE', #71845, #89802 ) ;
#40899=FACE_OUTER_BOUND ( 'NONE', #65803, .T. ) ;
#40910=ADVANCED_FACE ( 'NONE', ( #69122 ), #14918, .F. ) ;
#40912=CYLINDRICAL_SURFACE ( 'NONE', #12648, 70.00000000000002842 ) ;
#40914=LINE ( 'NONE', #95187, #65190 ) ;
#40917=AXIS2_PLACEMENT_3D ( 'NONE', #34198, #48396, #79836 ) ;
#40918=ORIENTED_EDGE ( 'NONE', *, *, #18080, .F. ) ;
#40922=VECTOR ( 'NONE', #7131, 1000.000000000000114 ) ;
#40936=AXIS2_PLACEMENT_3D ( 'NONE', #35309, #27726, #88586 ) ;
#40947=PLANE ( 'NONE',  #72491 ) ;
#40956=VERTEX_POINT ( 'NONE', #44821 ) ;
#40958=EDGE_CURVE ( 'NONE', #72572, #23641, #53908, .T. ) ;
#40976=PLANE ( 'NONE',  #60783 ) ;
#40979=ORIENTED_EDGE ( 'NONE', *, *, #82938, .T. ) ;
#40985=LINE ( 'NONE', #34412, #30421 ) ;
#40992=DIRECTION ( 'NONE',  ( -1.000000000000000000, 0.000000000000000000, 0.000000000000000000 ) ) ;
#40994=AXIS2_PLACEMENT_3D ( 'NONE', #41400, #33838, #35305 ) ;
#41000=DIRECTION ( 'NONE',  ( -0.7135562106085678868, 0.7005979833698787740, 0.000000000000000000 ) ) ;
#41004=CARTESIAN_POINT ( 'NONE',  ( -52.80137019779957086, 90.67440762873908966, -10.00000000000000000 ) ) ;
#41007=LINE ( 'NONE', #2551, #72284 ) ;
#41023=CARTESIAN_POINT ( 'NONE',  ( -9.047287092407536591, 85.10493810089948852, 14.06874990193072428 ) ) ;
#41031=CARTESIAN_POINT ( 'NONE',  ( 19.18375657693640335, 36.32959363016015431, -10.00000000000000000 ) ) ;
#41038=EDGE_CURVE ( 'NONE', #26456, #90241, #5068, .T. ) ;
#41042=ORIENTED_EDGE ( 'NONE', *, *, #58416, .F. ) ;
#41047=VERTEX_POINT ( 'NONE', #35457 ) ;
#41051=VERTEX_POINT ( 'NONE', #35950 ) ;
#41053=CARTESIAN_POINT ( 'NONE',  ( 45.05588048050944394, 66.36777381976857271, 177.5919119679930134 ) ) ;
#41070=FACE_OUTER_BOUND ( 'NONE', #89483, .T. ) ;
#41094=DIRECTION ( 'NONE',  ( -1.000000000000000000, 0.000000000000000000, 0.000000000000000000 ) ) ;
#41100=ORIENTED_EDGE ( 'NONE', *, *, #74008, .F. ) ;
#41104=CARTESIAN_POINT ( 'NONE',  ( 40.82928596147627331, 60.38352576601455723, -10.00000000000000000 ) ) ;
#41116=ADVANCED_FACE ( 'NONE', ( #47750 ), #48272, .T. ) ;
#41117=DIRECTION ( 'NONE',  ( -0.000000000000000000, -0.000000000000000000, -1.000000000000000000 ) ) ;
#41133=EDGE_CURVE ( 'NONE', #46853, #80971, #79218, .T. ) ;
#41141=ADVANCED_FACE ( 'NONE', ( #79715 ), #25986, .F. ) ;
#41152=VECTOR ( 'NONE', #62488, 1000.000000000000227 ) ;
#41154=EDGE_CURVE ( 'NONE', #49332, #32899, #50621, .T. ) ;
#41155=CARTESIAN_POINT ( 'NONE',  ( -54.45295541630240166, 33.76759809053437067, 10.00000000000000000 ) ) ;
#41157=FACE_OUTER_BOUND ( 'NONE', #52430, .T. ) ;
#41162=ADVANCED_FACE ( 'NONE', ( #82082 ), #83570, .T. ) ;
#41181=CARTESIAN_POINT ( 'NONE',  ( 44.85937643310610667, 116.8208962945185050, 10.00000000000000000 ) ) ;
#41182=DIRECTION ( 'NONE',  ( 0.9538480676139723391, -0.3002896333693372277, 0.000000000000000000 ) ) ;
#41187=CARTESIAN_POINT ( 'NONE',  ( 50.59379163489128928, 94.40700863652010355, 10.00000000000000000 ) ) ;
#41188=CARTESIAN_POINT ( 'NONE',  ( -64.74139798177012040, 41.16849083240310847, -10.00000000000000000 ) ) ;
#41190=CARTESIAN_POINT ( 'NONE',  ( -19.52881935598935570, 92.99677094728539828, 59.99999999999999289 ) ) ;
#41193=ORIENTED_EDGE ( 'NONE', *, *, #97085, .T. ) ;
#41195=ORIENTED_EDGE ( 'NONE', *, *, #88231, .F. ) ;
#41197=VERTEX_POINT ( 'NONE', #13639 ) ;
#41198=DIRECTION ( 'NONE',  ( 0.000000000000000000, 0.000000000000000000, 1.000000000000000000 ) ) ;
#41206=CARTESIAN_POINT ( 'NONE',  ( 50.26447705663006360, 96.46038765672592774, 10.00000000000000000 ) ) ;
#41211=DIRECTION ( 'NONE',  ( 0.000000000000000000, 0.000000000000000000, 1.000000000000000000 ) ) ;
#41213=ORIENTED_EDGE ( 'NONE', *, *, #42407, .T. ) ;
#41216=CARTESIAN_POINT ( 'NONE',  ( 33.63407072503001416, 49.62913085183822659, -10.00000000000000000 ) ) ;
#41228=VECTOR ( 'NONE', #56089, 1000.000000000000114 ) ;
#41235=ORIENTED_EDGE ( 'NONE', *, *, #86667, .T. ) ;
#41239=EDGE_CURVE ( 'NONE', #55233, #96593, #4529, .T. ) ;
#41243=LINE ( 'NONE', #80306, #22343 ) ;
#41244=CARTESIAN_POINT ( 'NONE',  ( 45.79324619304848909, 117.8999360398438654, 10.00000000000000000 ) ) ;
#41265=LINE ( 'NONE', #18002, #14280 ) ;
#41272=EDGE_CURVE ( 'NONE', #38622, #1218, #5533, .T. ) ;
#41280=VERTEX_POINT ( 'NONE', #44512 ) ;
#41283=CARTESIAN_POINT ( 'NONE',  ( -59.65739779450132829, 37.15562860896454112, -10.00000000000000000 ) ) ;
#41284=ADVANCED_FACE ( 'NONE', ( #89687 ), #99242, .F. ) ;
#41287=LINE ( 'NONE', #80863, #84983 ) ;
#41291=ORIENTED_EDGE ( 'NONE', *, *, #83461, .T. ) ;
#41299=ORIENTED_EDGE ( 'NONE', *, *, #84079, .F. ) ;
#41307=EDGE_LOOP ( 'NONE', ( #98192, #34218, #88474, #48588 ) ) ;
#41312=CARTESIAN_POINT ( 'NONE',  ( 21.20245638554209222, 36.22472881207375650, 10.00000000000000000 ) ) ;
#41313=EDGE_CURVE ( 'NONE', #25484, #34369, #98248, .T. ) ;
#41323=EDGE_CURVE ( 'NONE', #58606, #11558, #98755, .T. ) ;
#41329=CARTESIAN_POINT ( 'NONE',  ( 32.30839531297598910, 123.0650415295850593, 203.6502102582797420 ) ) ;
#41332=ORIENTED_EDGE ( 'NONE', *, *, #5131, .T. ) ;
#41333=AXIS2_PLACEMENT_3D ( 'NONE', #10471, #80921, #72801 ) ;
#41335=ORIENTED_EDGE ( 'NONE', *, *, #24098, .T. ) ;
#41336=CARTESIAN_POINT ( 'NONE',  ( 39.77289032284286208, 58.49985355908044937, -10.00000000000000000 ) ) ;
#41339=DIRECTION ( 'NONE',  ( 0.000000000000000000, 0.000000000000000000, 1.000000000000000000 ) ) ;
#41345=DIRECTION ( 'NONE',  ( 0.9403255362191060840, -0.3402761906661271873, 0.000000000000000000 ) ) ;
#41351=DIRECTION ( 'NONE',  ( -0.000000000000000000, 0.000000000000000000, -1.000000000000000000 ) ) ;
#41359=ORIENTED_EDGE ( 'NONE', *, *, #63303, .F. ) ;
#41360=AXIS2_PLACEMENT_3D ( 'NONE', #28323, #82083, #42032 ) ;
#41364=LINE ( 'NONE', #79428, #38641 ) ;
#41367=EDGE_CURVE ( 'NONE', #52913, #33351, #6536, .T. ) ;
#41375=DIRECTION ( 'NONE',  ( -1.000000000000000000, 0.000000000000000000, 0.000000000000000000 ) ) ;
#41376=EDGE_CURVE ( 'NONE', #95472, #7334, #12132, .T. ) ;
#41388=DIRECTION ( 'NONE',  ( 0.000000000000000000, 0.000000000000000000, 1.000000000000000000 ) ) ;
#41395=LINE ( 'NONE', #72338, #88995 ) ;
#41400=CARTESIAN_POINT ( 'NONE',  ( -19.65312891409030271, 93.06504152958497400, 177.5919119679930134 ) ) ;
#41401=ORIENTED_EDGE ( 'NONE', *, *, #91868, .F. ) ;
#41408=AXIS2_PLACEMENT_3D ( 'NONE', #53685, #21807, #84642 ) ;
#41409=FACE_OUTER_BOUND ( 'NONE', #51466, .T. ) ;
#41415=ORIENTED_EDGE ( 'NONE', *, *, #89458, .T. ) ;
#41417=ORIENTED_EDGE ( 'NONE', *, *, #94138, .F. ) ;
#41419=DIRECTION ( 'NONE',  ( -0.9184028970038772277, -0.3956464567955659817, 0.000000000000000000 ) ) ;
#41436=VECTOR ( 'NONE', #44726, 1000.000000000000000 ) ;
#41437=ORIENTED_EDGE ( 'NONE', *, *, #55034, .F. ) ;
#41438=ORIENTED_EDGE ( 'NONE', *, *, #36924, .T. ) ;
#41444=PLANE ( 'NONE',  #56068 ) ;
#41445=CARTESIAN_POINT ( 'NONE',  ( -57.88150100324660485, 35.92665207732902388, -10.00000000000000000 ) ) ;
#41450=ORIENTED_EDGE ( 'NONE', *, *, #86480, .F. ) ;
#41451=DIRECTION ( 'NONE',  ( -1.000000000000000000, 0.000000000000000000, 0.000000000000000000 ) ) ;
#41463=EDGE_LOOP ( 'NONE', ( #10077, #485, #76809, #32158 ) ) ;
#41465=ORIENTED_EDGE ( 'NONE', *, *, #25964, .F. ) ;
#41478=EDGE_CURVE ( 'NONE', #85923, #88235, #99741, .T. ) ;
#41479=VECTOR ( 'NONE', #51557, 1000.000000000000000 ) ;
#41480=FACE_OUTER_BOUND ( 'NONE', #24004, .T. ) ;
#41481=CARTESIAN_POINT ( 'NONE',  ( -9.055497838557601042, 23.87190447404380222, 177.5919119679930134 ) ) ;
#41482=ORIENTED_EDGE ( 'NONE', *, *, #12249, .F. ) ;
#41483=EDGE_CURVE ( 'NONE', #57725, #7407, #53610, .T. ) ;
#41490=FACE_OUTER_BOUND ( 'NONE', #90970, .T. ) ;
#41492=EDGE_CURVE ( 'NONE', #78230, #16775, #19151, .T. ) ;
#41496=VECTOR ( 'NONE', #25795, 1000.000000000000000 ) ;
#41502=DIRECTION ( 'NONE',  ( -0.9932214622066116716, 0.1162373735601425623, 0.000000000000000000 ) ) ;
#41504=DIRECTION ( 'NONE',  ( -0.000000000000000000, -0.000000000000000000, -1.000000000000000000 ) ) ;
#41505=DIRECTION ( 'NONE',  ( 0.000000000000000000, 0.000000000000000000, 1.000000000000000000 ) ) ;
#41510=ORIENTED_EDGE ( 'NONE', *, *, #96425, .F. ) ;
#41533=CARTESIAN_POINT ( 'NONE',  ( -9.885233179245682678, 85.35632536023292971, 14.27670553151784283 ) ) ;
#41546=ORIENTED_EDGE ( 'NONE', *, *, #7083, .F. ) ;
#41549=LINE ( 'NONE', #3096, #44026 ) ;
#41555=ADVANCED_FACE ( 'NONE', ( #78957 ), #10037, .F. ) ;
#41556=ORIENTED_EDGE ( 'NONE', *, *, #42609, .F. ) ;
#41570=VERTEX_POINT ( 'NONE', #13044 ) ;
#41571=AXIS2_PLACEMENT_3D ( 'NONE', #90012, #65175, #11001 ) ;
#41572=VECTOR ( 'NONE', #77510, 1000.000000000000000 ) ;
#41574=ORIENTED_EDGE ( 'NONE', *, *, #90858, .F. ) ;
#41585=PLANE ( 'NONE',  #77149 ) ;
#41595=DIRECTION ( 'NONE',  ( -0.9995486091367050685, 0.03004293549036784680, 0.000000000000000000 ) ) ;
#41607=VERTEX_POINT ( 'NONE', #35313 ) ;
#41614=FACE_OUTER_BOUND ( 'NONE', #27969, .T. ) ;
#41626=DIRECTION ( 'NONE',  ( -0.000000000000000000, 0.000000000000000000, -1.000000000000000000 ) ) ;
#41630=ORIENTED_EDGE ( 'NONE', *, *, #80152, .F. ) ;
#41636=DIRECTION ( 'NONE',  ( 0.5011331959107180323, 0.8653701635463924013, 0.000000000000000000 ) ) ;
#41651=VECTOR ( 'NONE', #90420, 1000.000000000000000 ) ;
#41660=CARTESIAN_POINT ( 'NONE',  ( 32.07315653955450330, 47.77038272570916888, -10.00000000000000000 ) ) ;
#41661=CARTESIAN_POINT ( 'NONE',  ( -14.06329310883398875, 23.28858607597028296, 177.5919119679930134 ) ) ;
#41665=FACE_OUTER_BOUND ( 'NONE', #17405, .T. ) ;
#41675=DIRECTION ( 'NONE',  ( 0.000000000000000000, 0.000000000000000000, 1.000000000000000000 ) ) ;
#41680=VERTEX_POINT ( 'NONE', #69701 ) ;
#41681=AXIS2_PLACEMENT_3D ( 'NONE', #67694, #20115, #35796 ) ;
#41685=ADVANCED_FACE ( 'NONE', ( #93031 ), #76333, .F. ) ;
#41700=ORIENTED_EDGE ( 'NONE', *, *, #39874, .T. ) ;
#41705=ORIENTED_EDGE ( 'NONE', *, *, #50876, .T. ) ;
#41706=DIRECTION ( 'NONE',  ( -1.000000000000000000, 0.000000000000000000, 0.000000000000000000 ) ) ;
#41711=CARTESIAN_POINT ( 'NONE',  ( -30.18034446749236821, 25.12100238203590763, 10.00000000000000000 ) ) ;
#41718=CARTESIAN_POINT ( 'NONE',  ( -10.54235908185773773, 24.92402704602492491, -10.00000000000000000 ) ) ;
#41719=EDGE_LOOP ( 'NONE', ( #96568, #50171, #56000, #51930 ) ) ;
#41721=ORIENTED_EDGE ( 'NONE', *, *, #11273, .F. ) ;
#41729=ORIENTED_EDGE ( 'NONE', *, *, #10882, .T. ) ;
#41731=ADVANCED_FACE ( 'NONE', ( #92547 ), #72743, .F. ) ;
#41742=EDGE_CURVE ( 'NONE', #21753, #7803, #2324, .T. ) ;
#41743=DIRECTION ( 'NONE',  ( -1.000000000000000000, 0.000000000000000000, 0.000000000000000000 ) ) ;
#41756=VECTOR ( 'NONE', #15563, 1000.000000000000000 ) ;
#41760=AXIS2_PLACEMENT_3D ( 'NONE', #63925, #94864, #25423 ) ;
#41762=CIRCLE ( 'NONE', #30484, 14.99999999999967493 ) ;
#41767=CYLINDRICAL_SURFACE ( 'NONE', #83145, 11.89249999999999652 ) ;
#41771=VERTEX_POINT ( 'NONE', #96054 ) ;
#41774=FACE_BOUND ( 'NONE', #89727, .T. ) ;
#41781=DIRECTION ( 'NONE',  ( -0.8080546441192405505, 0.5891075386695773242, 0.000000000000000000 ) ) ;
#41789=ORIENTED_EDGE ( 'NONE', *, *, #53472, .F. ) ;
#41797=VECTOR ( 'NONE', #85810, 1000.000000000000000 ) ;
#41809=LINE ( 'NONE', #3350, #55614 ) ;
#41815=ORIENTED_EDGE ( 'NONE', *, *, #29384, .F. ) ;
#41816=EDGE_CURVE ( 'NONE', #24657, #39565, #41287, .T. ) ;
#41831=VECTOR ( 'NONE', #60547, 1000.000000000000114 ) ;
#41837=EDGE_LOOP ( 'NONE', ( #50215, #82364, #48683, #36729 ) ) ;
#41840=ORIENTED_EDGE ( 'NONE', *, *, #34302, .F. ) ;
#41841=AXIS2_PLACEMENT_3D ( 'NONE', #46797, #53873, #9299 ) ;
#41845=CARTESIAN_POINT ( 'NONE',  ( 23.64814127513158937, 118.0650415295850451, 60.00000000000000000 ) ) ;
#41847=CARTESIAN_POINT ( 'NONE',  ( 47.96820964746023463, 80.67316705762479501, -10.00000000000000000 ) ) ;
#41849=CARTESIAN_POINT ( 'NONE',  ( -19.56352399852919888, 92.95511110727130699, 59.99999999999999289 ) ) ;
#41852=CARTESIAN_POINT ( 'NONE',  ( -39.52511050156713424, 25.94496742513404541, -10.00000000000000000 ) ) ;
#41853=VECTOR ( 'NONE', #66216, 1000.000000000000227 ) ;
#41858=ORIENTED_EDGE ( 'NONE', *, *, #21602, .T. ) ;
#41859=CARTESIAN_POINT ( 'NONE',  ( -19.71595605685117647, 92.93789402164532021, 59.99999999999999289 ) ) ;
#41869=AXIS2_PLACEMENT_3D ( 'NONE', #53698, #7614, #38502 ) ;
#41870=DIRECTION ( 'NONE',  ( 1.000000000000000000, 0.000000000000000000, 0.000000000000000000 ) ) ;
#41880=CARTESIAN_POINT ( 'NONE',  ( -19.65312891409030271, 93.06504152958497400, -10.00000000000000888 ) ) ;
#41903=PLANE ( 'NONE',  #71698 ) ;
#41907=AXIS2_PLACEMENT_3D ( 'NONE', #92762, #18111, #63706 ) ;
#41912=ORIENTED_EDGE ( 'NONE', *, *, #74800, .F. ) ;
#41919=CARTESIAN_POINT ( 'NONE',  ( -14.83894680564148238, 24.48641780169620219, -10.00000000000000000 ) ) ;
#41922=VECTOR ( 'NONE', #52550, 1000.000000000000227 ) ;
#41926=ORIENTED_EDGE ( 'NONE', *, *, #46855, .F. ) ;
#41931=DIRECTION ( 'NONE',  ( -0.000000000000000000, -0.000000000000000000, 1.000000000000000000 ) ) ;
#41940=CIRCLE ( 'NONE', #19339, 70.00000000000001421 ) ;
#41941=ORIENTED_EDGE ( 'NONE', *, *, #92875, .F. ) ;
#41944=DIRECTION ( 'NONE',  ( -1.000000000000000000, 0.000000000000000000, 0.000000000000000000 ) ) ;
#41945=EDGE_CURVE ( 'NONE', #17025, #27367, #77184, .T. ) ;
#41946=DIRECTION ( 'NONE',  ( -1.000000000000000000, 0.000000000000000000, 0.000000000000000000 ) ) ;
#41947=EDGE_CURVE ( 'NONE', #39213, #38622, #70072, .T. ) ;
#41948=ORIENTED_EDGE ( 'NONE', *, *, #46771, .F. ) ;
#41961=VERTEX_POINT ( 'NONE', #76691 ) ;
#41963=LINE ( 'NONE', #3490, #36657 ) ;
#41966=VERTEX_POINT ( 'NONE', #6297 ) ;
#41972=VERTEX_POINT ( 'NONE', #6793 ) ;
#41973=EDGE_LOOP ( 'NONE', ( #6238, #40581, #29893, #60394 ) ) ;
#41977=CIRCLE ( 'NONE', #97062, 70.00000000000001421 ) ;
#41983=FACE_OUTER_BOUND ( 'NONE', #71541, .T. ) ;
#41984=CARTESIAN_POINT ( 'NONE',  ( -19.65312891409030271, 93.06504152958497400, 10.00000000000000888 ) ) ;
#41985=VECTOR ( 'NONE', #12492, 999.9999999999998863 ) ;
#41994=FACE_OUTER_BOUND ( 'NONE', #71346, .T. ) ;
#41995=AXIS2_PLACEMENT_3D ( 'NONE', #7151, #84700, #51395 ) ;
#42001=DIRECTION ( 'NONE',  ( -0.5803476755362181327, -0.8143688203140567738, 0.000000000000000000 ) ) ;
#42010=DIRECTION ( 'NONE',  ( 0.000000000000000000, 0.000000000000000000, 1.000000000000000000 ) ) ;
#42012=DIRECTION ( 'NONE',  ( -0.9439450758449140499, 0.3301025504114431519, 0.000000000000000000 ) ) ;
#42016=CARTESIAN_POINT ( 'NONE',  ( -19.65312891409030271, 93.06504152958497400, -10.00000000000000888 ) ) ;
#42031=DIRECTION ( 'NONE',  ( -0.9481851146622203297, -0.3177184104407421716, 0.000000000000000000 ) ) ;
#42032=DIRECTION ( 'NONE',  ( -0.9923183454821322691, -0.1237105541964931832, 0.000000000000000000 ) ) ;
#42034=CARTESIAN_POINT ( 'NONE',  ( 29.59124024723001156, 43.31574901297117464, 177.5919119679930134 ) ) ;
#42035=DIRECTION ( 'NONE',  ( 0.000000000000000000, 0.000000000000000000, 1.000000000000000000 ) ) ;
#42037=ORIENTED_EDGE ( 'NONE', *, *, #57213, .T. ) ;
#42038=CARTESIAN_POINT ( 'NONE',  ( -6.063985638175826587, 82.91156382185207008, 13.42466032036877266 ) ) ;
#42041=LINE ( 'NONE', #50145, #92001 ) ;
#42050=ORIENTED_EDGE ( 'NONE', *, *, #25564, .F. ) ;
#42058=DIRECTION ( 'NONE',  ( 0.6066398774942437511, -0.7949767663484065272, 0.000000000000000000 ) ) ;
#42061=AXIS2_PLACEMENT_3D ( 'NONE', #59046, #95641, #50469 ) ;
#42062=ORIENTED_EDGE ( 'NONE', *, *, #94145, .T. ) ;
#42064=CYLINDRICAL_SURFACE ( 'NONE', #49209, 70.00000000000002842 ) ;
#42074=ADVANCED_FACE ( 'NONE', ( #31569 ), #84826, .T. ) ;
#42114=DIRECTION ( 'NONE',  ( 0.000000000000000000, 0.000000000000000000, 1.000000000000000000 ) ) ;
#42117=VECTOR ( 'NONE', #26695, 1000.000000000000000 ) ;
#42173=VERTEX_POINT ( 'NONE', #79735 ) ;
#42183=ORIENTED_EDGE ( 'NONE', *, *, #25840, .T. ) ;
#42186=ORIENTED_EDGE ( 'NONE', *, *, #24850, .F. ) ;
#42196=ORIENTED_EDGE ( 'NONE', *, *, #70287, .F. ) ;
#42202=VECTOR ( 'NONE', #63492, 1000.000000000000114 ) ;
#42218=ORIENTED_EDGE ( 'NONE', *, *, #15571, .F. ) ;
#42221=CARTESIAN_POINT ( 'NONE',  ( -62.95439910331221256, 68.06504152958493137, 60.00000000000000000 ) ) ;
#42222=CARTESIAN_POINT ( 'NONE',  ( -71.07364842061382149, 47.42355933771584375, -10.00000000000000000 ) ) ;
#42225=EDGE_LOOP ( 'NONE', ( #30578, #74856, #76094, #44183 ) ) ;
#42236=EDGE_CURVE ( 'NONE', #45437, #1972, #10296, .T. ) ;
#42250=ORIENTED_EDGE ( 'NONE', *, *, #87525, .F. ) ;
#42251=EDGE_CURVE ( 'NONE', #70967, #49038, #97895, .T. ) ;
#42255=CARTESIAN_POINT ( 'NONE',  ( -19.65312891409030271, 93.06504152958497400, 177.5919119679930134 ) ) ;
#42260=DIRECTION ( 'NONE',  ( -0.000000000000000000, 0.000000000000000000, 1.000000000000000000 ) ) ;
#42296=ORIENTED_EDGE ( 'NONE', *, *, #37813, .F. ) ;
#42302=EDGE_CURVE ( 'NONE', #1644, #15777, #57377, .T. ) ;
#42304=DIRECTION ( 'NONE',  ( -0.5634352399127592337, -0.8261602328994366307, 0.000000000000000000 ) ) ;
#42311=VERTEX_POINT ( 'NONE', #14767 ) ;
#42312=ADVANCED_FACE ( 'NONE', ( #61357 ), #44651, .T. ) ;
#42315=ORIENTED_EDGE ( 'NONE', *, *, #16462, .F. ) ;
#42316=LINE ( 'NONE', #27647, #91932 ) ;
#42318=DIRECTION ( 'NONE',  ( 0.1577859398657057433, -0.9874733399847793747, 0.000000000000000000 ) ) ;
#42327=FACE_OUTER_BOUND ( 'NONE', #16259, .T. ) ;
#42331=DIRECTION ( 'NONE',  ( -0.000000000000000000, -0.000000000000000000, -1.000000000000000000 ) ) ;
#42333=ORIENTED_EDGE ( 'NONE', *, *, #84274, .F. ) ;
#42335=EDGE_LOOP ( 'NONE', ( #39273, #3810, #81242, #39954 ) ) ;
#42336=LINE ( 'NONE', #10971, #30342 ) ;
#42342=CARTESIAN_POINT ( 'NONE',  ( -19.65312891409030271, 93.06504152958497400, 10.00000000000000888 ) ) ;
#42345=DIRECTION ( 'NONE',  ( -1.000000000000000000, 0.000000000000000000, 0.000000000000000000 ) ) ;
#42350=DIRECTION ( 'NONE',  ( -0.9413434404457865501, 0.3374500364938337049, 0.000000000000000000 ) ) ;
#42351=CARTESIAN_POINT ( 'NONE',  ( -31.59160691316810343, 24.09060609829247213, 177.5919119679930134 ) ) ;
#42357=ORIENTED_EDGE ( 'NONE', *, *, #96381, .F. ) ;
#42370=EDGE_CURVE ( 'NONE', #6973, #17025, #55776, .T. ) ;
#42371=DIRECTION ( 'NONE',  ( -0.1344185706417024839, 0.9909246428798921258, 0.000000000000000000 ) ) ;
#42372=VECTOR ( 'NONE', #18774, 1000.000000000000114 ) ;
#42373=CARTESIAN_POINT ( 'NONE',  ( 49.04287251715432205, 95.72274150194785136, 10.00000000000000000 ) ) ;
#42378=CARTESIAN_POINT ( 'NONE',  ( -48.02262176224491697, 41.70345557631966926, 59.99999999999999289 ) ) ;
#42382=EDGE_CURVE ( 'NONE', #88881, #71264, #13772, .T. ) ;
#42385=CARTESIAN_POINT ( 'NONE',  ( -19.65312891409030271, 93.06504152958497400, 177.5919119679930134 ) ) ;
#42396=VERTEX_POINT ( 'NONE', #37068 ) ;
#42400=DIRECTION ( 'NONE',  ( 0.02225111142181396273, 0.9997524133706774396, 0.000000000000000000 ) ) ;
#42401=CARTESIAN_POINT ( 'NONE',  ( 35.14194503788360890, 114.0493334331461455, 59.99999999999999289 ) ) ;
#42404=LINE ( 'NONE', #65710, #19410 ) ;
#42407=EDGE_CURVE ( 'NONE', #8402, #20413, #68615, .T. ) ;
#42409=ORIENTED_EDGE ( 'NONE', *, *, #95225, .T. ) ;
#42411=ORIENTED_EDGE ( 'NONE', *, *, #47834, .T. ) ;
#42422=CARTESIAN_POINT ( 'NONE',  ( -19.65312891409030271, 93.06504152958497400, -10.00000000000000888 ) ) ;
#42441=ORIENTED_EDGE ( 'NONE', *, *, #10851, .F. ) ;
#42442=DIRECTION ( 'NONE',  ( 0.1887253692075823441, -0.9820299053580097137, 0.000000000000000000 ) ) ;
#42443=CARTESIAN_POINT ( 'NONE',  ( -19.65312891409030271, 93.06504152958497400, 10.00000000000000888 ) ) ;
#42446=AXIS2_PLACEMENT_3D ( 'NONE', #81222, #66470, #27492 ) ;
#42447=ORIENTED_EDGE ( 'NONE', *, *, #52233, .T. ) ;
#42451=DIRECTION ( 'NONE',  ( -0.000000000000000000, -0.000000000000000000, -1.000000000000000000 ) ) ;
#42460=VECTOR ( 'NONE', #81163, 1000.000000000000227 ) ;
#42462=CARTESIAN_POINT ( 'NONE',  ( 41.71240375114938814, 62.05720181600818108, -10.00000000000000000 ) ) ;
#42467=DIRECTION ( 'NONE',  ( -0.8660254037844369313, -0.5000000000000029976, 0.000000000000000000 ) ) ;
#42468=VERTEX_POINT ( 'NONE', #74372 ) ;
#42473=LINE ( 'NONE', #59669, #18863 ) ;
#42476=DIRECTION ( 'NONE',  ( -0.06442261589617466477, -0.9979227057047523886, 0.000000000000000000 ) ) ;
#42489=ADVANCED_FACE ( 'NONE', ( #62098 ), #31212, .F. ) ;
#42497=DIRECTION ( 'NONE',  ( 1.000000000000000000, 0.000000000000000000, 0.000000000000000000 ) ) ;
#42500=FACE_OUTER_BOUND ( 'NONE', #73869, .T. ) ;
#42504=VECTOR ( 'NONE', #23197, 1000.000000000000000 ) ;
#42513=CIRCLE ( 'NONE', #18251, 70.00000000000001421 ) ;
#42518=CARTESIAN_POINT ( 'NONE',  ( -6.281727404287059890, 25.63055774385195917, -10.00000000000000000 ) ) ;
#42520=DIRECTION ( 'NONE',  ( 0.2168075248790211351, 0.9762143704923794685, 0.000000000000000000 ) ) ;
#42528=VECTOR ( 'NONE', #33320, 1000.000000000000000 ) ;
#42540=FACE_OUTER_BOUND ( 'NONE', #73965, .T. ) ;
#42541=EDGE_CURVE ( 'NONE', #10181, #27077, #37988, .T. ) ;
#42546=ORIENTED_EDGE ( 'NONE', *, *, #25860, .F. ) ;
#42548=DIRECTION ( 'NONE',  ( -0.6623377501714527993, 0.7492053821868994712, 0.000000000000000000 ) ) ;
#42561=ORIENTED_EDGE ( 'NONE', *, *, #68211, .F. ) ;
#42563=FACE_BOUND ( 'NONE', #37684, .T. ) ;
#42566=ORIENTED_EDGE ( 'NONE', *, *, #96113, .T. ) ;
#42572=EDGE_CURVE ( 'NONE', #52414, #85874, #63119, .T. ) ;
#42578=EDGE_CURVE ( 'NONE', #7863, #79260, #83398, .T. ) ;
#42585=CARTESIAN_POINT ( 'NONE',  ( 47.49582885874516336, 78.29235751436857527, -10.00000000000000000 ) ) ;
#42589=ORIENTED_EDGE ( 'NONE', *, *, #69077, .T. ) ;
#42591=LINE ( 'NONE', #12223, #2852 ) ;
#42596=DIRECTION ( 'NONE',  ( 0.1857746241280557598, -0.9825923819316327856, 0.000000000000000000 ) ) ;
#42599=CIRCLE ( 'NONE', #55604, 70.00000000000001421 ) ;
#42603=CARTESIAN_POINT ( 'NONE',  ( -48.71813016832984289, 30.75580926756359901, -10.00000000000000000 ) ) ;
#42606=CYLINDRICAL_SURFACE ( 'NONE', #48283, 70.00000000000002842 ) ;
#42609=EDGE_CURVE ( 'NONE', #52564, #82653, #73117, .T. ) ;
#42628=CARTESIAN_POINT ( 'NONE',  ( -67.83107014231842413, 42.28230845022618922, -10.00000000000000000 ) ) ;
#42656=ORIENTED_EDGE ( 'NONE', *, *, #10593, .F. ) ;
#42660=CARTESIAN_POINT ( 'NONE',  ( 38.90713690219553200, 54.71539658304152454, 10.00000000000000000 ) ) ;
#42666=ORIENTED_EDGE ( 'NONE', *, *, #34155, .T. ) ;
#42670=ORIENTED_EDGE ( 'NONE', *, *, #71711, .T. ) ;
#42671=CARTESIAN_POINT ( 'NONE',  ( -62.83817737799399339, 37.97373922903764765, 10.00000000000000000 ) ) ;
#42674=LINE ( 'NONE', #41181, #28080 ) ;
#42677=EDGE_CURVE ( 'NONE', #94567, #94878, #7095, .T. ) ;
#42682=LINE ( 'NONE', #57396, #55807 ) ;
#42696=CARTESIAN_POINT ( 'NONE',  ( -46.74660806181546491, 29.87360136034011049, -10.00000000000000000 ) ) ;
#42699=ORIENTED_EDGE ( 'NONE', *, *, #48738, .F. ) ;
#42700=DIRECTION ( 'NONE',  ( -0.9263643838751194348, -0.3766285016932073293, 0.000000000000000000 ) ) ;
#42704=DIRECTION ( 'NONE',  ( -1.000000000000000000, 0.000000000000000000, 0.000000000000000000 ) ) ;
#42705=VERTEX_POINT ( 'NONE', #28994 ) ;
#42713=ORIENTED_EDGE ( 'NONE', *, *, #6649, .T. ) ;
#42726=VERTEX_POINT ( 'NONE', #59868 ) ;
#42728=LINE ( 'NONE', #35146, #55922 ) ;
#42732=DIRECTION ( 'NONE',  ( -0.5696381972391160176, 0.8218955677251033043, 0.000000000000000000 ) ) ;
#42733=AXIS2_PLACEMENT_3D ( 'NONE', #74565, #80695, #35536 ) ;
#42758=LINE ( 'NONE', #20496, #69235 ) ;
#42765=CARTESIAN_POINT ( 'NONE',  ( -63.08903959183646748, 39.77784189046417396, -10.00000000000000000 ) ) ;
#42767=ORIENTED_EDGE ( 'NONE', *, *, #20259, .T. ) ;
#42773=VERTEX_POINT ( 'NONE', #75591 ) ;
#42785=ORIENTED_EDGE ( 'NONE', *, *, #11096, .F. ) ;
#42791=DIRECTION ( 'NONE',  ( -0.000000000000000000, -0.000000000000000000, -1.000000000000000000 ) ) ;
#42793=CARTESIAN_POINT ( 'NONE',  ( 42.45923888023187232, 122.5484010731363043, -10.00000000000000000 ) ) ;
#42797=CARTESIAN_POINT ( 'NONE',  ( -26.60548277334042666, 60.56602913741141947, -10.00000000000000000 ) ) ;
#42799=ORIENTED_EDGE ( 'NONE', *, *, #21058, .F. ) ;
#42804=ORIENTED_EDGE ( 'NONE', *, *, #41947, .F. ) ;
#42805=ADVANCED_FACE ( 'NONE', ( #76107 ), #6681, .T. ) ;
#42808=VERTEX_POINT ( 'NONE', #45654 ) ;
#42809=CARTESIAN_POINT ( 'NONE',  ( 30.68864658225822240, 104.9767549103658126, 59.99999999999999289 ) ) ;
#42815=DIRECTION ( 'NONE',  ( -0.9890802632347809320, 0.1473778574936430164, 0.000000000000000000 ) ) ;
#42816=VECTOR ( 'NONE', #53775, 1000.000000000000000 ) ;
#42817=LINE ( 'NONE', #11474, #92083 ) ;
#42843=VECTOR ( 'NONE', #92180, 1000.000000000000000 ) ;
#42845=EDGE_LOOP ( 'NONE', ( #59195, #13324, #32609, #23103 ) ) ;
#42849=EDGE_CURVE ( 'NONE', #27245, #27644, #38558, .T. ) ;
#42857=MANIFOLD_SOLID_BREP ( 'Split Line1', #96095 ) ;
#42860=LINE ( 'NONE', #72315, #91704 ) ;
#42861=ADVANCED_FACE ( 'NONE', ( #18288 ), #53752, .F. ) ;
#42862=CARTESIAN_POINT ( 'NONE',  ( 0.5143710859096835009, 78.77562236714182120, 59.99999999999999289 ) ) ;
#42865=EDGE_CURVE ( 'NONE', #76712, #80425, #58258, .T. ) ;
#42869=AXIS2_PLACEMENT_3D ( 'NONE', #86496, #9438, #71253 ) ;
#42884=CARTESIAN_POINT ( 'NONE',  ( -50.66443677795496825, 105.0157659939631145, -10.00000000000000000 ) ) ;
#42885=CARTESIAN_POINT ( 'NONE',  ( 0.005075371086064872639, 27.18819441265828019, 10.00000000000000000 ) ) ;
#42888=DIRECTION ( 'NONE',  ( -0.000000000000000000, 0.000000000000000000, -1.000000000000000000 ) ) ;
#42894=ORIENTED_EDGE ( 'NONE', *, *, #98274, .F. ) ;
#42899=ORIENTED_EDGE ( 'NONE', *, *, #13762, .T. ) ;
#42900=DIRECTION ( 'NONE',  ( -0.3358313672678264750, 0.9419221266957381600, 0.000000000000000000 ) ) ;
#42901=ORIENTED_EDGE ( 'NONE', *, *, #56716, .T. ) ;
#42902=DIRECTION ( 'NONE',  ( -0.8279987035736640077, -0.5607300124661883656, 0.000000000000000000 ) ) ;
#42907=AXIS2_PLACEMENT_3D ( 'NONE', #24899, #3622, #34500 ) ;
#42923=DIRECTION ( 'NONE',  ( 0.7059494278973771353, -0.7082622432767159415, 0.000000000000000000 ) ) ;
#42926=ADVANCED_FACE ( 'NONE', ( #89236 ), #42064, .T. ) ;
#42930=ORIENTED_EDGE ( 'NONE', *, *, #11100, .T. ) ;
#42937=EDGE_CURVE ( 'NONE', #23641, #32592, #72502, .T. ) ;
#42942=EDGE_CURVE ( 'NONE', #20188, #57629, #26877, .T. ) ;
#42955=DIRECTION ( 'NONE',  ( 0.000000000000000000, 0.000000000000000000, 1.000000000000000000 ) ) ;
#42972=EDGE_CURVE ( 'NONE', #28914, #34378, #19302, .T. ) ;
#42974=VECTOR ( 'NONE', #31518, 1000.000000000000000 ) ;
#42983=LINE ( 'NONE', #4506, #83281 ) ;
#43002=DIRECTION ( 'NONE',  ( 0.9979227057047517224, -0.06442261589618512863, 0.000000000000000000 ) ) ;
#43004=DIRECTION ( 'NONE',  ( 0.000000000000000000, 0.000000000000000000, 1.000000000000000000 ) ) ;
#43005=DIRECTION ( 'NONE',  ( -0.9598361373656995044, 0.2805612043866617111, 0.000000000000000000 ) ) ;
#43013=ORIENTED_EDGE ( 'NONE', *, *, #38335, .F. ) ;
#43029=CARTESIAN_POINT ( 'NONE',  ( 30.34687108590970794, 93.06504152958497400, 25.00000000000000000 ) ) ;
#43030=VERTEX_POINT ( 'NONE', #75990 ) ;
#43035=ORIENTED_EDGE ( 'NONE', *, *, #100167, .T. ) ;
#43037=CARTESIAN_POINT ( 'NONE',  ( -19.65312891409030271, 93.06504152958497400, 10.00000000000000888 ) ) ;
#43041=DIRECTION ( 'NONE',  ( -0.8600446134263898257, -0.5102188382608503492, 0.000000000000000000 ) ) ;
#43042=DIRECTION ( 'NONE',  ( -0.000000000000000000, -0.000000000000000000, -1.000000000000000000 ) ) ;
#43051=VERTEX_POINT ( 'NONE', #5073 ) ;
#43053=FACE_OUTER_BOUND ( 'NONE', #32757, .T. ) ;
#43062=VECTOR ( 'NONE', #84365, 1000.000000000000000 ) ;
#43064=EDGE_CURVE ( 'NONE', #97421, #24006, #78272, .T. ) ;
#43065=ORIENTED_EDGE ( 'NONE', *, *, #93329, .F. ) ;
#43068=ORIENTED_EDGE ( 'NONE', *, *, #73876, .T. ) ;
#43070=DIRECTION ( 'NONE',  ( -0.5609510170580174204, -0.8278489937552475642, 0.000000000000000000 ) ) ;
#43072=CARTESIAN_POINT ( 'NONE',  ( -19.60980644863471412, 92.92999745296690151, 59.99999999999999289 ) ) ;
#43077=ORIENTED_EDGE ( 'NONE', *, *, #88198, .F. ) ;
#43080=ORIENTED_EDGE ( 'NONE', *, *, #77016, .T. ) ;
#43081=AXIS2_PLACEMENT_3D ( 'NONE', #38754, #62038, #51983 ) ;
#43088=VERTEX_POINT ( 'NONE', #29858 ) ;
#43097=ADVANCED_FACE ( 'NONE', ( #13668 ), #91195, .T. ) ;
#43100=EDGE_CURVE ( 'NONE', #40576, #34323, #82116, .T. ) ;
#43109=ORIENTED_EDGE ( 'NONE', *, *, #94976, .T. ) ;
#43113=AXIS2_PLACEMENT_3D ( 'NONE', #6581, #76960, #76003 ) ;
#43120=VECTOR ( 'NONE', #72993, 1000.000000000000000 ) ;
#43121=CARTESIAN_POINT ( 'NONE',  ( -19.65312891409030271, 93.06504152958497400, 10.00000000000000000 ) ) ;
#43126=DIRECTION ( 'NONE',  ( 0.8660254037844399289, 0.4999999999999976130, -0.000000000000000000 ) ) ;
#43149=VERTEX_POINT ( 'NONE', #44040 ) ;
#43154=VERTEX_POINT ( 'NONE', #60728 ) ;
#43157=AXIS2_PLACEMENT_3D ( 'NONE', #70719, #22129, #45901 ) ;
#43160=VERTEX_POINT ( 'NONE', #52642 ) ;
#43162=LINE ( 'NONE', #45653, #94025 ) ;
#43163=DIRECTION ( 'NONE',  ( 0.000000000000000000, 0.000000000000000000, 1.000000000000000000 ) ) ;
#43172=EDGE_CURVE ( 'NONE', #52670, #38281, #81554, .T. ) ;
#43174=VERTEX_POINT ( 'NONE', #68350 ) ;
#43182=VERTEX_POINT ( 'NONE', #22253 ) ;
#43183=EDGE_CURVE ( 'NONE', #48909, #63370, #75097, .T. ) ;
#43187=EDGE_CURVE ( 'NONE', #68818, #46791, #37818, .T. ) ;
#43188=DIRECTION ( 'NONE',  ( -1.000000000000000000, 0.000000000000000000, 0.000000000000000000 ) ) ;
#43191=PLANE ( 'NONE',  #73577 ) ;
#43197=ORIENTED_EDGE ( 'NONE', *, *, #89907, .T. ) ;
#43199=VECTOR ( 'NONE', #30531, 1000.000000000000000 ) ;
#43210=CARTESIAN_POINT ( 'NONE',  ( -19.65312891409030271, 93.06504152958497400, 59.99999999999999289 ) ) ;
#43216=VECTOR ( 'NONE', #88765, 1000.000000000000000 ) ;
#43217=DIRECTION ( 'NONE',  ( 0.3358313672678264750, -0.9419221266957381600, 0.000000000000000000 ) ) ;
#43225=CARTESIAN_POINT ( 'NONE',  ( -1.979643831746636495, 43.07307769237275608, 59.99999999999999289 ) ) ;
#43227=CARTESIAN_POINT ( 'NONE',  ( 13.18854085237251539, 31.24736827225017777, -10.00000000000000000 ) ) ;
#43230=ORIENTED_EDGE ( 'NONE', *, *, #63312, .T. ) ;
#43231=AXIS2_PLACEMENT_3D ( 'NONE', #27425, #57799, #19348 ) ;
#43241=VECTOR ( 'NONE', #79224, 1000.000000000000114 ) ;
#43248=EDGE_CURVE ( 'NONE', #41972, #54771, #17149, .T. ) ;
#43251=DIRECTION ( 'NONE',  ( 0.2398044646550214765, 0.9708212084269268738, 0.000000000000000000 ) ) ;
#43258=DIRECTION ( 'NONE',  ( -0.000000000000000000, -0.000000000000000000, -1.000000000000000000 ) ) ;
#43266=CARTESIAN_POINT ( 'NONE',  ( -32.30932376655839988, 25.48519649537503184, -10.00000000000000000 ) ) ;
#43267=CARTESIAN_POINT ( 'NONE',  ( 48.29091023345865352, 82.53782597618220507, -10.00000000000000000 ) ) ;
#43271=ORIENTED_EDGE ( 'NONE', *, *, #72412, .T. ) ;
#43276=DIRECTION ( 'NONE',  ( -0.4245406647209920559, -0.9054088711727195093, 0.000000000000000000 ) ) ;
#43279=CARTESIAN_POINT ( 'NONE',  ( 22.66956910419568061, 38.88013629349136835, 10.00000000000000000 ) ) ;
#43287=FACE_OUTER_BOUND ( 'NONE', #94521, .T. ) ;
#43289=ORIENTED_EDGE ( 'NONE', *, *, #93204, .T. ) ;
#43291=CARTESIAN_POINT ( 'NONE',  ( -40.42249077443059235, 27.53003111760058630, 10.00000000000000000 ) ) ;
#43292=VERTEX_POINT ( 'NONE', #50055 ) ;
#43293=LINE ( 'NONE', #36689, #96775 ) ;
#43295=LINE ( 'NONE', #91438, #93747 ) ;
#43296=ORIENTED_EDGE ( 'NONE', *, *, #83749, .T. ) ;
#43302=ORIENTED_EDGE ( 'NONE', *, *, #35397, .T. ) ;
#43312=DIRECTION ( 'NONE',  ( -1.000000000000000000, 0.000000000000000000, 0.000000000000000000 ) ) ;
#43319=AXIS2_PLACEMENT_3D ( 'NONE', #82942, #29207, #28194 ) ;
#43322=ADVANCED_FACE ( 'NONE', ( #90602 ), #81494, .T. ) ;
#43332=EDGE_LOOP ( 'NONE', ( #16264, #24062, #39779, #50017 ) ) ;
#43336=DIRECTION ( 'NONE',  ( 0.000000000000000000, 0.000000000000000000, 1.000000000000000000 ) ) ;
#43337=LINE ( 'NONE', #41845, #98128 ) ;
#43347=CIRCLE ( 'NONE', #19157, 70.00000000000001421 ) ;
#43348=FACE_OUTER_BOUND ( 'NONE', #69410, .T. ) ;
#43350=DIRECTION ( 'NONE',  ( -0.9995486091367050685, 0.03004293549036790231, 0.000000000000000000 ) ) ;
#43352=VECTOR ( 'NONE', #46724, 1000.000000000000000 ) ;
#43353=CARTESIAN_POINT ( 'NONE',  ( -8.406493707509316238, 25.24382671950691304, -10.00000000000000000 ) ) ;
#43354=DIRECTION ( 'NONE',  ( 1.000000000000000000, 1.465097884282125932E-13, 0.000000000000000000 ) ) ;
#43358=ORIENTED_EDGE ( 'NONE', *, *, #41154, .T. ) ;
#43359=LINE ( 'NONE', #81915, #41985 ) ;
#43363=LINE ( 'NONE', #57067, #29139 ) ;
#43367=CARTESIAN_POINT ( 'NONE',  ( 24.55112987542764458, 40.41347472807389352, 10.00000000000000000 ) ) ;
#43383=VECTOR ( 'NONE', #642, 1000.000000000000000 ) ;
#43385=EDGE_CURVE ( 'NONE', #95480, #66118, #68732, .T. ) ;
#43400=DIRECTION ( 'NONE',  ( -0.9999990636452669168, -0.001368469433193631119, 0.000000000000000000 ) ) ;
#43403=ORIENTED_EDGE ( 'NONE', *, *, #38266, .F. ) ;
#43407=DIRECTION ( 'NONE',  ( 0.000000000000000000, 0.000000000000000000, 1.000000000000000000 ) ) ;
#43412=ORIENTED_EDGE ( 'NONE', *, *, #90040, .F. ) ;
#43416=ORIENTED_EDGE ( 'NONE', *, *, #77997, .F. ) ;
#43419=VERTEX_POINT ( 'NONE', #83989 ) ;
#43422=VECTOR ( 'NONE', #97852, 999.9999999999998863 ) ;
#43425=DIRECTION ( 'NONE',  ( -0.06142469166374898287, -0.9981117208278906805, 0.000000000000000000 ) ) ;
#43435=EDGE_LOOP ( 'NONE', ( #24296, #96420, #241, #67874 ) ) ;
#43436=EDGE_LOOP ( 'NONE', ( #45121, #45334, #30737, #57947 ) ) ;
#43438=VECTOR ( 'NONE', #96415, 1000.000000000000000 ) ;
#43445=ADVANCED_FACE ( 'NONE', ( #76362 ), #16034, .F. ) ;
#43452=DIRECTION ( 'NONE',  ( 1.000000000000000000, 0.000000000000000000, 0.000000000000000000 ) ) ;
#43454=EDGE_LOOP ( 'NONE', ( #75287, #28424, #35120, #75449 ) ) ;
#43471=ORIENTED_EDGE ( 'NONE', *, *, #49308, .T. ) ;
#43482=CIRCLE ( 'NONE', #25721, 50.00000000000000711 ) ;
#43489=CIRCLE ( 'NONE', #85644, 70.00000000000001421 ) ;
#43506=ADVANCED_FACE ( 'NONE', ( #53529 ), #92099, .F. ) ;
#43508=CARTESIAN_POINT ( 'NONE',  ( -69.61464189717713680, 45.83092310410447112, -10.00000000000000000 ) ) ;
#43519=CARTESIAN_POINT ( 'NONE',  ( 33.47037235539277589, 49.41749479597460493, -10.00000000000000000 ) ) ;
#43520=LINE ( 'NONE', #13636, #21711 ) ;
#43526=CARTESIAN_POINT ( 'NONE',  ( -19.65312891409030271, 93.06504152958497400, 10.00000000000000888 ) ) ;
#43527=FACE_OUTER_BOUND ( 'NONE', #3835, .T. ) ;
#43539=LINE ( 'NONE', #74480, #96718 ) ;
#43544=DIRECTION ( 'NONE',  ( 0.8560416229147678191, 0.5169068966820336009, 0.000000000000000000 ) ) ;
#43546=CARTESIAN_POINT ( 'NONE',  ( 48.61286661847091040, 84.94359857078811160, -10.00000000000000000 ) ) ;
#43548=EDGE_LOOP ( 'NONE', ( #33618, #775, #20643, #81038 ) ) ;
#43552=ORIENTED_EDGE ( 'NONE', *, *, #72458, .F. ) ;
#43556=DIRECTION ( 'NONE',  ( -0.000000000000000000, -0.000000000000000000, 1.000000000000000000 ) ) ;
#43558=ORIENTED_EDGE ( 'NONE', *, *, #59685, .T. ) ;
#43561=DIRECTION ( 'NONE',  ( -0.000000000000000000, -0.000000000000000000, 1.000000000000000000 ) ) ;
#43562=CARTESIAN_POINT ( 'NONE',  ( -6.134002256249970308, 43.13092002735066188, 59.99999999999999289 ) ) ;
#43563=EDGE_CURVE ( 'NONE', #79622, #16754, #75247, .T. ) ;
#43565=VECTOR ( 'NONE', #38666, 999.9999999999998863 ) ;
#43568=VERTEX_POINT ( 'NONE', #42809 ) ;
#43574=FACE_BOUND ( 'NONE', #66757, .T. ) ;
#43575=LINE ( 'NONE', #66383, #12640 ) ;
#43578=CARTESIAN_POINT ( 'NONE',  ( -75.18208942163934694, 50.44421862632483311, 10.00000000000000000 ) ) ;
#43579=CARTESIAN_POINT ( 'NONE',  ( -19.65312891409030271, 93.06504152958497400, 10.00000000000000888 ) ) ;
#43582=EDGE_LOOP ( 'NONE', ( #15895, #81580, #5330, #60376 ) ) ;
#43583=AXIS2_PLACEMENT_3D ( 'NONE', #99631, #93545, #76808 ) ;
#43586=LINE ( 'NONE', #34983, #75548 ) ;
#43593=LINE ( 'NONE', #51186, #57544 ) ;
#43597=DIRECTION ( 'NONE',  ( -0.9995486091367050685, 0.03004293549036784680, 0.000000000000000000 ) ) ;
#43603=CARTESIAN_POINT ( 'NONE',  ( -2.073866539663252073, 26.60322154129611505, -10.00000000000000000 ) ) ;
#43612=DIRECTION ( 'NONE',  ( -0.000000000000000000, -0.000000000000000000, -1.000000000000000000 ) ) ;
#43625=VECTOR ( 'NONE', #19455, 1000.000000000000114 ) ;
#43638=EDGE_CURVE ( 'NONE', #82969, #66038, #89440, .T. ) ;
#43640=ADVANCED_FACE ( 'NONE', ( #98502 ), #29092, .F. ) ;
#43641=VECTOR ( 'NONE', #94509, 1000.000000000000000 ) ;
#43664=DIRECTION ( 'NONE',  ( -0.000000000000000000, 0.000000000000000000, 1.000000000000000000 ) ) ;
#43668=DIRECTION ( 'NONE',  ( 0.000000000000000000, -0.000000000000000000, -1.000000000000000000 ) ) ;
#43684=EDGE_CURVE ( 'NONE', #97801, #98545, #57203, .T. ) ;
#43689=ORIENTED_EDGE ( 'NONE', *, *, #69842, .T. ) ;
#43692=VERTEX_POINT ( 'NONE', #79217 ) ;
#43693=CARTESIAN_POINT ( 'NONE',  ( 50.59379163489128928, 94.40700863652010355, -10.00000000000000000 ) ) ;
#43694=ORIENTED_EDGE ( 'NONE', *, *, #37703, .T. ) ;
#43702=VECTOR ( 'NONE', #14992, 1000.000000000000000 ) ;
#43703=LINE ( 'NONE', #87895, #27314 ) ;
#43705=ORIENTED_EDGE ( 'NONE', *, *, #2043, .T. ) ;
#43712=ORIENTED_EDGE ( 'NONE', *, *, #40470, .T. ) ;
#43719=CARTESIAN_POINT ( 'NONE',  ( -11.40312891409031693, 78.77562236714182120, 52.49999999999999289 ) ) ;
#43731=DIRECTION ( 'NONE',  ( -0.000000000000000000, -0.000000000000000000, -1.000000000000000000 ) ) ;
#43732=VERTEX_POINT ( 'NONE', #94405 ) ;
#43740=CARTESIAN_POINT ( 'NONE',  ( 49.06003799288187395, 95.45573527953635562, -10.00000000000000000 ) ) ;
#43755=EDGE_CURVE ( 'NONE', #41607, #17175, #15248, .T. ) ;
#43760=EDGE_CURVE ( 'NONE', #58606, #35725, #48782, .T. ) ;
#43790=CARTESIAN_POINT ( 'NONE',  ( 15.11407551230992219, 32.30945333909093620, -10.00000000000000000 ) ) ;
#43793=ORIENTED_EDGE ( 'NONE', *, *, #15702, .T. ) ;
#43813=ORIENTED_EDGE ( 'NONE', *, *, #45583, .F. ) ;
#43827=VERTEX_POINT ( 'NONE', #88835 ) ;
#43837=PLANE ( 'NONE',  #4244 ) ;
#43843=VERTEX_POINT ( 'NONE', #40148 ) ;
#43844=CARTESIAN_POINT ( 'NONE',  ( 27.53018959221258655, 41.35687530090520880, 177.5919119679930134 ) ) ;
#43849=CARTESIAN_POINT ( 'NONE',  ( -23.47208873469913115, 24.42380372261332155, -10.00000000000000000 ) ) ;
#43857=CARTESIAN_POINT ( 'NONE',  ( 30.80155721116056355, 46.36891074996812989, 10.00000000000000000 ) ) ;
#43862=AXIS2_PLACEMENT_3D ( 'NONE', #62973, #25993, #46774 ) ;
#43864=CARTESIAN_POINT ( 'NONE',  ( 46.22371820283660782, 112.7232458147606451, -10.00000000000000000 ) ) ;
#43875=PLANE ( 'NONE',  #53009 ) ;
#43881=DIRECTION ( 'NONE',  ( 0.000000000000000000, -0.000000000000000000, 1.000000000000000000 ) ) ;
#43882=EDGE_CURVE ( 'NONE', #89109, #15864, #8763, .T. ) ;
#43884=EDGE_CURVE ( 'NONE', #42705, #6582, #46868, .T. ) ;
#43899=CARTESIAN_POINT ( 'NONE',  ( 49.07419501245632176, 91.40403951869188859, -10.00000000000000000 ) ) ;
#43900=LINE ( 'NONE', #67206, #73305 ) ;
#43911=CARTESIAN_POINT ( 'NONE',  ( 17.60357497223980516, 35.28838536716091312, -10.00000000000000000 ) ) ;
#43912=VERTEX_POINT ( 'NONE', #14960 ) ;
#43915=ORIENTED_EDGE ( 'NONE', *, *, #98914, .T. ) ;
#43922=CARTESIAN_POINT ( 'NONE',  ( 17.26055046206296950, 33.28368158147418399, 10.00000000000000000 ) ) ;
#43928=VECTOR ( 'NONE', #7398, 1000.000000000000114 ) ;
#43929=ORIENTED_EDGE ( 'NONE', *, *, #61883, .T. ) ;
#43934=DIRECTION ( 'NONE',  ( 0.7694697644498922351, -0.6386832404231594928, 0.000000000000000000 ) ) ;
#43954=ORIENTED_EDGE ( 'NONE', *, *, #4583, .F. ) ;
#43963=DIRECTION ( 'NONE',  ( 0.3077152132536229434, 0.9514785060800257099, 0.000000000000000000 ) ) ;
#43964=ORIENTED_EDGE ( 'NONE', *, *, #6634, .F. ) ;
#43970=CARTESIAN_POINT ( 'NONE',  ( -22.20871200244593879, 23.11170711957622004, -10.00000000000000000 ) ) ;
#43971=DIRECTION ( 'NONE',  ( 0.5864613938488599798, -0.8099771808667527440, 0.000000000000000000 ) ) ;
#43981=LINE ( 'NONE', #27317, #74271 ) ;
#43994=DIRECTION ( 'NONE',  ( -0.000000000000000000, -0.000000000000000000, -1.000000000000000000 ) ) ;
#44012=VERTEX_POINT ( 'NONE', #59307 ) ;
#44013=DIRECTION ( 'NONE',  ( 1.000000000000000000, 0.000000000000000000, 0.000000000000000000 ) ) ;
#44014=DIRECTION ( 'NONE',  ( 1.000000000000000000, 0.000000000000000000, 0.000000000000000000 ) ) ;
#44020=FACE_OUTER_BOUND ( 'NONE', #71041, .T. ) ;
#44026=VECTOR ( 'NONE', #33986, 1000.000000000000000 ) ;
#44040=CARTESIAN_POINT ( 'NONE',  ( 28.66479899236089679, 61.08171380020798580, 59.99999999999999289 ) ) ;
#44047=CARTESIAN_POINT ( 'NONE',  ( -19.65312891409030271, 93.06504152958497400, 60.00000000000000000 ) ) ;
#44050=LINE ( 'NONE', #26390, #46412 ) ;
#44052=ADVANCED_FACE ( 'NONE', ( #20352 ), #4643, .F. ) ;
#44055=ORIENTED_EDGE ( 'NONE', *, *, #50427, .F. ) ;
#44061=DIRECTION ( 'NONE',  ( 0.4174706225611763410, 0.9086904199442095154, 0.000000000000000000 ) ) ;
#44065=EDGE_LOOP ( 'NONE', ( #13442, #71222, #50385, #53407 ) ) ;
#44067=CARTESIAN_POINT ( 'NONE',  ( 49.06003799288187395, 95.45573527953635562, -10.00000000000000000 ) ) ;
#44070=EDGE_LOOP ( 'NONE', ( #84735, #60377, #41705, #71884 ) ) ;
#44088=EDGE_LOOP ( 'NONE', ( #23720, #29133, #95805, #36304 ) ) ;
#44097=AXIS2_PLACEMENT_3D ( 'NONE', #25080, #95555, #1802 ) ;
#44098=VECTOR ( 'NONE', #87483, 1000.000000000000114 ) ;
#44099=CARTESIAN_POINT ( 'NONE',  ( -19.65312891409030271, 93.06504152958497400, 10.00000000000000888 ) ) ;
#44102=VECTOR ( 'NONE', #38917, 1000.000000000000000 ) ;
#44115=AXIS2_PLACEMENT_3D ( 'NONE', #20323, #96355, #33523 ) ;
#44123=CARTESIAN_POINT ( 'NONE',  ( 20.94669640352213236, 37.57748520232516398, -10.00000000000000000 ) ) ;
#44125=ADVANCED_FACE ( 'NONE', ( #96764 ), #3059, .T. ) ;
#44140=DIRECTION ( 'NONE',  ( 1.000000000000000000, 0.000000000000000000, 0.000000000000000000 ) ) ;
#44155=LINE ( 'NONE', #95935, #51266 ) ;
#44156=ORIENTED_EDGE ( 'NONE', *, *, #76416, .T. ) ;
#44174=EDGE_CURVE ( 'NONE', #56928, #72976, #83552, .T. ) ;
#44183=ORIENTED_EDGE ( 'NONE', *, *, #25022, .T. ) ;
#44186=ORIENTED_EDGE ( 'NONE', *, *, #100057, .T. ) ;
#44193=EDGE_CURVE ( 'NONE', #39676, #72634, #5517, .T. ) ;
#44196=VECTOR ( 'NONE', #26723, 1000.000000000000227 ) ;
#44197=EDGE_LOOP ( 'NONE', ( #36242, #304, #83377, #37326 ) ) ;
#44199=DIRECTION ( 'NONE',  ( 0.000000000000000000, 0.000000000000000000, 1.000000000000000000 ) ) ;
#44204=ORIENTED_EDGE ( 'NONE', *, *, #52570, .F. ) ;
#44212=DIRECTION ( 'NONE',  ( 0.000000000000000000, 0.000000000000000000, 1.000000000000000000 ) ) ;
#44215=DIRECTION ( 'NONE',  ( -0.1032265479692960342, 0.9946578707245736783, 0.000000000000000000 ) ) ;
#44220=CARTESIAN_POINT ( 'NONE',  ( 41.85954357502990320, 126.4744881464662001, 10.00000000000000000 ) ) ;
#44222=CARTESIAN_POINT ( 'NONE',  ( 37.40852414342580801, 106.7320921514703826, 59.99999999999999289 ) ) ;
#44226=VERTEX_POINT ( 'NONE', #15092 ) ;
#44227=LINE ( 'NONE', #51855, #83539 ) ;
#44230=CARTESIAN_POINT ( 'NONE',  ( 48.98810889288134263, 89.24608170897542436, -10.00000000000000000 ) ) ;
#44233=CARTESIAN_POINT ( 'NONE',  ( -63.39619785071779035, 38.08345695496143435, -10.00000000000000000 ) ) ;
#44251=EDGE_CURVE ( 'NONE', #14427, #11056, #18547, .T. ) ;
#44269=VECTOR ( 'NONE', #89358, 1000.000000000000000 ) ;
#44279=ORIENTED_EDGE ( 'NONE', *, *, #45944, .T. ) ;
#44283=DIRECTION ( 'NONE',  ( -0.4554470513245730823, -0.8902628732232696906, 0.000000000000000000 ) ) ;
#44290=CARTESIAN_POINT ( 'NONE',  ( 45.66470909604093720, 114.5311720768849995, 10.00000000000000000 ) ) ;
#44311=VERTEX_POINT ( 'NONE', #50490 ) ;
#44318=FACE_OUTER_BOUND ( 'NONE', #8190, .T. ) ;
#44319=ADVANCED_FACE ( 'NONE', ( #87589 ), #18114, .F. ) ;
#44322=VERTEX_POINT ( 'NONE', #72838 ) ;
#44323=DIRECTION ( 'NONE',  ( -0.9599109957006544125, -0.2803049773603353279, 0.000000000000000000 ) ) ;
#44341=ORIENTED_EDGE ( 'NONE', *, *, #12345, .T. ) ;
#44344=AXIS2_PLACEMENT_3D ( 'NONE', #45032, #27847, #81589 ) ;
#44357=PLANE ( 'NONE',  #7585 ) ;
#44368=DIRECTION ( 'NONE',  ( -0.9922852870422786964, 0.1239754375649568807, 0.000000000000000000 ) ) ;
#44380=CARTESIAN_POINT ( 'NONE',  ( -19.65312891409030271, 93.06504152958497400, 45.00000000000000711 ) ) ;
#44384=LINE ( 'NONE', #91528, #20708 ) ;
#44389=CARTESIAN_POINT ( 'NONE',  ( 38.65784837781280459, 56.65029301956751340, -10.00000000000000000 ) ) ;
#44395=DIRECTION ( 'NONE',  ( 0.1696015684586875405, 0.9855127132494806430, 0.000000000000000000 ) ) ;
#44398=ORIENTED_EDGE ( 'NONE', *, *, #78927, .T. ) ;
#44399=CARTESIAN_POINT ( 'NONE',  ( 37.67364948790085322, 52.89489741671174272, -10.00000000000000000 ) ) ;
#44401=VECTOR ( 'NONE', #85777, 1000.000000000000114 ) ;
#44411=ORIENTED_EDGE ( 'NONE', *, *, #31583, .F. ) ;
#44415=ORIENTED_EDGE ( 'NONE', *, *, #65194, .F. ) ;
#44425=FACE_OUTER_BOUND ( 'NONE', #73131, .T. ) ;
#44428=DIRECTION ( 'NONE',  ( 0.5102188382608533468, -0.8600446134263880493, 0.000000000000000000 ) ) ;
#44438=DIRECTION ( 'NONE',  ( 1.000000000000000000, 3.568574007723717001E-15, 0.000000000000000000 ) ) ;
#44445=ORIENTED_EDGE ( 'NONE', *, *, #32593, .T. ) ;
#44457=CARTESIAN_POINT ( 'NONE',  ( -19.65312891409030271, 93.06504152958497400, -10.00000000000000888 ) ) ;
#44459=CARTESIAN_POINT ( 'NONE',  ( 44.44844410339183582, 68.22168590943847732, 10.00000000000000000 ) ) ;
#44463=CARTESIAN_POINT ( 'NONE',  ( 29.30989995549245464, 44.80713248141895377, -10.00000000000000000 ) ) ;
#44464=DIRECTION ( 'NONE',  ( -0.7300871660154473197, -0.6833540297821711906, 0.000000000000000000 ) ) ;
#44465=ORIENTED_EDGE ( 'NONE', *, *, #71824, .F. ) ;
#44470=CARTESIAN_POINT ( 'NONE',  ( 44.44844410339183582, 68.22168590943847732, -10.00000000000000000 ) ) ;
#44471=CARTESIAN_POINT ( 'NONE',  ( 41.37327796571899796, 124.7191351846657028, -10.00000000000000000 ) ) ;
#44472=VECTOR ( 'NONE', #8101, 1000.000000000000000 ) ;
#44488=CARTESIAN_POINT ( 'NONE',  ( 27.82114452072190147, 69.44848197715137417, 59.99999999999999289 ) ) ;
#44490=LINE ( 'NONE', #60179, #7795 ) ;
#44494=ADVANCED_FACE ( 'NONE', ( #40764 ), #18502, .F. ) ;
#44500=EDGE_CURVE ( 'NONE', #90241, #30665, #33704, .T. ) ;
#44501=VECTOR ( 'NONE', #75585, 1000.000000000000000 ) ;
#44504=FACE_OUTER_BOUND ( 'NONE', #37095, .T. ) ;
#44511=LINE ( 'NONE', #24094, #8547 ) ;
#44512=CARTESIAN_POINT ( 'NONE',  ( -59.82327302696292293, 35.73826312759339174, -10.00000000000000000 ) ) ;
#44516=ORIENTED_EDGE ( 'NONE', *, *, #93241, .F. ) ;
#44523=DIRECTION ( 'NONE',  ( -0.6384778167143362326, 0.7696402260561061581, 0.000000000000000000 ) ) ;
#44525=DIRECTION ( 'NONE',  ( 0.000000000000000000, 0.000000000000000000, 1.000000000000000000 ) ) ;
#44527=CARTESIAN_POINT ( 'NONE',  ( -19.65312891409030271, 93.06504152958497400, 60.00000000000000000 ) ) ;
#44534=ORIENTED_EDGE ( 'NONE', *, *, #42382, .T. ) ;
#44536=FACE_OUTER_BOUND ( 'NONE', #18425, .T. ) ;
#44537=VECTOR ( 'NONE', #32977, 1000.000000000000227 ) ;
#44555=ORIENTED_EDGE ( 'NONE', *, *, #32346, .F. ) ;
#44558=CARTESIAN_POINT ( 'NONE',  ( -19.65312891409030271, 93.06504152958497400, 10.00000000000000888 ) ) ;
#44565=ORIENTED_EDGE ( 'NONE', *, *, #55315, .F. ) ;
#44566=EDGE_CURVE ( 'NONE', #70676, #22043, #55303, .T. ) ;
#44570=CARTESIAN_POINT ( 'NONE',  ( 0.1404396296823678947, 45.26966602009034801, 59.99999999999999289 ) ) ;
#44572=EDGE_CURVE ( 'NONE', #26627, #5926, #72040, .T. ) ;
#44575=CIRCLE ( 'NONE', #42907, 70.00000000000001421 ) ;
#44580=LINE ( 'NONE', #37972, #27107 ) ;
#44587=LINE ( 'NONE', #13235, #88343 ) ;
#44595=VECTOR ( 'NONE', #34647, 1000.000000000000000 ) ;
#44599=LINE ( 'NONE', #6119, #15964 ) ;
#44600=DIRECTION ( 'NONE',  ( 0.2701803667135113662, 0.9628097264997651505, 0.000000000000000000 ) ) ;
#44602=VECTOR ( 'NONE', #45066, 1000.000000000000114 ) ;
#44609=PLANE ( 'NONE',  #58071 ) ;
#44618=DIRECTION ( 'NONE',  ( 0.03277852384265245167, -0.9994626398093610087, 0.000000000000000000 ) ) ;
#44629=EDGE_CURVE ( 'NONE', #92184, #43912, #76738, .T. ) ;
#44632=CARTESIAN_POINT ( 'NONE',  ( -19.65312891409030271, 93.06504152958497400, -10.00000000000000888 ) ) ;
#44633=LINE ( 'NONE', #83697, #53107 ) ;
#44635=CARTESIAN_POINT ( 'NONE',  ( 39.64431452495995245, 58.26521502737223557, -10.00000000000000000 ) ) ;
#44636=DIRECTION ( 'NONE',  ( -0.9055221650797476984, -0.4242989612870696758, 0.000000000000000000 ) ) ;
#44641=AXIS2_PLACEMENT_3D ( 'NONE', #44457, #53555, #76859 ) ;
#44650=VECTOR ( 'NONE', #31716, 1000.000000000000114 ) ;
#44651=CYLINDRICAL_SURFACE ( 'NONE', #5687, 70.00000000000002842 ) ;
#44653=VERTEX_POINT ( 'NONE', #89287 ) ;
#44659=FACE_OUTER_BOUND ( 'NONE', #93676, .T. ) ;
#44661=DIRECTION ( 'NONE',  ( 1.000000000000000000, 0.000000000000000000, 0.000000000000000000 ) ) ;
#44662=ORIENTED_EDGE ( 'NONE', *, *, #93701, .F. ) ;
#44664=ORIENTED_EDGE ( 'NONE', *, *, #26998, .T. ) ;
#44666=VECTOR ( 'NONE', #13814, 1000.000000000000114 ) ;
#44667=DIRECTION ( 'NONE',  ( 0.000000000000000000, -0.000000000000000000, 1.000000000000000000 ) ) ;
#44669=ORIENTED_EDGE ( 'NONE', *, *, #6967, .T. ) ;
#44673=ORIENTED_EDGE ( 'NONE', *, *, #68143, .T. ) ;
#44676=DIRECTION ( 'NONE',  ( 0.000000000000000000, 0.000000000000000000, 1.000000000000000000 ) ) ;
#44678=VECTOR ( 'NONE', #69299, 1000.000000000000000 ) ;
#44679=ORIENTED_EDGE ( 'NONE', *, *, #81177, .T. ) ;
#44686=EDGE_CURVE ( 'NONE', #52414, #65850, #5124, .T. ) ;
#44698=VERTEX_POINT ( 'NONE', #20333 ) ;
#44717=CARTESIAN_POINT ( 'NONE',  ( -19.69645137954583802, 93.20008560620287597, 59.99999999999999289 ) ) ;
#44722=DIRECTION ( 'NONE',  ( 0.000000000000000000, 0.000000000000000000, 1.000000000000000000 ) ) ;
#44726=DIRECTION ( 'NONE',  ( -0.000000000000000000, -0.000000000000000000, -1.000000000000000000 ) ) ;
#44730=VERTEX_POINT ( 'NONE', #21320 ) ;
#44733=DIRECTION ( 'NONE',  ( -0.9981117208278914577, 0.06142469166373826922, 0.000000000000000000 ) ) ;
#44738=VECTOR ( 'NONE', #17432, 1000.000000000000000 ) ;
#44741=FACE_OUTER_BOUND ( 'NONE', #58960, .T. ) ;
#44767=CARTESIAN_POINT ( 'NONE',  ( 34.97213163436671124, 51.32435524152968753, -10.00000000000000000 ) ) ;
#44771=CARTESIAN_POINT ( 'NONE',  ( 48.53010236944518851, 101.9116055364396090, 10.00000000000000000 ) ) ;
#44774=CARTESIAN_POINT ( 'NONE',  ( -21.58168810074490551, 24.33735145887882112, -10.00000000000000000 ) ) ;
#44777=DIRECTION ( 'NONE',  ( -0.9086904199442051855, 0.4174706225611858335, 0.000000000000000000 ) ) ;
#44780=DIRECTION ( 'NONE',  ( -0.7082622432767082810, -0.7059494278973847958, 0.000000000000000000 ) ) ;
#44783=ORIENTED_EDGE ( 'NONE', *, *, #69873, .T. ) ;
#44789=CARTESIAN_POINT ( 'NONE',  ( 50.30020549591841927, 90.50945844122861672, 10.00000000000000000 ) ) ;
#44793=ORIENTED_EDGE ( 'NONE', *, *, #35071, .F. ) ;
#44796=AXIS2_PLACEMENT_3D ( 'NONE', #79624, #10187, #70994 ) ;
#44799=ORIENTED_EDGE ( 'NONE', *, *, #67248, .T. ) ;
#44803=DIRECTION ( 'NONE',  ( 0.000000000000000000, 0.000000000000000000, 1.000000000000000000 ) ) ;
#44808=DIRECTION ( 'NONE',  ( -0.7909930170786233505, 0.6118251767726273771, 0.000000000000000000 ) ) ;
#44810=DIRECTION ( 'NONE',  ( -0.000000000000000000, -0.000000000000000000, -1.000000000000000000 ) ) ;
#44815=VERTEX_POINT ( 'NONE', #99206 ) ;
#44818=ORIENTED_EDGE ( 'NONE', *, *, #6479, .T. ) ;
#44821=CARTESIAN_POINT ( 'NONE',  ( 49.28760614098965220, 105.1966139777580338, 10.00000000000000000 ) ) ;
#44824=EDGE_CURVE ( 'NONE', #40677, #91721, #45478, .T. ) ;
#44830=CARTESIAN_POINT ( 'NONE',  ( -22.85267942241863182, 23.13820207187276168, 10.00000000000000000 ) ) ;
#44831=DIRECTION ( 'NONE',  ( -0.000000000000000000, 0.000000000000000000, -1.000000000000000000 ) ) ;
#44848=ORIENTED_EDGE ( 'NONE', *, *, #10359, .T. ) ;
#44849=FACE_OUTER_BOUND ( 'NONE', #18524, .T. ) ;
#44851=DIRECTION ( 'NONE',  ( -0.6857383512133925496, -0.7278481391575704063, 0.000000000000000000 ) ) ;
#44860=PLANE ( 'NONE',  #35551 ) ;
#44861=VECTOR ( 'NONE', #52480, 1000.000000000000000 ) ;
#44863=VECTOR ( 'NONE', #48127, 1000.000000000000000 ) ;
#44867=CARTESIAN_POINT ( 'NONE',  ( -78.57153713424663977, 57.64153020465174393, -10.00000000000000000 ) ) ;
#44870=CARTESIAN_POINT ( 'NONE',  ( -19.65312891409030271, 93.06504152958497400, 10.00000000000000888 ) ) ;
#44871=FACE_OUTER_BOUND ( 'NONE', #18806, .T. ) ;
#44873=CARTESIAN_POINT ( 'NONE',  ( 48.91227514082039107, 78.96591507484178862, 10.00000000000000000 ) ) ;
#44882=DIRECTION ( 'NONE',  ( -0.1889875038809470387, -0.9819794923402672682, 0.000000000000000000 ) ) ;
#44884=PLANE ( 'NONE',  #12185 ) ;
#44888=VERTEX_POINT ( 'NONE', #38372 ) ;
#44905=DIRECTION ( 'NONE',  ( -0.1550826972584531394, -0.9879014915521905360, 0.000000000000000000 ) ) ;
#44909=ORIENTED_EDGE ( 'NONE', *, *, #26473, .T. ) ;
#44910=DIRECTION ( 'NONE',  ( 1.000000000000000000, 0.000000000000000000, 0.000000000000000000 ) ) ;
#44923=DIRECTION ( 'NONE',  ( 0.4552093898365224267, -0.8903844177683372108, 0.000000000000000000 ) ) ;
#44932=VECTOR ( 'NONE', #49102, 1000.000000000000000 ) ;
#44937=EDGE_CURVE ( 'NONE', #511, #96562, #92625, .T. ) ;
#44947=EDGE_CURVE ( 'NONE', #36501, #75140, #63184, .T. ) ;
#44954=ORIENTED_EDGE ( 'NONE', *, *, #23190, .T. ) ;
#44958=LINE ( 'NONE', #98698, #72173 ) ;
#44959=ORIENTED_EDGE ( 'NONE', *, *, #15891, .F. ) ;
#44961=AXIS2_PLACEMENT_3D ( 'NONE', #13555, #28742, #75357 ) ;
#44971=CARTESIAN_POINT ( 'NONE',  ( -44.26501565779586400, 27.25709555612339230, -10.00000000000000000 ) ) ;
#44977=CARTESIAN_POINT ( 'NONE',  ( -35.82302091652844922, 24.69132351629776423, 10.00000000000000000 ) ) ;
#44986=CARTESIAN_POINT ( 'NONE',  ( 5.783292089056025098, 27.85010085989870277, -10.00000000000000000 ) ) ;
#44993=CIRCLE ( 'NONE', #74108, 70.00000000000001421 ) ;
#45009=AXIS2_PLACEMENT_3D ( 'NONE', #43579, #74513, #13688 ) ;
#45015=CARTESIAN_POINT ( 'NONE',  ( -19.52224708177258705, 93.11966464384923370, 59.99999999999999289 ) ) ;
#45017=EDGE_CURVE ( 'NONE', #16029, #57256, #51092, .T. ) ;
#45024=VERTEX_POINT ( 'NONE', #81550 ) ;
#45026=CARTESIAN_POINT ( 'NONE',  ( -19.42194755839791753, 24.31068691715149299, -10.00000000000000000 ) ) ;
#45032=CARTESIAN_POINT ( 'NONE',  ( -19.65312891409030271, 93.06504152958497400, -10.00000000000000888 ) ) ;
#45041=ORIENTED_EDGE ( 'NONE', *, *, #28321, .F. ) ;
#45045=ORIENTED_EDGE ( 'NONE', *, *, #66044, .T. ) ;
#45048=EDGE_CURVE ( 'NONE', #35725, #58503, #34897, .T. ) ;
#45053=PLANE ( 'NONE',  #20536 ) ;
#45060=ORIENTED_EDGE ( 'NONE', *, *, #11296, .F. ) ;
#45064=AXIS2_PLACEMENT_3D ( 'NONE', #85023, #99704, #54068 ) ;
#45066=DIRECTION ( 'NONE',  ( -0.2433040867433108045, -0.9699500612784162090, 0.000000000000000000 ) ) ;
#45067=ORIENTED_EDGE ( 'NONE', *, *, #73547, .T. ) ;
#45069=FACE_BOUND ( 'NONE', #32693, .T. ) ;
#45080=AXIS2_PLACEMENT_3D ( 'NONE', #82918, #51979, #52964 ) ;
#45086=VECTOR ( 'NONE', #10337, 1000.000000000000000 ) ;
#45087=EDGE_CURVE ( 'NONE', #23902, #81619, #42983, .T. ) ;
#45090=CARTESIAN_POINT ( 'NONE',  ( -66.34925969370661392, 42.61035540433362456, 10.00000000000000000 ) ) ;
#45091=DIRECTION ( 'NONE',  ( -1.000000000000000000, 0.000000000000000000, 0.000000000000000000 ) ) ;
#45092=CIRCLE ( 'NONE', #92084, 70.00000000000001421 ) ;
#45098=CARTESIAN_POINT ( 'NONE',  ( 9.476883925432959543, 29.12856466152289414, 10.00000000000000000 ) ) ;
#45100=ORIENTED_EDGE ( 'NONE', *, *, #30655, .T. ) ;
#45102=AXIS2_PLACEMENT_3D ( 'NONE', #90840, #7168, #99891 ) ;
#45103=DIRECTION ( 'NONE',  ( 1.000000000000000000, 0.000000000000000000, 0.000000000000000000 ) ) ;
#45107=DIRECTION ( 'NONE',  ( -1.000000000000000000, 0.000000000000000000, 0.000000000000000000 ) ) ;
#45114=CARTESIAN_POINT ( 'NONE',  ( 30.68386671255119325, 44.42157463747831514, -10.00000000000000000 ) ) ;
#45121=ORIENTED_EDGE ( 'NONE', *, *, #70203, .T. ) ;
#45133=EDGE_CURVE ( 'NONE', #47298, #59964, #82059, .T. ) ;
#45141=EDGE_CURVE ( 'NONE', #15749, #84837, #55036, .T. ) ;
#45144=PLANE ( 'NONE',  #98338 ) ;
#45155=ORIENTED_EDGE ( 'NONE', *, *, #53279, .F. ) ;
#45156=AXIS2_PLACEMENT_3D ( 'NONE', #73986, #43042, #66371 ) ;
#45162=DIRECTION ( 'NONE',  ( -1.000000000000000000, 0.000000000000000000, 0.000000000000000000 ) ) ;
#45166=VECTOR ( 'NONE', #96697, 1000.000000000000114 ) ;
#45176=LINE ( 'NONE', #98905, #76610 ) ;
#45177=VECTOR ( 'NONE', #88966, 1000.000000000000000 ) ;
#45178=ORIENTED_EDGE ( 'NONE', *, *, #18879, .F. ) ;
#45181=EDGE_LOOP ( 'NONE', ( #1324, #32663, #5972, #75340 ) ) ;
#45184=VERTEX_POINT ( 'NONE', #79893 ) ;
#45185=CARTESIAN_POINT ( 'NONE',  ( -14.94286098042907440, 73.02398837676157939, 13.77360950052949917 ) ) ;
#45190=ORIENTED_EDGE ( 'NONE', *, *, #78225, .F. ) ;
#45203=PLANE ( 'NONE',  #58997 ) ;
#45207=VERTEX_POINT ( 'NONE', #26158 ) ;
#45211=LINE ( 'NONE', #78635, #5322 ) ;
#45234=PLANE ( 'NONE',  #33628 ) ;
#45235=CARTESIAN_POINT ( 'NONE',  ( -53.68831936616818723, 31.89637462494507858, 177.5919119679930134 ) ) ;
#45238=AXIS2_PLACEMENT_3D ( 'NONE', #38005, #39498, #70425 ) ;
#45242=LINE ( 'NONE', #28053, #98266 ) ;
#45246=VECTOR ( 'NONE', #21624, 999.9999999999998863 ) ;
#45251=CARTESIAN_POINT ( 'NONE',  ( -62.95439910331221256, 68.06504152958493137, 45.00000000000000711 ) ) ;
#45256=VECTOR ( 'NONE', #62807, 1000.000000000000114 ) ;
#45272=ORIENTED_EDGE ( 'NONE', *, *, #9843, .F. ) ;
#45273=DIRECTION ( 'NONE',  ( -0.000000000000000000, -0.000000000000000000, -1.000000000000000000 ) ) ;
#45277=EDGE_LOOP ( 'NONE', ( #89043, #11870, #38432, #14638 ) ) ;
#45290=ORIENTED_EDGE ( 'NONE', *, *, #82639, .T. ) ;
#45292=DIRECTION ( 'NONE',  ( 0.8718556560469403749, 0.4897629171537585813, 0.000000000000000000 ) ) ;
#45295=VECTOR ( 'NONE', #71261, 1000.000000000000000 ) ;
#45303=DIRECTION ( 'NONE',  ( 0.000000000000000000, 0.000000000000000000, 1.000000000000000000 ) ) ;
#45308=ORIENTED_EDGE ( 'NONE', *, *, #93638, .T. ) ;
#45313=ORIENTED_EDGE ( 'NONE', *, *, #59808, .T. ) ;
#45322=EDGE_CURVE ( 'NONE', #84457, #34967, #52503, .T. ) ;
#45326=ORIENTED_EDGE ( 'NONE', *, *, #68501, .F. ) ;
#45334=ORIENTED_EDGE ( 'NONE', *, *, #10382, .F. ) ;
#45339=EDGE_CURVE ( 'NONE', #35809, #30665, #50918, .T. ) ;
#45350=EDGE_LOOP ( 'NONE', ( #49864, #16884, #95577, #47286 ) ) ;
#45351=CARTESIAN_POINT ( 'NONE',  ( 22.45462004596304695, 37.14601545153948337, 177.5919119679930134 ) ) ;
#45354=DIRECTION ( 'NONE',  ( 0.000000000000000000, -0.000000000000000000, 1.000000000000000000 ) ) ;
#45355=LINE ( 'NONE', #53450, #37217 ) ;
#45376=DIRECTION ( 'NONE',  ( 0.4174706225611763410, 0.9086904199442095154, 0.000000000000000000 ) ) ;
#45377=CIRCLE ( 'NONE', #24342, 70.00000000000001421 ) ;
#45378=EDGE_CURVE ( 'NONE', #39135, #19773, #52429, .T. ) ;
#45398=EDGE_CURVE ( 'NONE', #23843, #76681, #7837, .T. ) ;
#45400=ORIENTED_EDGE ( 'NONE', *, *, #48604, .T. ) ;
#45411=VERTEX_POINT ( 'NONE', #38205 ) ;
#45424=DIRECTION ( 'NONE',  ( 0.000000000000000000, 0.000000000000000000, 1.000000000000000000 ) ) ;
#45437=VERTEX_POINT ( 'NONE', #37716 ) ;
#45438=DIRECTION ( 'NONE',  ( 0.000000000000000000, 0.000000000000000000, -1.000000000000000000 ) ) ;
#45440=CARTESIAN_POINT ( 'NONE',  ( -19.02615211706134701, 34.39283837976707048, 59.99999999999999289 ) ) ;
#45441=VERTEX_POINT ( 'NONE', #30637 ) ;
#45449=LINE ( 'NONE', #61145, #33410 ) ;
#45452=VECTOR ( 'NONE', #77248, 1000.000000000000114 ) ;
#45464=VERTEX_POINT ( 'NONE', #10344 ) ;
#45472=EDGE_CURVE ( 'NONE', #90523, #93301, #21782, .T. ) ;
#45478=LINE ( 'NONE', #53087, #78348 ) ;
#45480=CARTESIAN_POINT ( 'NONE',  ( -6.281727404287059890, 25.63055774385195917, -10.00000000000000000 ) ) ;
#45507=EDGE_CURVE ( 'NONE', #27844, #39666, #78419, .T. ) ;
#45511=CIRCLE ( 'NONE', #6703, 70.00000000000001421 ) ;
#45521=CARTESIAN_POINT ( 'NONE',  ( -50.31241255605538498, 43.89631431014924345, 59.99999999999999289 ) ) ;
#45522=VERTEX_POINT ( 'NONE', #66028 ) ;
#45531=DIRECTION ( 'NONE',  ( -0.8614378286617615510, 0.5078630399532039208, 0.000000000000000000 ) ) ;
#45532=VERTEX_POINT ( 'NONE', #41718 ) ;
#45550=ORIENTED_EDGE ( 'NONE', *, *, #20471, .T. ) ;
#45553=PLANE ( 'NONE',  #43113 ) ;
#45559=FACE_BOUND ( 'NONE', #3362, .T. ) ;
#45566=FACE_OUTER_BOUND ( 'NONE', #81394, .T. ) ;
#45568=ORIENTED_EDGE ( 'NONE', *, *, #27888, .T. ) ;
#45570=ORIENTED_EDGE ( 'NONE', *, *, #75666, .F. ) ;
#45572=EDGE_CURVE ( 'NONE', #10579, #47882, #2420, .T. ) ;
#45579=DIRECTION ( 'NONE',  ( -0.1384676192453732635, 0.9903669614948382716, 0.000000000000000000 ) ) ;
#45583=EDGE_CURVE ( 'NONE', #93683, #27723, #51305, .T. ) ;
#45586=DIRECTION ( 'NONE',  ( -0.9919422576440838357, -0.1266907948509199411, 0.000000000000000000 ) ) ;
#45587=ORIENTED_EDGE ( 'NONE', *, *, #61883, .F. ) ;
#45596=FACE_OUTER_BOUND ( 'NONE', #77541, .T. ) ;
#45600=CARTESIAN_POINT ( 'NONE',  ( -11.40312891409031693, 78.77562236714182120, 59.99999999999999289 ) ) ;
#45602=DIRECTION ( 'NONE',  ( -0.5104483989331241034, -0.8599083858334038988, 0.000000000000000000 ) ) ;
#45604=EDGE_CURVE ( 'NONE', #81025, #87907, #3258, .T. ) ;
#45607=ORIENTED_EDGE ( 'NONE', *, *, #57359, .F. ) ;
#45613=VECTOR ( 'NONE', #6558, 1000.000000000000227 ) ;
#45619=EDGE_CURVE ( 'NONE', #85223, #84967, #81273, .T. ) ;
#45629=CARTESIAN_POINT ( 'NONE',  ( 48.98810889288134263, 89.24608170897542436, -10.00000000000000000 ) ) ;
#45632=CARTESIAN_POINT ( 'NONE',  ( 47.28113444070024229, 72.57591296950349147, 177.5919119679930134 ) ) ;
#45641=PLANE ( 'NONE',  #98764 ) ;
#45651=EDGE_LOOP ( 'NONE', ( #72135, #43080, #35322, #91208 ) ) ;
#45653=CARTESIAN_POINT ( 'NONE',  ( 50.23025173566474422, 97.10399052176643409, 177.5919119679930134 ) ) ;
#45654=CARTESIAN_POINT ( 'NONE',  ( 50.12332653952445582, 98.65487733484057742, 10.00000000000000000 ) ) ;
#45660=EDGE_CURVE ( 'NONE', #7803, #45437, #53786, .T. ) ;
#45664=ORIENTED_EDGE ( 'NONE', *, *, #39458, .T. ) ;
#45667=ORIENTED_EDGE ( 'NONE', *, *, #81431, .F. ) ;
#45675=ORIENTED_EDGE ( 'NONE', *, *, #10593, .T. ) ;
#45676=VERTEX_POINT ( 'NONE', #90872 ) ;
#45681=LINE ( 'NONE', #53778, #82533 ) ;
#45686=AXIS2_PLACEMENT_3D ( 'NONE', #54716, #48650, #93780 ) ;
#45697=EDGE_CURVE ( 'NONE', #80286, #84464, #98936, .T. ) ;
#45699=CARTESIAN_POINT ( 'NONE',  ( 12.00096474099108690, 32.03863464977599307, 10.00000000000000000 ) ) ;
#45705=ADVANCED_FACE ( 'NONE', ( #84747 ), #45203, .F. ) ;
#45711=AXIS2_PLACEMENT_3D ( 'NONE', #46502, #8527, #7510 ) ;
#45729=ORIENTED_EDGE ( 'NONE', *, *, #92641, .F. ) ;
#45737=DIRECTION ( 'NONE',  ( -0.7957378174433876739, 0.6056412518070690698, 0.000000000000000000 ) ) ;
#45754=DIRECTION ( 'NONE',  ( -0.9055221650797476984, -0.4242989612870696758, 0.000000000000000000 ) ) ;
#45755=ORIENTED_EDGE ( 'NONE', *, *, #96175, .T. ) ;
#45756=DIRECTION ( 'NONE',  ( -0.03304531753667278721, -0.9994538543569185807, 0.000000000000000000 ) ) ;
#45758=EDGE_CURVE ( 'NONE', #62226, #6303, #55778, .T. ) ;
#45760=CIRCLE ( 'NONE', #66755, 70.00000000000001421 ) ;
#45766=VECTOR ( 'NONE', #1173, 1000.000000000000114 ) ;
#45781=VECTOR ( 'NONE', #42902, 1000.000000000000000 ) ;
#45785=ORIENTED_EDGE ( 'NONE', *, *, #38722, .F. ) ;
#45792=VERTEX_POINT ( 'NONE', #46703 ) ;
#45793=ORIENTED_EDGE ( 'NONE', *, *, #14742, .F. ) ;
#45803=ORIENTED_EDGE ( 'NONE', *, *, #27289, .T. ) ;
#45811=FACE_OUTER_BOUND ( 'NONE', #57752, .T. ) ;
#45812=EDGE_CURVE ( 'NONE', #68464, #82593, #78123, .T. ) ;
#45820=DIRECTION ( 'NONE',  ( -0.9606745773021556634, 0.2776767122488391082, 0.000000000000000000 ) ) ;
#45824=DIRECTION ( 'NONE',  ( 0.3958915996110438096, 0.9182972510888884887, 0.000000000000000000 ) ) ;
#45833=FACE_OUTER_BOUND ( 'NONE', #19433, .T. ) ;
#45840=AXIS2_PLACEMENT_3D ( 'NONE', #16728, #63327, #94268 ) ;
#45845=CIRCLE ( 'NONE', #26513, 70.00000000000001421 ) ;
#45852=LINE ( 'NONE', #91028, #82207 ) ;
#45859=DIRECTION ( 'NONE',  ( -0.4340522123146846045, 0.9008877160804935613, 0.000000000000000000 ) ) ;
#45880=CARTESIAN_POINT ( 'NONE',  ( 43.24043327773039636, 120.8247932685368227, -10.00000000000000000 ) ) ;
#45891=EDGE_CURVE ( 'NONE', #66403, #54956, #26418, .T. ) ;
#45901=DIRECTION ( 'NONE',  ( -0.8099771808667466377, -0.5864613938488684175, 0.000000000000000000 ) ) ;
#45904=LINE ( 'NONE', #75865, #87059 ) ;
#45905=VERTEX_POINT ( 'NONE', #81155 ) ;
#45907=VERTEX_POINT ( 'NONE', #18324 ) ;
#45908=AXIS2_PLACEMENT_3D ( 'NONE', #56765, #3588, #48686 ) ;
#45909=ORIENTED_EDGE ( 'NONE', *, *, #83109, .T. ) ;
#45921=VECTOR ( 'NONE', #62736, 1000.000000000000114 ) ;
#45936=CARTESIAN_POINT ( 'NONE',  ( 46.50192534792603283, 74.36443251879779837, -10.00000000000000000 ) ) ;
#45941=LINE ( 'NONE', #91109, #991 ) ;
#45944=EDGE_CURVE ( 'NONE', #29881, #74122, #4101, .T. ) ;
#45950=DIRECTION ( 'NONE',  ( -0.6833540297821713017, 0.7300871660154474307, 0.000000000000000000 ) ) ;
#45955=CARTESIAN_POINT ( 'NONE',  ( -19.65312891409030271, 93.06504152958497400, 10.00000000000000888 ) ) ;
#45958=DIRECTION ( 'NONE',  ( -0.000000000000000000, -0.000000000000000000, -1.000000000000000000 ) ) ;
#45973=FACE_OUTER_BOUND ( 'NONE', #50141, .T. ) ;
#45980=LINE ( 'NONE', #21224, #53065 ) ;
#45981=VECTOR ( 'NONE', #2863, 1000.000000000000000 ) ;
#45985=CARTESIAN_POINT ( 'NONE',  ( -53.02163307513389867, 51.85713630120221751, 59.99999999999999289 ) ) ;
#45986=EDGE_CURVE ( 'NONE', #1733, #74953, #97330, .T. ) ;
#45989=DIRECTION ( 'NONE',  ( -0.000000000000000000, 0.000000000000000000, -1.000000000000000000 ) ) ;
#45992=CARTESIAN_POINT ( 'NONE',  ( -40.95769633352519890, 38.39369580655643688, 59.99999999999999289 ) ) ;
#45997=EDGE_CURVE ( 'NONE', #9815, #72762, #96851, .T. ) ;
#46009=EDGE_CURVE ( 'NONE', #14998, #8310, #31524, .T. ) ;
#46010=CARTESIAN_POINT ( 'NONE',  ( -75.57215499213535281, 50.95729256953105590, 10.00000000000000000 ) ) ;
#46011=ORIENTED_EDGE ( 'NONE', *, *, #12807, .F. ) ;
#46023=VERTEX_POINT ( 'NONE', #60763 ) ;
#46027=EDGE_LOOP ( 'NONE', ( #19449, #13387, #66237, #8314, #65829, #78849, #47306, #30113, #2726, #66004, #86875, #51892, #6314, #92196, #51556, #31052, #92519, #27877, #42656, #77456, #14387, #26247, #41450, #42566, #82489, #61346, #74368, #54379, #35501, #80325, #60709, #41193, #7777, #77512, #20934, #100139, #40169, #47329, #75719, #74623, #88109, #93097, #11701, #62029, #64742, #59773, #5962, #19299, #72236, #20673, #2497, #81852, #83962, #12189, #59079, #26990, #48813, #10589, #78986, #55619, #19975, #30853, #53748, #472, #11536, #60903, #40747, #39163, #58479, #91304, #55763, #46273, #18918, #15162, #83716, #13826, #84507, #70479, #52424, #56039, #38336, #9851, #94611, #12739, #23475, #57427, #48919, #94702, #75385, #72735, #29163, #96972, #80166, #29383, #89529, #43289, #83791, #60464, #70710, #19425, #13791, #29291, #64149, #68727, #58515, #80525, #53689, #82235, #15018, #66736, #49660, #82008, #19942, #26423, #11464, #62503, #30117, #23613, #15015, #20075, #83509, #28019, #51798, #50051, #37925, #93231, #38556, #43035, #99179, #12852, #73857, #91814, #24546, #95366, #55504, #97475, #19645, #50656, #1844, #12464, #74053, #6339, #14137, #2714, #53825, #62813, #42333, #87928, #43013, #36480, #35534, #79103, #77984, #98578, #95282, #94090, #13663, #22859, #15433, #40307, #17679, #70000, #82911, #10843, #66624, #17976, #45190, #33746, #97397, #45155, #99530, #69491, #64776, #68113, #205, #5928, #31589, #13540, #16633, #20641, #72366, #45793, #68487, #45550, #7268, #71161, #12319, #49801, #30625, #14782, #78503, #81864, #16406, #92558, #83229, #30690, #15396, #45272, #40698, #5740, #60951, #47034, #55458, #96082, #88970, #34927, #78509, #36698, #60213, #89913, #63358, #17673, #42196, #41815, #40797, #45400, #82756, #93954, #68366, #68389, #95186, #41465, #63462, #83106, #17642, #17126, #94189, #33452, #59085, #53893, #67771, #66270, #71898, #63563, #76104, #36812, #81617, #73277, #89976, #7213, #96185, #19156, #74647, #12859, #54604, #73593, #7679, #79130, #39560, #42250, #2589, #16183, #92316, #37435, #29218, #34107, #88897, #89259, #41100, #32596, #21493, #35379, #31080, #70373, #22270, #67985, #89283, #75220, #7294, #34151, #15110, #18030, #88745, #87278, #31967, #33098, #19037, #99899, #24176, #94582, #32367, #64270, #97537, #70693, #71973, #79630, #27185, #4362, #51060, #38801, #34874, #37427, #96156, #31741, #57153, #79115, #30399, #68225, #25141, #32630, #575, #20475, #87183, #58436, #76281, #51794, #33622, #49635, #35770, #38346, #22545, #39323, #35929, #8662, #36607, #74279, #62484, #100256, #58414, #51948, #41948, #91700, #80298, #6787, #22536, #31632, #20783, #39304, #67743, #68728, #79905, #95332, #54683, #88808, #4700, #57747, #54749, #87283, #70728, #44954, #60798, #16720, #69369, #16690, #46960, #97291, #39087, #38230, #55860, #42804, #39422, #12295, #81035, #89122, #80750, #24641, #85817, #34634, #82262, #14149, #96656, #96229, #44516, #54260, #25224, #76977, #46512, #59498, #99415, #20290, #94673, #4951, #99681, #95849, #94956, #48056, #8657, #74405, #65015, #81746, #36226, #41546, #52360, #28731, #3001, #83342, #67218, #87362, #42799, #80359, #23489, #44186, #65484, #37545, #92942, #43689, #33059, #57506, #44465, #56898, #18645, #74505, #63382, #36491 ) ) ;
#46028=CARTESIAN_POINT ( 'NONE',  ( 27.92801399040350319, 72.76188621587162686, 59.99999999999999289 ) ) ;
#46046=DIRECTION ( 'NONE',  ( -0.09573633691164462611, -0.9954067278227227700, 0.000000000000000000 ) ) ;
#46048=ORIENTED_EDGE ( 'NONE', *, *, #63337, .F. ) ;
#46049=EDGE_CURVE ( 'NONE', #71264, #79283, #20820, .T. ) ;
#46050=CARTESIAN_POINT ( 'NONE',  ( -19.65312891409030271, 93.06504152958497400, 59.99999999999999289 ) ) ;
#46054=FACE_OUTER_BOUND ( 'NONE', #81093, .T. ) ;
#46059=VECTOR ( 'NONE', #29032, 1000.000000000000000 ) ;
#46064=VECTOR ( 'NONE', #56747, 1000.000000000000000 ) ;
#46073=EDGE_CURVE ( 'NONE', #22887, #83079, #1995, .T. ) ;
#46080=ORIENTED_EDGE ( 'NONE', *, *, #92511, .T. ) ;
#46087=ORIENTED_EDGE ( 'NONE', *, *, #36576, .T. ) ;
#46090=VECTOR ( 'NONE', #9291, 1000.000000000000227 ) ;
#46092=CARTESIAN_POINT ( 'NONE',  ( -66.34925969370661392, 42.61035540433362456, 10.00000000000000000 ) ) ;
#46095=DIRECTION ( 'NONE',  ( 0.000000000000000000, 0.000000000000000000, 1.000000000000000000 ) ) ;
#46097=CARTESIAN_POINT ( 'NONE',  ( -31.59160691316810343, 24.09060609829247568, -10.00000000000000000 ) ) ;
#46104=CARTESIAN_POINT ( 'NONE',  ( -29.91485116994501325, 25.08783183303773967, -10.00000000000000000 ) ) ;
#46113=CARTESIAN_POINT ( 'NONE',  ( -52.83961229143921656, 94.84783475815204667, -10.00000000000000000 ) ) ;
#46123=CIRCLE ( 'NONE', #18693, 70.00000000000001421 ) ;
#46131=CARTESIAN_POINT ( 'NONE',  ( -68.10632939235270555, 44.28490124273479012, -10.00000000000000000 ) ) ;
#46143=EDGE_CURVE ( 'NONE', #21282, #99967, #15169, .T. ) ;
#46145=ORIENTED_EDGE ( 'NONE', *, *, #4718, .F. ) ;
#46146=VERTEX_POINT ( 'NONE', #62776 ) ;
#46149=ORIENTED_EDGE ( 'NONE', *, *, #98556, .T. ) ;
#46160=ORIENTED_EDGE ( 'NONE', *, *, #6151, .T. ) ;
#46162=CARTESIAN_POINT ( 'NONE',  ( -1.588913428802907202, 65.16871292612921707, -10.00000000000000000 ) ) ;
#46164=CARTESIAN_POINT ( 'NONE',  ( -14.36410898293827998, 72.70576163098405686, 13.91634736112990645 ) ) ;
#46166=DIRECTION ( 'NONE',  ( -0.009162850352631533510, 0.9999580202055560196, 0.000000000000000000 ) ) ;
#46167=VECTOR ( 'NONE', #58410, 1000.000000000000000 ) ;
#46169=VERTEX_POINT ( 'NONE', #86648 ) ;
#46171=ADVANCED_FACE ( 'NONE', ( #47579 ), #16191, .T. ) ;
#46189=AXIS2_PLACEMENT_3D ( 'NONE', #96295, #59221, #35945 ) ;
#46193=CARTESIAN_POINT ( 'NONE',  ( -76.23101443460923576, 54.01191295053621388, -10.00000000000000000 ) ) ;
#46204=LINE ( 'NONE', #14823, #43199 ) ;
#46210=ORIENTED_EDGE ( 'NONE', *, *, #61176, .T. ) ;
#46214=LINE ( 'NONE', #54827, #17507 ) ;
#46255=DIRECTION ( 'NONE',  ( 0.000000000000000000, -0.000000000000000000, 1.000000000000000000 ) ) ;
#46257=VECTOR ( 'NONE', #5996, 1000.000000000000000 ) ;
#46259=EDGE_CURVE ( 'NONE', #56418, #31865, #2506, .T. ) ;
#46262=CARTESIAN_POINT ( 'NONE',  ( -19.64260764713147012, 93.20647363903802329, 59.99999999999999289 ) ) ;
#46266=EDGE_LOOP ( 'NONE', ( #40449, #26862, #23490, #52510 ) ) ;
#46273=ORIENTED_EDGE ( 'NONE', *, *, #55410, .T. ) ;
#46278=EDGE_LOOP ( 'NONE', ( #77574, #25505, #52908, #47791 ) ) ;
#46284=VERTEX_POINT ( 'NONE', #18200 ) ;
#46285=ORIENTED_EDGE ( 'NONE', *, *, #51710, .F. ) ;
#46287=ORIENTED_EDGE ( 'NONE', *, *, #77073, .T. ) ;
#46289=ORIENTED_EDGE ( 'NONE', *, *, #32493, .T. ) ;
#46291=ADVANCED_FACE ( 'NONE', ( #41983 ), #49581, .T. ) ;
#46304=CARTESIAN_POINT ( 'NONE',  ( -40.08433460452723551, 25.84155934987275671, 10.00000000000000000 ) ) ;
#46305=VERTEX_POINT ( 'NONE', #49536 ) ;
#46324=EDGE_CURVE ( 'NONE', #97061, #89775, #78499, .T. ) ;
#46335=AXIS2_PLACEMENT_3D ( 'NONE', #8387, #39254, #47372 ) ;
#46368=CARTESIAN_POINT ( 'NONE',  ( -2.330697855141256269, 26.52822386297705393, 10.00000000000000000 ) ) ;
#46369=DIRECTION ( 'NONE',  ( -1.000000000000000000, 0.000000000000000000, 0.000000000000000000 ) ) ;
#46370=LINE ( 'NONE', #24089, #28362 ) ;
#46372=DIRECTION ( 'NONE',  ( -0.000000000000000000, -0.000000000000000000, -1.000000000000000000 ) ) ;
#46378=AXIS2_PLACEMENT_3D ( 'NONE', #49552, #90093, #96199 ) ;
#46388=ADVANCED_FACE ( 'NONE', ( #73353 ), #34824, .F. ) ;
#46399=DIRECTION ( 'NONE',  ( -0.4897629171537585258, 0.8718556560469402639, 0.000000000000000000 ) ) ;
#46400=ORIENTED_EDGE ( 'NONE', *, *, #14043, .F. ) ;
#46408=VECTOR ( 'NONE', #51716, 1000.000000000000000 ) ;
#46410=EDGE_LOOP ( 'NONE', ( #7065, #9573, #21198, #73495 ) ) ;
#46412=VECTOR ( 'NONE', #3597, 1000.000000000000000 ) ;
#46432=DIRECTION ( 'NONE',  ( -0.8653701635463872943, 0.5011331959107268030, 0.000000000000000000 ) ) ;
#46439=ORIENTED_EDGE ( 'NONE', *, *, #54078, .F. ) ;
#46447=VECTOR ( 'NONE', #53474, 1000.000000000000000 ) ;
#46448=EDGE_CURVE ( 'NONE', #63646, #93711, #88107, .T. ) ;
#46451=PLANE ( 'NONE',  #26956 ) ;
#46454=AXIS2_PLACEMENT_3D ( 'NONE', #18867, #11278, #64960 ) ;
#46460=CARTESIAN_POINT ( 'NONE',  ( -19.65312891409030271, 93.06504152958497400, 59.99999999999999289 ) ) ;
#46464=AXIS2_PLACEMENT_3D ( 'NONE', #52190, #92250, #99317 ) ;
#46465=DIRECTION ( 'NONE',  ( -0.9997524133706772176, 0.02225111142182466945, 0.000000000000000000 ) ) ;
#46476=CIRCLE ( 'NONE', #90225, 0.1418229129684159262 ) ;
#46480=LINE ( 'NONE', #53585, #85461 ) ;
#46485=DIRECTION ( 'NONE',  ( -0.7696402260561131525, -0.6384778167143280170, 0.000000000000000000 ) ) ;
#46502=CARTESIAN_POINT ( 'NONE',  ( 45.66470909604093720, 114.5311720768849995, -10.00000000000000000 ) ) ;
#46505=DIRECTION ( 'NONE',  ( 1.000000000000000000, 0.000000000000000000, 0.000000000000000000 ) ) ;
#46509=ORIENTED_EDGE ( 'NONE', *, *, #14609, .F. ) ;
#46512=ORIENTED_EDGE ( 'NONE', *, *, #65746, .F. ) ;
#46522=ORIENTED_EDGE ( 'NONE', *, *, #79482, .F. ) ;
#46523=CIRCLE ( 'NONE', #75704, 70.00000000000001421 ) ;
#46529=DIRECTION ( 'NONE',  ( 0.000000000000000000, 0.000000000000000000, 1.000000000000000000 ) ) ;
#46530=CARTESIAN_POINT ( 'NONE',  ( 44.18536904650256503, 64.34838820550514527, 10.00000000000000000 ) ) ;
#46532=CYLINDRICAL_SURFACE ( 'NONE', #16867, 70.00000000000002842 ) ;
#46533=CIRCLE ( 'NONE', #48135, 70.00000000000001421 ) ;
#46542=CIRCLE ( 'NONE', #80597, 70.00000000000001421 ) ;
#46547=ORIENTED_EDGE ( 'NONE', *, *, #60001, .T. ) ;
#46550=ORIENTED_EDGE ( 'NONE', *, *, #13163, .F. ) ;
#46560=FACE_OUTER_BOUND ( 'NONE', #99022, .T. ) ;
#46563=AXIS2_PLACEMENT_3D ( 'NONE', #1919, #63710, #16109 ) ;
#46565=FACE_OUTER_BOUND ( 'NONE', #83868, .T. ) ;
#46574=ORIENTED_EDGE ( 'NONE', *, *, #90749, .T. ) ;
#46577=ADVANCED_FACE ( 'NONE', ( #78856 ), #8438, .F. ) ;
#46585=DIRECTION ( 'NONE',  ( -0.2502735827033141236, -0.9681751565707764628, 0.000000000000000000 ) ) ;
#46588=CARTESIAN_POINT ( 'NONE',  ( -44.30466402961319972, 27.54938068083718861, -10.00000000000000000 ) ) ;
#46591=ORIENTED_EDGE ( 'NONE', *, *, #27213, .F. ) ;
#46594=AXIS2_PLACEMENT_3D ( 'NONE', #3240, #34605, #65503 ) ;
#46595=AXIS2_PLACEMENT_3D ( 'NONE', #3496, #42451, #33900 ) ;
#46596=DIRECTION ( 'NONE',  ( 0.02977611660965746171, -0.9995565931350001154, 0.000000000000000000 ) ) ;
#46600=APPLICATION_CONTEXT ( 'automotive_design' ) ;
#46602=EDGE_CURVE ( 'NONE', #82505, #63013, #20275, .T. ) ;
#46628=ADVANCED_FACE ( 'NONE', ( #89967 ), #20547, .T. ) ;
#46632=AXIS2_PLACEMENT_3D ( 'NONE', #81795, #3288, #42732 ) ;
#46635=FACE_OUTER_BOUND ( 'NONE', #25247, .T. ) ;
#46636=CARTESIAN_POINT ( 'NONE',  ( -59.65739779450132829, 37.15562860896454112, 10.00000000000000000 ) ) ;
#46640=EDGE_CURVE ( 'NONE', #12952, #52938, #68773, .T. ) ;
#46643=DIRECTION ( 'NONE',  ( -0.1696015684586882066, -0.9855127132494805320, 0.000000000000000000 ) ) ;
#46649=ORIENTED_EDGE ( 'NONE', *, *, #43760, .T. ) ;
#46656=DIRECTION ( 'NONE',  ( -0.7005979833698863235, -0.7135562106085605594, 0.000000000000000000 ) ) ;
#46663=CARTESIAN_POINT ( 'NONE',  ( -55.13986305262019982, 55.42364176852501600, 59.99999999999999289 ) ) ;
#46673=AXIS2_PLACEMENT_3D ( 'NONE', #42342, #28152, #35754 ) ;
#46674=DIRECTION ( 'NONE',  ( 1.000000000000000000, 0.000000000000000000, 0.000000000000000000 ) ) ;
#46684=CARTESIAN_POINT ( 'NONE',  ( -4.653128914090328472, 78.77562236714182120, 13.81405534229504717 ) ) ;
#46686=LINE ( 'NONE', #76598, #19182 ) ;
#46693=DIRECTION ( 'NONE',  ( 0.1550826972584426755, 0.9879014915521923124, 0.000000000000000000 ) ) ;
#46702=DIRECTION ( 'NONE',  ( -0.8279987035736640077, -0.5607300124661883656, 0.000000000000000000 ) ) ;
#46703=CARTESIAN_POINT ( 'NONE',  ( 43.24043327773040346, 120.8247932685368227, -10.00000000000000000 ) ) ;
#46707=ORIENTED_EDGE ( 'NONE', *, *, #39203, .F. ) ;
#46715=ORIENTED_EDGE ( 'NONE', *, *, #45986, .T. ) ;
#46724=DIRECTION ( 'NONE',  ( 0.000000000000000000, 0.000000000000000000, 1.000000000000000000 ) ) ;
#46733=DIRECTION ( 'NONE',  ( -0.000000000000000000, -0.000000000000000000, 1.000000000000000000 ) ) ;
#46738=AXIS2_PLACEMENT_3D ( 'NONE', #100064, #85911, #39708 ) ;
#46739=CARTESIAN_POINT ( 'NONE',  ( -10.80656490723494123, 24.88181024604956804, -10.00000000000000000 ) ) ;
#46741=VECTOR ( 'NONE', #21591, 1000.000000000000000 ) ;
#46751=CARTESIAN_POINT ( 'NONE',  ( -76.86719868626529717, 52.73452925779879763, -10.00000000000000000 ) ) ;
#46760=AXIS2_PLACEMENT_3D ( 'NONE', #96065, #20525, #27130 ) ;
#46771=EDGE_CURVE ( 'NONE', #3544, #40063, #77210, .T. ) ;
#46774=DIRECTION ( 'NONE',  ( -0.4272584830711199100, -0.9041295198387040433, 0.000000000000000000 ) ) ;
#46779=VECTOR ( 'NONE', #4278, 1000.000000000000000 ) ;
#46783=EDGE_CURVE ( 'NONE', #69110, #35956, #81771, .T. ) ;
#46791=VERTEX_POINT ( 'NONE', #56893 ) ;
#46796=EDGE_LOOP ( 'NONE', ( #66643, #68651, #25539, #66358 ) ) ;
#46797=CARTESIAN_POINT ( 'NONE',  ( -75.14068524134967220, 52.46521621197197760, -10.00000000000000000 ) ) ;
#46808=ORIENTED_EDGE ( 'NONE', *, *, #24012, .F. ) ;
#46818=EDGE_CURVE ( 'NONE', #20252, #11356, #24504, .T. ) ;
#46820=AXIS2_PLACEMENT_3D ( 'NONE', #49924, #80881, #72246 ) ;
#46823=PLANE ( 'NONE',  #49590 ) ;
#46827=VECTOR ( 'NONE', #7373, 1000.000000000000000 ) ;
#46829=ORIENTED_EDGE ( 'NONE', *, *, #59102, .T. ) ;
#46833=FACE_OUTER_BOUND ( 'NONE', #49195, .T. ) ;
#46837=EDGE_LOOP ( 'NONE', ( #92458, #70604, #17007, #96951 ) ) ;
#46840=CARTESIAN_POINT ( 'NONE',  ( -16.25778278694858869, 23.14743555886464321, 177.5919119679930134 ) ) ;
#46852=ORIENTED_EDGE ( 'NONE', *, *, #16877, .T. ) ;
#46853=VERTEX_POINT ( 'NONE', #54898 ) ;
#46855=EDGE_CURVE ( 'NONE', #81160, #10579, #10319, .T. ) ;
#46856=DIRECTION ( 'NONE',  ( -0.7280311630581435267, -0.6855440362341479466, 0.000000000000000000 ) ) ;
#46857=EDGE_CURVE ( 'NONE', #35590, #38181, #77728, .T. ) ;
#46868=LINE ( 'NONE', #47361, #26571 ) ;
#46886=VECTOR ( 'NONE', #43070, 1000.000000000000000 ) ;
#46887=CARTESIAN_POINT ( 'NONE',  ( 44.98086946945896614, 119.9434018396067785, -10.00000000000000000 ) ) ;
#46889=LINE ( 'NONE', #47870, #65167 ) ;
#46905=VECTOR ( 'NONE', #21205, 1000.000000000000000 ) ;
#46907=VERTEX_POINT ( 'NONE', #41188 ) ;
#46913=CARTESIAN_POINT ( 'NONE',  ( -52.33464467766007289, 32.58262665401804270, 10.00000000000000000 ) ) ;
#46917=CARTESIAN_POINT ( 'NONE',  ( -50.27375324258477463, 105.9839577528636738, -10.00000000000000000 ) ) ;
#46919=DIRECTION ( 'NONE',  ( -1.000000000000000000, 0.000000000000000000, 0.000000000000000000 ) ) ;
#46920=EDGE_CURVE ( 'NONE', #1592, #72762, #33204, .T. ) ;
#46922=PLANE ( 'NONE',  #72353 ) ;
#46942=LINE ( 'NONE', #54514, #19456 ) ;
#46955=CARTESIAN_POINT ( 'NONE',  ( -22.85267942241863182, 23.13820207187276168, -10.00000000000000000 ) ) ;
#46957=CARTESIAN_POINT ( 'NONE',  ( -14.83894680564148238, 24.48641780169620219, 10.00000000000000000 ) ) ;
#46958=LINE ( 'NONE', #77876, #64129 ) ;
#46960=ORIENTED_EDGE ( 'NONE', *, *, #7740, .F. ) ;
#46973=ORIENTED_EDGE ( 'NONE', *, *, #22163, .F. ) ;
#46979=EDGE_CURVE ( 'NONE', #42396, #80773, #3237, .T. ) ;
#46982=ADVANCED_FACE ( 'NONE', ( #34121 ), #81742, .T. ) ;
#46993=EDGE_CURVE ( 'NONE', #99166, #54753, #42682, .T. ) ;
#46996=DIRECTION ( 'NONE',  ( -1.000000000000000000, 0.000000000000000000, 0.000000000000000000 ) ) ;
#47006=CARTESIAN_POINT ( 'NONE',  ( -19.65312891409030271, 93.06504152958497400, 177.5919119679930134 ) ) ;
#47034=ORIENTED_EDGE ( 'NONE', *, *, #13996, .F. ) ;
#47039=CARTESIAN_POINT ( 'NONE',  ( 7.819191540449068611, 28.68125778831127803, 177.5919119679930134 ) ) ;
#47049=ORIENTED_EDGE ( 'NONE', *, *, #7400, .F. ) ;
#47063=ORIENTED_EDGE ( 'NONE', *, *, #55574, .F. ) ;
#47072=DIRECTION ( 'NONE',  ( -0.000000000000000000, -0.000000000000000000, 1.000000000000000000 ) ) ;
#47077=ORIENTED_EDGE ( 'NONE', *, *, #32550, .T. ) ;
#47079=ORIENTED_EDGE ( 'NONE', *, *, #86226, .T. ) ;
#47091=DIRECTION ( 'NONE',  ( -0.9981117208278914577, 0.06142469166373826922, 0.000000000000000000 ) ) ;
#47092=ORIENTED_EDGE ( 'NONE', *, *, #36134, .T. ) ;
#47099=EDGE_CURVE ( 'NONE', #526, #43182, #62315, .T. ) ;
#47112=VECTOR ( 'NONE', #56764, 1000.000000000000114 ) ;
#47116=ORIENTED_EDGE ( 'NONE', *, *, #19412, .T. ) ;
#47130=CARTESIAN_POINT ( 'NONE',  ( 37.34220537994156786, 54.61056725541210710, -10.00000000000000000 ) ) ;
#47137=CARTESIAN_POINT ( 'NONE',  ( -11.23413608767113026, 23.57316747377392119, -10.00000000000000000 ) ) ;
#47148=CARTESIAN_POINT ( 'NONE',  ( 48.16808589598787904, 104.3116767361652535, 10.00000000000000000 ) ) ;
#47151=VERTEX_POINT ( 'NONE', #57900 ) ;
#47157=ORIENTED_EDGE ( 'NONE', *, *, #72763, .T. ) ;
#47158=ORIENTED_EDGE ( 'NONE', *, *, #55194, .T. ) ;
#47179=VERTEX_POINT ( 'NONE', #14784 ) ;
#47181=DIRECTION ( 'NONE',  ( -0.6625377181876236365, -0.7490285521785781109, 0.000000000000000000 ) ) ;
#47186=AXIS2_PLACEMENT_3D ( 'NONE', #89333, #58355, #19886 ) ;
#47192=LINE ( 'NONE', #52788, #65707 ) ;
#47205=EDGE_CURVE ( 'NONE', #51689, #57017, #69481, .T. ) ;
#47208=CARTESIAN_POINT ( 'NONE',  ( -19.77026489254404495, 92.98508590942948615, 59.99999999999999289 ) ) ;
#47220=EDGE_CURVE ( 'NONE', #14650, #62301, #59880, .T. ) ;
#47223=CARTESIAN_POINT ( 'NONE',  ( 45.11483101423404918, 69.99284853207299761, -10.00000000000000000 ) ) ;
#47225=VECTOR ( 'NONE', #47273, 1000.000000000000000 ) ;
#47228=CARTESIAN_POINT ( 'NONE',  ( 38.90713690219553200, 54.71539658304151743, 177.5919119679930134 ) ) ;
#47229=EDGE_CURVE ( 'NONE', #54866, #82108, #36445, .T. ) ;
#47231=EDGE_CURVE ( 'NONE', #57637, #71229, #29490, .T. ) ;
#47239=CARTESIAN_POINT ( 'NONE',  ( -15.10528209597770299, 24.46087392797018722, 10.00000000000000000 ) ) ;
#47246=DIRECTION ( 'NONE',  ( 0.7280311630581364213, 0.6855440362341556071, 0.000000000000000000 ) ) ;
#47254=VERTEX_POINT ( 'NONE', #53763 ) ;
#47256=PLANE ( 'NONE',  #19923 ) ;
#47267=CARTESIAN_POINT ( 'NONE',  ( 37.34220537994157496, 54.61056725541210710, -10.00000000000000000 ) ) ;
#47273=DIRECTION ( 'NONE',  ( 0.06415622980647768536, -0.9979398670145503969, 0.000000000000000000 ) ) ;
#47275=LINE ( 'NONE', #55362, #47366 ) ;
#47280=ORIENTED_EDGE ( 'NONE', *, *, #43884, .T. ) ;
#47286=ORIENTED_EDGE ( 'NONE', *, *, #50252, .F. ) ;
#47293=ORIENTED_EDGE ( 'NONE', *, *, #43183, .F. ) ;
#47298=VERTEX_POINT ( 'NONE', #31969 ) ;
#47301=EDGE_CURVE ( 'NONE', #94538, #43912, #94323, .T. ) ;
#47302=ORIENTED_EDGE ( 'NONE', *, *, #89569, .T. ) ;
#47306=ORIENTED_EDGE ( 'NONE', *, *, #76722, .T. ) ;
#47314=AXIS2_PLACEMENT_3D ( 'NONE', #16926, #48852, #79288 ) ;
#47317=DIRECTION ( 'NONE',  ( -0.9413434404457832194, 0.3374500364938435859, 0.000000000000000000 ) ) ;
#47318=FACE_OUTER_BOUND ( 'NONE', #66547, .T. ) ;
#47322=EDGE_CURVE ( 'NONE', #39676, #98547, #85750, .T. ) ;
#47329=ORIENTED_EDGE ( 'NONE', *, *, #72071, .F. ) ;
#47331=EDGE_CURVE ( 'NONE', #48909, #32826, #78601, .T. ) ;
#47338=PLANE ( 'NONE',  #66432 ) ;
#47346=ORIENTED_EDGE ( 'NONE', *, *, #88798, .T. ) ;
#47347=ADVANCED_FACE ( 'NONE', ( #29871 ), #83111, .F. ) ;
#47351=CARTESIAN_POINT ( 'NONE',  ( 47.78135487164287554, 106.4364430393875267, -10.00000000000000000 ) ) ;
#47361=CARTESIAN_POINT ( 'NONE',  ( -25.89332989531674301, 24.59406508915897760, -10.00000000000000000 ) ) ;
#47366=VECTOR ( 'NONE', #16878, 1000.000000000000000 ) ;
#47372=DIRECTION ( 'NONE',  ( 1.000000000000000000, 0.000000000000000000, 0.000000000000000000 ) ) ;
#47389=DIRECTION ( 'NONE',  ( -0.9820299053580079374, -0.1887253692075927247, 0.000000000000000000 ) ) ;
#47394=VERTEX_POINT ( 'NONE', #7064 ) ;
#47403=EDGE_LOOP ( 'NONE', ( #89697, #26136, #24628, #31443 ) ) ;
#47412=DIRECTION ( 'NONE',  ( 0.9140770918436947889, 0.4055404667435467680, 0.000000000000000000 ) ) ;
#47413=FACE_OUTER_BOUND ( 'NONE', #12634, .T. ) ;
#47415=DIRECTION ( 'NONE',  ( -0.000000000000000000, -0.000000000000000000, -1.000000000000000000 ) ) ;
#47420=EDGE_CURVE ( 'NONE', #47179, #71872, #83612, .T. ) ;
#47438=VERTEX_POINT ( 'NONE', #68365 ) ;
#47441=DIRECTION ( 'NONE',  ( -0.5435407515102095299, 0.8393827800519358950, 0.000000000000000000 ) ) ;
#47445=DIRECTION ( 'NONE',  ( 1.000000000000000000, 0.000000000000000000, 0.000000000000000000 ) ) ;
#47454=CIRCLE ( 'NONE', #49128, 70.00000000000001421 ) ;
#47457=VECTOR ( 'NONE', #45424, 1000.000000000000000 ) ;
#47458=ADVANCED_FACE ( 'NONE', ( #91706 ), #22776, .F. ) ;
#47466=ORIENTED_EDGE ( 'NONE', *, *, #84316, .T. ) ;
#47482=CYLINDRICAL_SURFACE ( 'NONE', #86844, 70.00000000000002842 ) ;
#47493=LINE ( 'NONE', #70809, #44678 ) ;
#47494=ADVANCED_FACE ( 'NONE', ( #5085 ), #53172, .F. ) ;
#47516=AXIS2_PLACEMENT_3D ( 'NONE', #82621, #13184, #53155 ) ;
#47523=ORIENTED_EDGE ( 'NONE', *, *, #6392, .F. ) ;
#47540=EDGE_CURVE ( 'NONE', #81228, #60097, #24273, .T. ) ;
#47555=ORIENTED_EDGE ( 'NONE', *, *, #41313, .F. ) ;
#47557=LINE ( 'NONE', #9587, #77089 ) ;
#47564=FACE_OUTER_BOUND ( 'NONE', #92537, .T. ) ;
#47565=DIRECTION ( 'NONE',  ( -1.000000000000000000, 0.000000000000000000, 0.000000000000000000 ) ) ;
#47579=FACE_OUTER_BOUND ( 'NONE', #1926, .T. ) ;
#47581=ORIENTED_EDGE ( 'NONE', *, *, #15768, .T. ) ;
#47596=CARTESIAN_POINT ( 'NONE',  ( 46.43574122514302616, 74.10519008736565638, -10.00000000000000000 ) ) ;
#47616=DIRECTION ( 'NONE',  ( 0.1162373735601425762, 0.9932214622066117826, 0.000000000000000000 ) ) ;
#47636=LINE ( 'NONE', #45632, #97877 ) ;
#47637=LINE ( 'NONE', #93283, #92495 ) ;
#47642=ORIENTED_EDGE ( 'NONE', *, *, #63312, .F. ) ;
#47658=LINE ( 'NONE', #87750, #95232 ) ;
#47659=EDGE_CURVE ( 'NONE', #49332, #52913, #6334, .T. ) ;
#47668=DIRECTION ( 'NONE',  ( 1.000000000000000000, 0.000000000000000000, 0.000000000000000000 ) ) ;
#47670=VERTEX_POINT ( 'NONE', #17657 ) ;
#47680=CARTESIAN_POINT ( 'NONE',  ( 48.32408078245681793, 82.80331927372955647, -10.00000000000000000 ) ) ;
#47682=VERTEX_POINT ( 'NONE', #11068 ) ;
#47689=VECTOR ( 'NONE', #74949, 1000.000000000000000 ) ;
#47702=VERTEX_POINT ( 'NONE', #18155 ) ;
#47704=CARTESIAN_POINT ( 'NONE',  ( 19.18375657693640335, 36.32959363016014720, 10.00000000000000000 ) ) ;
#47711=LINE ( 'NONE', #9232, #30411 ) ;
#47721=VECTOR ( 'NONE', #54377, 1000.000000000000114 ) ;
#47722=EDGE_CURVE ( 'NONE', #45441, #95521, #56126, .T. ) ;
#47735=CARTESIAN_POINT ( 'NONE',  ( -1.712471552152344811, 43.16833485791677560, 59.99999999999999289 ) ) ;
#47739=LINE ( 'NONE', #24948, #99096 ) ;
#47742=VERTEX_POINT ( 'NONE', #49054 ) ;
#47750=FACE_OUTER_BOUND ( 'NONE', #2706, .T. ) ;
#47753=CARTESIAN_POINT ( 'NONE',  ( -20.65464553008482795, 23.07220643578491348, 10.00000000000000000 ) ) ;
#47761=VECTOR ( 'NONE', #24306, 1000.000000000000114 ) ;
#47765=DIRECTION ( 'NONE',  ( 0.8599083858334037878, -0.5104483989331242144, 0.000000000000000000 ) ) ;
#47768=CARTESIAN_POINT ( 'NONE',  ( 15.77038241084232517, 34.14663330942826747, -10.00000000000000000 ) ) ;
#47772=CARTESIAN_POINT ( 'NONE',  ( 48.61286661847091040, 84.94359857078811160, 10.00000000000000000 ) ) ;
#47774=EDGE_LOOP ( 'NONE', ( #5907, #73676, #3706, #7669 ) ) ;
#47777=DIRECTION ( 'NONE',  ( 0.000000000000000000, 0.000000000000000000, 1.000000000000000000 ) ) ;
#47778=EDGE_LOOP ( 'NONE', ( #73882, #85603, #7289, #68193 ) ) ;
#47779=DIRECTION ( 'NONE',  ( -1.000000000000000000, 0.000000000000000000, 0.000000000000000000 ) ) ;
#47783=CARTESIAN_POINT ( 'NONE',  ( 3.722289961109204626, 27.08330320443190331, 10.00000000000000000 ) ) ;
#47784=ORIENTED_EDGE ( 'NONE', *, *, #34499, .F. ) ;
#47789=ORIENTED_EDGE ( 'NONE', *, *, #33747, .T. ) ;
#47791=ORIENTED_EDGE ( 'NONE', *, *, #42677, .T. ) ;
#47794=VECTOR ( 'NONE', #8117, 1000.000000000000000 ) ;
#47804=CARTESIAN_POINT ( 'NONE',  ( -64.74139798177010618, 41.16849083240310847, -10.00000000000000000 ) ) ;
#47817=ORIENTED_EDGE ( 'NONE', *, *, #97395, .T. ) ;
#47829=EDGE_CURVE ( 'NONE', #4560, #5926, #70511, .T. ) ;
#47834=EDGE_CURVE ( 'NONE', #98025, #87101, #35338, .T. ) ;
#47837=LINE ( 'NONE', #47351, #73787 ) ;
#47843=ORIENTED_EDGE ( 'NONE', *, *, #25564, .T. ) ;
#47851=CIRCLE ( 'NONE', #28486, 0.1418229129681557177 ) ;
#47852=CIRCLE ( 'NONE', #21986, 70.00000000000001421 ) ;
#47860=EDGE_LOOP ( 'NONE', ( #10968, #53445, #96163, #79611 ) ) ;
#47863=FACE_OUTER_BOUND ( 'NONE', #91826, .T. ) ;
#47868=CARTESIAN_POINT ( 'NONE',  ( 0.4893710859096792598, 78.77562236714182120, 59.97499999999998721 ) ) ;
#47870=CARTESIAN_POINT ( 'NONE',  ( -19.69202633138669967, 92.92865703790650400, 59.99999999999999289 ) ) ;
#47878=CARTESIAN_POINT ( 'NONE',  ( 15.54467260552930341, 34.00295985972733348, 10.00000000000000000 ) ) ;
#47882=VERTEX_POINT ( 'NONE', #93050 ) ;
#47887=EDGE_CURVE ( 'NONE', #12886, #7039, #30014, .T. ) ;
#47903=AXIS2_PLACEMENT_3D ( 'NONE', #20532, #81857, #50907 ) ;
#47908=ORIENTED_EDGE ( 'NONE', *, *, #12722, .T. ) ;
#47911=VECTOR ( 'NONE', #20054, 1000.000000000000114 ) ;
#47912=ORIENTED_EDGE ( 'NONE', *, *, #82703, .F. ) ;
#47939=CARTESIAN_POINT ( 'NONE',  ( -19.65312891409030271, 93.06504152958497400, -10.00000000000000888 ) ) ;
#47947=ORIENTED_EDGE ( 'NONE', *, *, #1027, .T. ) ;
#47948=DIRECTION ( 'NONE',  ( 0.000000000000000000, -0.000000000000000000, 1.000000000000000000 ) ) ;
#47957=EDGE_LOOP ( 'NONE', ( #8932, #1487, #13971, #18952 ) ) ;
#47976=LINE ( 'NONE', #31284, #65927 ) ;
#47977=VECTOR ( 'NONE', #28751, 1000.000000000000227 ) ;
#47982=EDGE_CURVE ( 'NONE', #89109, #88625, #6442, .T. ) ;
#47988=EDGE_CURVE ( 'NONE', #49571, #81157, #38093, .T. ) ;
#47997=CARTESIAN_POINT ( 'NONE',  ( 44.18794977381974576, 118.5901545549086791, -10.00000000000000000 ) ) ;
#48001=AXIS2_PLACEMENT_3D ( 'NONE', #97602, #49982, #11506 ) ;
#48011=CARTESIAN_POINT ( 'NONE',  ( -67.83107014231842413, 42.28230845022618922, 10.00000000000000000 ) ) ;
#48013=CIRCLE ( 'NONE', #22136, 70.00000000000001421 ) ;
#48014=DIRECTION ( 'NONE',  ( -0.7715546603183375263, -0.6361630342459823062, 0.000000000000000000 ) ) ;
#48022=ORIENTED_EDGE ( 'NONE', *, *, #92557, .F. ) ;
#48026=VERTEX_POINT ( 'NONE', #94067 ) ;
#48027=CARTESIAN_POINT ( 'NONE',  ( 50.30020549591841927, 90.50945844122861672, -10.00000000000000000 ) ) ;
#48028=EDGE_CURVE ( 'NONE', #40468, #39976, #24618, .T. ) ;
#48034=EDGE_LOOP ( 'NONE', ( #18496, #7180, #79371, #54784 ) ) ;
#48042=CARTESIAN_POINT ( 'NONE',  ( -32.30932376655839988, 25.48519649537502119, -10.00000000000000000 ) ) ;
#48043=ORIENTED_EDGE ( 'NONE', *, *, #75358, .T. ) ;
#48044=ORIENTED_EDGE ( 'NONE', *, *, #3015, .F. ) ;
#48056=ORIENTED_EDGE ( 'NONE', *, *, #34182, .T. ) ;
#48059=CIRCLE ( 'NONE', #4385, 70.00000000000001421 ) ;
#48065=DIRECTION ( 'NONE',  ( -1.000000000000000000, 0.000000000000000000, 0.000000000000000000 ) ) ;
#48076=ORIENTED_EDGE ( 'NONE', *, *, #81302, .F. ) ;
#48082=EDGE_LOOP ( 'NONE', ( #83349, #8406, #6432, #87597 ) ) ;
#48083=AXIS2_PLACEMENT_3D ( 'NONE', #93738, #9096, #7090 ) ;
#48102=EDGE_CURVE ( 'NONE', #5362, #28497, #62702, .T. ) ;
#48109=DIRECTION ( 'NONE',  ( -0.000000000000000000, -0.000000000000000000, -1.000000000000000000 ) ) ;
#48115=EDGE_CURVE ( 'NONE', #77592, #91230, #25214, .T. ) ;
#48127=DIRECTION ( 'NONE',  ( -0.8660254037844369313, -0.5000000000000029976, 0.000000000000000000 ) ) ;
#48134=PLANE ( 'NONE',  #67878 ) ;
#48135=AXIS2_PLACEMENT_3D ( 'NONE', #84778, #29546, #144 ) ;
#48138=DIRECTION ( 'NONE',  ( 1.000000000000000000, 0.000000000000000000, 0.000000000000000000 ) ) ;
#48145=FACE_OUTER_BOUND ( 'NONE', #14549, .T. ) ;
#48146=VERTEX_POINT ( 'NONE', #21563 ) ;
#48155=EDGE_LOOP ( 'NONE', ( #67861, #17065, #99149, #43197 ) ) ;
#48156=VECTOR ( 'NONE', #76833, 1000.000000000000227 ) ;
#48161=EDGE_CURVE ( 'NONE', #29721, #70849, #60531, .T. ) ;
#48166=LINE ( 'NONE', #79107, #50107 ) ;
#48168=ORIENTED_EDGE ( 'NONE', *, *, #3849, .F. ) ;
#48193=ORIENTED_EDGE ( 'NONE', *, *, #66082, .F. ) ;
#48194=DIRECTION ( 'NONE',  ( 0.06115825522547522347, -0.9981280818701454560, -0.000000000000000000 ) ) ;
#48197=VECTOR ( 'NONE', #97503, 1000.000000000000000 ) ;
#48206=AXIS2_PLACEMENT_3D ( 'NONE', #26786, #17176, #57168 ) ;
#48211=DIRECTION ( 'NONE',  ( 0.000000000000000000, 0.000000000000000000, 1.000000000000000000 ) ) ;
#48212=VECTOR ( 'NONE', #44803, 1000.000000000000000 ) ;
#48222=VECTOR ( 'NONE', #100101, 999.9999999999998863 ) ;
#48228=AXIS2_PLACEMENT_3D ( 'NONE', #9309, #40183, #71123 ) ;
#48236=ADVANCED_FACE ( 'NONE', ( #79796 ), #70127, .F. ) ;
#48256=PLANE ( 'NONE',  #59006 ) ;
#48260=CARTESIAN_POINT ( 'NONE',  ( -52.01928280585847375, 85.51831290684647513, -10.00000000000000000 ) ) ;
#48262=EDGE_LOOP ( 'NONE', ( #48790, #93328, #18202, #96936 ) ) ;
#48272=CYLINDRICAL_SURFACE ( 'NONE', #53241, 70.00000000000002842 ) ;
#48275=DIRECTION ( 'NONE',  ( -0.7082622432767082810, -0.7059494278973847958, 0.000000000000000000 ) ) ;
#48279=VERTEX_POINT ( 'NONE', #20455 ) ;
#48283=AXIS2_PLACEMENT_3D ( 'NONE', #26934, #43612, #96872 ) ;
#48287=DIRECTION ( 'NONE',  ( -1.000000000000000000, 0.000000000000000000, 0.000000000000000000 ) ) ;
#48288=VECTOR ( 'NONE', #59373, 1000.000000000000000 ) ;
#48289=PLANE ( 'NONE',  #63162 ) ;
#48298=VECTOR ( 'NONE', #53290, 1000.000000000000000 ) ;
#48303=LINE ( 'NONE', #40681, #9541 ) ;
#48304=CARTESIAN_POINT ( 'NONE',  ( -70.89022602266994966, 47.22876919346843749, -10.00000000000000000 ) ) ;
#48317=DIRECTION ( 'NONE',  ( -0.1577859398657163181, 0.9874733399847778204, 0.000000000000000000 ) ) ;
#48319=ORIENTED_EDGE ( 'NONE', *, *, #3280, .T. ) ;
#48322=CARTESIAN_POINT ( 'NONE',  ( 35.52150138090271980, 110.7651959890790039, 59.99999999999999289 ) ) ;
#48326=ADVANCED_FACE ( 'NONE', ( #22917 ), #76161, .T. ) ;
#48328=LINE ( 'NONE', #40199, #45086 ) ;
#48329=CARTESIAN_POINT ( 'NONE',  ( 11.72935026791635416, 51.93958514983272323, 59.99999999999999289 ) ) ;
#48330=ORIENTED_EDGE ( 'NONE', *, *, #51647, .T. ) ;
#48333=VECTOR ( 'NONE', #75797, 1000.000000000000227 ) ;
#48335=DIRECTION ( 'NONE',  ( -0.7911563084720434347, -0.6116140086401625764, 0.000000000000000000 ) ) ;
#48337=EDGE_LOOP ( 'NONE', ( #73896, #51139, #72639, #8691 ) ) ;
#48338=ORIENTED_EDGE ( 'NONE', *, *, #46993, .F. ) ;
#48340=PLANE ( 'NONE',  #12528 ) ;
#48342=DIRECTION ( 'NONE',  ( 1.000000000000000000, 0.000000000000000000, 0.000000000000000000 ) ) ;
#48354=VECTOR ( 'NONE', #5273, 1000.000000000000227 ) ;
#48357=AXIS2_PLACEMENT_3D ( 'NONE', #32362, #49556, #33362 ) ;
#48362=VECTOR ( 'NONE', #64749, 1000.000000000000114 ) ;
#48364=ORIENTED_EDGE ( 'NONE', *, *, #30122, .T. ) ;
#48374=DIRECTION ( 'NONE',  ( -1.000000000000000000, 0.000000000000000000, 0.000000000000000000 ) ) ;
#48375=VERTEX_POINT ( 'NONE', #14335 ) ;
#48377=EDGE_CURVE ( 'NONE', #5980, #26753, #83774, .T. ) ;
#48396=DIRECTION ( 'NONE',  ( 0.000000000000000000, 0.000000000000000000, 1.000000000000000000 ) ) ;
#48402=DIRECTION ( 'NONE',  ( 0.000000000000000000, 0.000000000000000000, 1.000000000000000000 ) ) ;
#48404=CARTESIAN_POINT ( 'NONE',  ( 49.06003799288187395, 95.45573527953635562, -10.00000000000000000 ) ) ;
#48409=CARTESIAN_POINT ( 'NONE',  ( -11.87431992379006651, 23.49859753039504540, 177.5919119679930134 ) ) ;
#48419=DIRECTION ( 'NONE',  ( 0.000000000000000000, 0.000000000000000000, 1.000000000000000000 ) ) ;
#48426=VECTOR ( 'NONE', #76282, 999.9999999999998863 ) ;
#48430=EDGE_LOOP ( 'NONE', ( #40454, #83505, #22016, #69839 ) ) ;
#48450=ORIENTED_EDGE ( 'NONE', *, *, #49270, .T. ) ;
#48465=EDGE_CURVE ( 'NONE', #94679, #78204, #70014, .T. ) ;
#48481=VERTEX_POINT ( 'NONE', #62405 ) ;
#48485=LINE ( 'NONE', #86045, #60937 ) ;
#48491=CARTESIAN_POINT ( 'NONE',  ( 19.39999966495784989, 36.48715600906564305, 10.00000000000000000 ) ) ;
#48500=EDGE_CURVE ( 'NONE', #95263, #24773, #11739, .T. ) ;
#48501=AXIS2_PLACEMENT_3D ( 'NONE', #80064, #64322, #49615 ) ;
#48510=CARTESIAN_POINT ( 'NONE',  ( -19.65312891409030271, 93.06504152958497400, -10.00000000000000888 ) ) ;
#48518=CYLINDRICAL_SURFACE ( 'NONE', #69261, 70.00000000000002842 ) ;
#48527=EDGE_LOOP ( 'NONE', ( #63980, #15669, #82737, #23238 ) ) ;
#48532=CARTESIAN_POINT ( 'NONE',  ( 3.722289961109204626, 27.08330320443190331, -10.00000000000000000 ) ) ;
#48556=CARTESIAN_POINT ( 'NONE',  ( -19.65312891409030271, 93.06504152958497400, 59.99999999999999289 ) ) ;
#48568=EDGE_CURVE ( 'NONE', #83607, #5345, #56189, .T. ) ;
#48573=ORIENTED_EDGE ( 'NONE', *, *, #45048, .T. ) ;
#48575=CARTESIAN_POINT ( 'NONE',  ( -12.95261720355844126, 24.63757726406876714, -10.00000000000000000 ) ) ;
#48579=VERTEX_POINT ( 'NONE', #47596 ) ;
#48581=ADVANCED_FACE ( 'NONE', ( #509 ), #31397, .F. ) ;
#48588=ORIENTED_EDGE ( 'NONE', *, *, #14495, .F. ) ;
#48589=VECTOR ( 'NONE', #47091, 1000.000000000000114 ) ;
#48601=VERTEX_POINT ( 'NONE', #50105 ) ;
#48604=EDGE_CURVE ( 'NONE', #76243, #23143, #7376, .T. ) ;
#48606=CARTESIAN_POINT ( 'NONE',  ( -28.04097607764120781, 24.82386083235215679, -10.00000000000000000 ) ) ;
#48609=LINE ( 'NONE', #41481, #11438 ) ;
#48618=CARTESIAN_POINT ( 'NONE',  ( -4.429217378738782962, 26.01694505731172313, 10.00000000000000000 ) ) ;
#48620=DIRECTION ( 'NONE',  ( -1.000000000000000000, 0.000000000000000000, 0.000000000000000000 ) ) ;
#48621=EDGE_CURVE ( 'NONE', #36836, #17411, #15462, .T. ) ;
#48630=DIRECTION ( 'NONE',  ( 0.3301025504114431519, 0.9439450758449140499, 0.000000000000000000 ) ) ;
#48632=CARTESIAN_POINT ( 'NONE',  ( 50.40832357593285451, 87.79023373031367328, 10.00000000000000000 ) ) ;
#48636=FACE_OUTER_BOUND ( 'NONE', #46796, .T. ) ;
#48639=CARTESIAN_POINT ( 'NONE',  ( -19.65312891409030271, 93.06504152958497400, 59.99999999999999289 ) ) ;
#48650=DIRECTION ( 'NONE',  ( -0.8450603975019799208, 0.5346708562974007428, 0.000000000000000000 ) ) ;
#48651=PLANE ( 'NONE',  #40372 ) ;
#48653=VECTOR ( 'NONE', #10302, 1000.000000000000000 ) ;
#48661=DIRECTION ( 'NONE',  ( -0.9820299053580079374, -0.1887253692075927247, 0.000000000000000000 ) ) ;
#48663=ORIENTED_EDGE ( 'NONE', *, *, #73450, .T. ) ;
#48668=DIRECTION ( 'NONE',  ( -0.3986482622784180974, -0.9171038997749370036, 0.000000000000000000 ) ) ;
#48672=DIRECTION ( 'NONE',  ( -0.8660254037844378194, -0.5000000000000013323, -0.000000000000000000 ) ) ;
#48683=ORIENTED_EDGE ( 'NONE', *, *, #1707, .F. ) ;
#48686=DIRECTION ( 'NONE',  ( -0.9922852870422786964, 0.1239754375649568807, 0.000000000000000000 ) ) ;
#48708=EDGE_CURVE ( 'NONE', #22737, #61085, #19725, .T. ) ;
#48728=ORIENTED_EDGE ( 'NONE', *, *, #16187, .F. ) ;
#48736=VERTEX_POINT ( 'NONE', #48618 ) ;
#48738=EDGE_CURVE ( 'NONE', #61424, #37421, #89178, .T. ) ;
#48757=PLANE ( 'NONE',  #28900 ) ;
#48765=CARTESIAN_POINT ( 'NONE',  ( 44.73065482718367747, 120.5373619841236774, -10.00000000000000000 ) ) ;
#48771=CARTESIAN_POINT ( 'NONE',  ( -4.429217378738782962, 26.01694505731172313, -10.00000000000000000 ) ) ;
#48774=CARTESIAN_POINT ( 'NONE',  ( -19.65312891409030271, 93.06504152958497400, 177.5919119679930134 ) ) ;
#48782=LINE ( 'NONE', #10780, #94566 ) ;
#48783=CARTESIAN_POINT ( 'NONE',  ( 47.54560441532652959, 78.55524412553474178, -10.00000000000000000 ) ) ;
#48789=CARTESIAN_POINT ( 'NONE',  ( -22.20871200244593169, 23.11170711957623070, 177.5919119679930134 ) ) ;
#48790=ORIENTED_EDGE ( 'NONE', *, *, #45472, .F. ) ;
#48796=CYLINDRICAL_SURFACE ( 'NONE', #23051, 70.00000000000002842 ) ;
#48804=VECTOR ( 'NONE', #87978, 1000.000000000000000 ) ;
#48807=ORIENTED_EDGE ( 'NONE', *, *, #71091, .T. ) ;
#48810=VERTEX_POINT ( 'NONE', #15438 ) ;
#48813=ORIENTED_EDGE ( 'NONE', *, *, #95752, .F. ) ;
#48817=CARTESIAN_POINT ( 'NONE',  ( -23.73952538801239598, 24.43184193311135743, -10.00000000000000000 ) ) ;
#48823=ORIENTED_EDGE ( 'NONE', *, *, #52628, .T. ) ;
#48828=ORIENTED_EDGE ( 'NONE', *, *, #76516, .F. ) ;
#48834=EDGE_CURVE ( 'NONE', #54113, #79361, #47837, .T. ) ;
#48839=CARTESIAN_POINT ( 'NONE',  ( -42.72532191160158987, 28.29708160126036987, 10.00000000000000000 ) ) ;
#48846=DIRECTION ( 'NONE',  ( 0.000000000000000000, 0.000000000000000000, 1.000000000000000000 ) ) ;
#48849=VERTEX_POINT ( 'NONE', #2282 ) ;
#48852=DIRECTION ( 'NONE',  ( -0.9956898167541080591, 0.09274582908234035861, 0.000000000000000000 ) ) ;
#48857=LINE ( 'NONE', #56435, #36488 ) ;
#48859=EDGE_CURVE ( 'NONE', #32616, #73603, #40240, .T. ) ;
#48879=ORIENTED_EDGE ( 'NONE', *, *, #20933, .F. ) ;
#48888=LINE ( 'NONE', #64587, #34588 ) ;
#48897=DIRECTION ( 'NONE',  ( 0.5607300124661794838, -0.8279987035736700030, 0.000000000000000000 ) ) ;
#48909=VERTEX_POINT ( 'NONE', #41244 ) ;
#48911=AXIS2_PLACEMENT_3D ( 'NONE', #35577, #58366, #20897 ) ;
#48919=ORIENTED_EDGE ( 'NONE', *, *, #82936, .F. ) ;
#48920=LINE ( 'NONE', #40287, #82822 ) ;
#48927=ORIENTED_EDGE ( 'NONE', *, *, #88252, .T. ) ;
#48937=EDGE_CURVE ( 'NONE', #5335, #709, #24553, .T. ) ;
#48941=EDGE_LOOP ( 'NONE', ( #23357, #22363, #80757, #19937 ) ) ;
#48951=DIRECTION ( 'NONE',  ( -0.6056412518070772855, -0.7957378174433814566, 0.000000000000000000 ) ) ;
#48964=CARTESIAN_POINT ( 'NONE',  ( 48.29091023345864642, 82.53782597618220507, -10.00000000000000000 ) ) ;
#48970=ORIENTED_EDGE ( 'NONE', *, *, #76953, .T. ) ;
#48971=DIRECTION ( 'NONE',  ( 1.000000000000000000, -1.084449990124929494E-13, 0.000000000000000000 ) ) ;
#48974=LINE ( 'NONE', #73278, #11199 ) ;
#48980=AXIS2_PLACEMENT_3D ( 'NONE', #87592, #81448, #88078 ) ;
#48987=FACE_OUTER_BOUND ( 'NONE', #64538, .T. ) ;
#48992=CARTESIAN_POINT ( 'NONE',  ( 45.19716250472275476, 70.24742367233086782, 10.00000000000000000 ) ) ;
#48998=DIRECTION ( 'NONE',  ( -0.000000000000000000, 0.000000000000000000, 1.000000000000000000 ) ) ;
#48999=CIRCLE ( 'NONE', #86208, 70.00000000000001421 ) ;
#49014=ADVANCED_FACE ( 'NONE', ( #13369 ), #19498, .F. ) ;
#49017=DIRECTION ( 'NONE',  ( -0.1032265479692855564, 0.9946578707245747886, 0.000000000000000000 ) ) ;
#49019=CARTESIAN_POINT ( 'NONE',  ( -43.64404709005470551, 40.32064712455566990, 59.99999999999999289 ) ) ;
#49020=DIRECTION ( 'NONE',  ( -0.8615733660689098850, -0.5076330711061763923, 0.000000000000000000 ) ) ;
#49032=CARTESIAN_POINT ( 'NONE',  ( 24.19030146973739193, 38.49624447322263165, 177.5919119679930134 ) ) ;
#49034=DIRECTION ( 'NONE',  ( 0.000000000000000000, 0.000000000000000000, 1.000000000000000000 ) ) ;
#49038=VERTEX_POINT ( 'NONE', #96011 ) ;
#49042=CARTESIAN_POINT ( 'NONE',  ( -64.94778771796556782, 41.33875607593970614, -10.00000000000000000 ) ) ;
#49044=ORIENTED_EDGE ( 'NONE', *, *, #17486, .T. ) ;
#49054=CARTESIAN_POINT ( 'NONE',  ( -23.29562891409031522, 78.77562236714182120, 52.49999999999999289 ) ) ;
#49055=EDGE_CURVE ( 'NONE', #63052, #60481, #99462, .T. ) ;
#49058=LINE ( 'NONE', #79992, #77207 ) ;
#49059=EDGE_LOOP ( 'NONE', ( #51746, #32520, #28844, #3390 ) ) ;
#49069=EDGE_CURVE ( 'NONE', #63771, #2846, #30039, .T. ) ;
#49072=FACE_OUTER_BOUND ( 'NONE', #99676, .T. ) ;
#49077=ORIENTED_EDGE ( 'NONE', *, *, #3947, .T. ) ;
#49079=ORIENTED_EDGE ( 'NONE', *, *, #68382, .T. ) ;
#49082=PLANE ( 'NONE',  #2924 ) ;
#49085=CARTESIAN_POINT ( 'NONE',  ( 50.34596055286379368, 92.70800680107760172, 10.00000000000000000 ) ) ;
#49102=DIRECTION ( 'NONE',  ( 0.000000000000000000, 0.000000000000000000, 1.000000000000000000 ) ) ;
#49109=DIRECTION ( 'NONE',  ( -0.9055221650797476984, -0.4242989612870696758, 0.000000000000000000 ) ) ;
#49113=AXIS2_PLACEMENT_3D ( 'NONE', #43899, #43400, #5909 ) ;
#49125=PLANE ( 'NONE',  #7452 ) ;
#49128=AXIS2_PLACEMENT_3D ( 'NONE', #38670, #54868, #24968 ) ;
#49130=ORIENTED_EDGE ( 'NONE', *, *, #74800, .T. ) ;
#49131=ADVANCED_FACE ( 'NONE', ( #98966 ), #38116, .F. ) ;
#49143=CARTESIAN_POINT ( 'NONE',  ( -19.53599293563658179, 93.14499714974044764, 59.99999999999999289 ) ) ;
#49180=EDGE_CURVE ( 'NONE', #85997, #6688, #69034, .T. ) ;
#49186=LINE ( 'NONE', #41053, #25354 ) ;
#49195=EDGE_LOOP ( 'NONE', ( #69675, #23858, #20539, #73736 ) ) ;
#49206=LINE ( 'NONE', #93842, #83913 ) ;
#49207=DIRECTION ( 'NONE',  ( 0.9997524133706775507, -0.02225111142181396620, 0.000000000000000000 ) ) ;
#49209=AXIS2_PLACEMENT_3D ( 'NONE', #17786, #49663, #95827 ) ;
#49221=DIRECTION ( 'NONE',  ( 0.000000000000000000, 0.000000000000000000, 1.000000000000000000 ) ) ;
#49222=LINE ( 'NONE', #72539, #64414 ) ;
#49232=VERTEX_POINT ( 'NONE', #61430 ) ;
#49237=FACE_OUTER_BOUND ( 'NONE', #35967, .T. ) ;
#49239=CARTESIAN_POINT ( 'NONE',  ( -46.49770490450613636, 29.77544742692501245, -10.00000000000000000 ) ) ;
#49250=EDGE_LOOP ( 'NONE', ( #79477, #44673, #87087, #5338 ) ) ;
#49265=DIRECTION ( 'NONE',  ( 0.000000000000000000, 0.000000000000000000, 1.000000000000000000 ) ) ;
#49270=EDGE_CURVE ( 'NONE', #59009, #47394, #26922, .T. ) ;
#49279=VECTOR ( 'NONE', #80893, 1000.000000000000000 ) ;
#49280=CARTESIAN_POINT ( 'NONE',  ( -2.590881078880516331, 25.17631125121047475, 10.00000000000000000 ) ) ;
#49283=FACE_OUTER_BOUND ( 'NONE', #5475, .T. ) ;
#49288=CARTESIAN_POINT ( 'NONE',  ( -27.77457187288642615, 24.79904599702366852, -10.00000000000000000 ) ) ;
#49300=EDGE_CURVE ( 'NONE', #68396, #34443, #78155, .T. ) ;
#49305=PLANE ( 'NONE',  #62958 ) ;
#49306=VERTEX_POINT ( 'NONE', #62934 ) ;
#49308=EDGE_CURVE ( 'NONE', #28514, #72111, #87322, .T. ) ;
#49314=ORIENTED_EDGE ( 'NONE', *, *, #63793, .F. ) ;
#49315=EDGE_CURVE ( 'NONE', #81256, #34660, #21989, .T. ) ;
#49332=VERTEX_POINT ( 'NONE', #24443 ) ;
#49337=DIRECTION ( 'NONE',  ( -0.2502735827033041316, -0.9681751565707789053, 0.000000000000000000 ) ) ;
#49342=CARTESIAN_POINT ( 'NONE',  ( -35.11898741612374408, 42.34664502445047418, 59.99999999999999289 ) ) ;
#49353=DIRECTION ( 'NONE',  ( -0.5169068966820336009, 0.8560416229147678191, 0.000000000000000000 ) ) ;
#49362=FACE_OUTER_BOUND ( 'NONE', #43548, .T. ) ;
#49379=EDGE_CURVE ( 'NONE', #85319, #52516, #25245, .T. ) ;
#49388=DIRECTION ( 'NONE',  ( -0.000000000000000000, 0.000000000000000000, -1.000000000000000000 ) ) ;
#49389=CARTESIAN_POINT ( 'NONE',  ( 36.76746430747500938, 51.63176190406337440, 10.00000000000000000 ) ) ;
#49393=VERTEX_POINT ( 'NONE', #81184 ) ;
#49400=CARTESIAN_POINT ( 'NONE',  ( -71.61465314115659453, 63.06504152958490295, 45.00000000000001421 ) ) ;
#49404=VECTOR ( 'NONE', #91324, 1000.000000000000000 ) ;
#49417=ORIENTED_EDGE ( 'NONE', *, *, #48859, .T. ) ;
#49424=VERTEX_POINT ( 'NONE', #65433 ) ;
#49428=EDGE_LOOP ( 'NONE', ( #59229, #97342, #69399, #90008, #6487, #52495 ) ) ;
#49429=LINE ( 'NONE', #25125, #49279 ) ;
#49438=CARTESIAN_POINT ( 'NONE',  ( -4.294359489194460089, 63.59252496917286379, -10.00000000000000000 ) ) ;
#49445=AXIS2_PLACEMENT_3D ( 'NONE', #50949, #58061, #42345 ) ;
#49449=CYLINDRICAL_SURFACE ( 'NONE', #36628, 60.00000000000002132 ) ;
#49453=CARTESIAN_POINT ( 'NONE',  ( -36.26652983198114555, 26.35523046909639788, -10.00000000000000000 ) ) ;
#49461=LINE ( 'NONE', #71786, #85638 ) ;
#49467=LINE ( 'NONE', #96119, #20979 ) ;
#49469=DIRECTION ( 'NONE',  ( -0.000000000000000000, -0.000000000000000000, 1.000000000000000000 ) ) ;
#49473=DIRECTION ( 'NONE',  ( -0.1548189829846212950, 0.9879428538673720173, 0.000000000000000000 ) ) ;
#49491=EDGE_CURVE ( 'NONE', #51421, #1235, #91756, .T. ) ;
#49503=DIRECTION ( 'NONE',  ( 0.06115825522547173321, -0.9981280818701455670, 0.000000000000000000 ) ) ;
#49517=AXIS2_PLACEMENT_3D ( 'NONE', #16203, #38988, #22807 ) ;
#49529=CARTESIAN_POINT ( 'NONE',  ( 48.83428215874786815, 87.09189275153327969, 10.00000000000000000 ) ) ;
#49531=ORIENTED_EDGE ( 'NONE', *, *, #10883, .T. ) ;
#49533=EDGE_LOOP ( 'NONE', ( #39478, #94805, #76578, #98569 ) ) ;
#49536=CARTESIAN_POINT ( 'NONE',  ( -2.330697855141256269, 26.52822386297705393, -10.00000000000000000 ) ) ;
#49543=DIRECTION ( 'NONE',  ( -0.9919084036772447543, 0.1269555777209495362, 0.000000000000000000 ) ) ;
#49545=ORIENTED_EDGE ( 'NONE', *, *, #50238, .T. ) ;
#49550=LINE ( 'NONE', #26264, #62605 ) ;
#49552=CARTESIAN_POINT ( 'NONE',  ( 49.06003799288187395, 95.45573527953635562, -10.00000000000000000 ) ) ;
#49556=DIRECTION ( 'NONE',  ( -0.000000000000000000, -0.000000000000000000, 1.000000000000000000 ) ) ;
#49561=CARTESIAN_POINT ( 'NONE',  ( -11.23413608767113026, 23.57316747377392119, 10.00000000000000000 ) ) ;
#49562=ADVANCED_FACE ( 'NONE', ( #24323 ), #54195, .F. ) ;
#49563=VERTEX_POINT ( 'NONE', #39994 ) ;
#49571=VERTEX_POINT ( 'NONE', #32421 ) ;
#49572=ORIENTED_EDGE ( 'NONE', *, *, #37989, .T. ) ;
#49574=ORIENTED_EDGE ( 'NONE', *, *, #65804, .T. ) ;
#49578=CIRCLE ( 'NONE', #88486, 70.00000000000001421 ) ;
#49581=CYLINDRICAL_SURFACE ( 'NONE', #13823, 45.00000000000000000 ) ;
#49583=VECTOR ( 'NONE', #12343, 1000.000000000000114 ) ;
#49586=DIRECTION ( 'NONE',  ( 0.000000000000000000, 0.000000000000000000, 1.000000000000000000 ) ) ;
#49590=AXIS2_PLACEMENT_3D ( 'NONE', #47804, #9329, #40201 ) ;
#49591=CARTESIAN_POINT ( 'NONE',  ( 22.87549206224920084, 39.05096577487528720, -10.00000000000000000 ) ) ;
#49599=DIRECTION ( 'NONE',  ( 1.000000000000000000, 0.000000000000000000, 0.000000000000000000 ) ) ;
#49600=AXIS2_PLACEMENT_3D ( 'NONE', #81806, #89901, #59434 ) ;
#49605=DIRECTION ( 'NONE',  ( -0.1889875038809470387, -0.9819794923402672682, 0.000000000000000000 ) ) ;
#49608=CARTESIAN_POINT ( 'NONE',  ( 43.53831125515428369, 65.97156238185917232, -10.00000000000000000 ) ) ;
#49615=DIRECTION ( 'NONE',  ( -1.000000000000000000, 0.000000000000000000, 0.000000000000000000 ) ) ;
#49630=ADVANCED_FACE ( 'NONE', ( #74441 ), #49125, .F. ) ;
#49635=ORIENTED_EDGE ( 'NONE', *, *, #28639, .T. ) ;
#49636=CARTESIAN_POINT ( 'NONE',  ( -14.79927404260907231, 84.62610232342093752, 15.00661255959723483 ) ) ;
#49646=AXIS2_PLACEMENT_3D ( 'NONE', #9588, #39940, #8575 ) ;
#49657=DIRECTION ( 'NONE',  ( -0.9053220668578555452, -0.4247257412262889220, 0.000000000000000000 ) ) ;
#49658=CARTESIAN_POINT ( 'NONE',  ( 32.61785165683025411, 46.50599740114042646, 177.5919119679930134 ) ) ;
#49660=ORIENTED_EDGE ( 'NONE', *, *, #26528, .F. ) ;
#49661=AXIS2_PLACEMENT_3D ( 'NONE', #1866, #1368, #17557 ) ;
#49663=DIRECTION ( 'NONE',  ( -0.000000000000000000, -0.000000000000000000, -1.000000000000000000 ) ) ;
#49666=ORIENTED_EDGE ( 'NONE', *, *, #93127, .F. ) ;
#49680=FACE_BOUND ( 'NONE', #26041, .T. ) ;
#49690=CIRCLE ( 'NONE', #85388, 70.00000000000001421 ) ;
#49702=DIRECTION ( 'NONE',  ( -0.7751245550734549017, -0.6318084552474576565, 0.000000000000000000 ) ) ;
#49704=VERTEX_POINT ( 'NONE', #69794 ) ;
#49707=VERTEX_POINT ( 'NONE', #32795 ) ;
#49715=ORIENTED_EDGE ( 'NONE', *, *, #12523, .F. ) ;
#49723=CARTESIAN_POINT ( 'NONE',  ( 27.53018959221258655, 41.35687530090521591, -10.00000000000000000 ) ) ;
#49726=VECTOR ( 'NONE', #70418, 1000.000000000000000 ) ;
#49727=AXIS2_PLACEMENT_3D ( 'NONE', #76941, #30851, #61737 ) ;
#49729=ADVANCED_FACE ( 'NONE', ( #23682 ), #31783, .F. ) ;
#49730=EDGE_CURVE ( 'NONE', #92719, #15908, #18830, .T. ) ;
#49742=EDGE_CURVE ( 'NONE', #42808, #76499, #72206, .T. ) ;
#49755=EDGE_CURVE ( 'NONE', #23113, #37415, #38387, .T. ) ;
#49763=CARTESIAN_POINT ( 'NONE',  ( -18.88433730096684116, 34.39435382651002726, 59.99999999999999289 ) ) ;
#49771=CARTESIAN_POINT ( 'NONE',  ( 37.34220537994157496, 54.61056725541210710, -10.00000000000000000 ) ) ;
#49782=ORIENTED_EDGE ( 'NONE', *, *, #93081, .F. ) ;
#49786=EDGE_LOOP ( 'NONE', ( #10098, #75736, #30648, #21861 ) ) ;
#49794=VERTEX_POINT ( 'NONE', #39376 ) ;
#49801=ORIENTED_EDGE ( 'NONE', *, *, #85926, .T. ) ;
#49805=DIRECTION ( 'NONE',  ( -0.000000000000000000, 0.000000000000000000, 1.000000000000000000 ) ) ;
#49809=EDGE_CURVE ( 'NONE', #82431, #69980, #15582, .T. ) ;
#49815=CIRCLE ( 'NONE', #19108, 70.00000000000001421 ) ;
#49824=VECTOR ( 'NONE', #99268, 1000.000000000000000 ) ;
#49835=EDGE_CURVE ( 'NONE', #68611, #51434, #47493, .T. ) ;
#49836=DIRECTION ( 'NONE',  ( -1.000000000000000000, 0.000000000000000000, 0.000000000000000000 ) ) ;
#49840=ORIENTED_EDGE ( 'NONE', *, *, #28666, .F. ) ;
#49841=DIRECTION ( 'NONE',  ( 0.000000000000000000, -0.000000000000000000, 1.000000000000000000 ) ) ;
#49856=CARTESIAN_POINT ( 'NONE',  ( 42.25626477193290498, 60.39660150822810891, -10.00000000000000000 ) ) ;
#49863=AXIS2_PLACEMENT_3D ( 'NONE', #9998, #77902, #24186 ) ;
#49864=ORIENTED_EDGE ( 'NONE', *, *, #55999, .F. ) ;
#49868=CIRCLE ( 'NONE', #11063, 50.00000000000000711 ) ;
#49870=AXIS2_PLACEMENT_3D ( 'NONE', #79264, #9837, #69610 ) ;
#49879=CARTESIAN_POINT ( 'NONE',  ( -5.362061845104283186, 24.53938646500536436, 177.5919119679930134 ) ) ;
#49881=VECTOR ( 'NONE', #41502, 1000.000000000000114 ) ;
#49884=DIRECTION ( 'NONE',  ( -0.9213551052231903071, 0.3887219701524006754, 0.000000000000000000 ) ) ;
#49889=CIRCLE ( 'NONE', #54705, 70.00000000000001421 ) ;
#49890=DIRECTION ( 'NONE',  ( 0.000000000000000000, 0.000000000000000000, 1.000000000000000000 ) ) ;
#49899=VERTEX_POINT ( 'NONE', #58094 ) ;
#49908=VECTOR ( 'NONE', #73543, 1000.000000000000000 ) ;
#49909=ORIENTED_EDGE ( 'NONE', *, *, #58548, .T. ) ;
#49918=EDGE_LOOP ( 'NONE', ( #33166, #87744, #94855, #71388 ) ) ;
#49920=CARTESIAN_POINT ( 'NONE',  ( -19.65312891409030271, 93.06504152958497400, 177.5919119679930134 ) ) ;
#49921=LINE ( 'NONE', #17012, #35075 ) ;
#49922=AXIS2_PLACEMENT_3D ( 'NONE', #14099, #13607, #60169 ) ;
#49923=ORIENTED_EDGE ( 'NONE', *, *, #97779, .T. ) ;
#49924=CARTESIAN_POINT ( 'NONE',  ( -63.08903959183645327, 39.77784189046417396, -10.00000000000000000 ) ) ;
#49935=ORIENTED_EDGE ( 'NONE', *, *, #46143, .T. ) ;
#49940=VECTOR ( 'NONE', #97935, 999.9999999999998863 ) ;
#49949=VECTOR ( 'NONE', #12209, 1000.000000000000000 ) ;
#49951=VECTOR ( 'NONE', #71236, 1000.000000000000114 ) ;
#49953=ORIENTED_EDGE ( 'NONE', *, *, #93081, .T. ) ;
#49965=AXIS2_PLACEMENT_3D ( 'NONE', #68237, #82513, #44438 ) ;
#49966=ORIENTED_EDGE ( 'NONE', *, *, #8219, .F. ) ;
#49977=CIRCLE ( 'NONE', #41869, 45.00000000000000000 ) ;
#49982=DIRECTION ( 'NONE',  ( 0.000000000000000000, 0.000000000000000000, 1.000000000000000000 ) ) ;
#49986=PLANE ( 'NONE',  #91913 ) ;
#49998=EDGE_CURVE ( 'NONE', #1644, #75140, #68985, .T. ) ;
#50009=LINE ( 'NONE', #94648, #53321 ) ;
#50015=DIRECTION ( 'NONE',  ( 0.3693965786901518555, -0.9292718480896806632, 0.000000000000000000 ) ) ;
#50017=ORIENTED_EDGE ( 'NONE', *, *, #59102, .F. ) ;
#50033=ORIENTED_EDGE ( 'NONE', *, *, #74187, .T. ) ;
#50051=ORIENTED_EDGE ( 'NONE', *, *, #54053, .T. ) ;
#50055=CARTESIAN_POINT ( 'NONE',  ( -63.34358462235559273, 38.37368864812747660, -10.00000000000000000 ) ) ;
#50062=CARTESIAN_POINT ( 'NONE',  ( 22.45462004596304695, 37.14601545153949047, -10.00000000000000000 ) ) ;
#50064=ORIENTED_EDGE ( 'NONE', *, *, #60232, .F. ) ;
#50068=EDGE_LOOP ( 'NONE', ( #74101, #84007, #27503, #84947 ) ) ;
#50071=FACE_OUTER_BOUND ( 'NONE', #55909, .T. ) ;
#50077=ORIENTED_EDGE ( 'NONE', *, *, #19912, .T. ) ;
#50079=ADVANCED_FACE ( 'NONE', ( #280 ), #15978, .F. ) ;
#50093=LINE ( 'NONE', #64804, #4765 ) ;
#50094=DIRECTION ( 'NONE',  ( -0.9825427565607363078, 0.1860369090530953895, 0.000000000000000000 ) ) ;
#50095=FACE_OUTER_BOUND ( 'NONE', #48430, .T. ) ;
#50096=PLANE ( 'NONE',  #98564 ) ;
#50097=LINE ( 'NONE', #81053, #14595 ) ;
#50105=CARTESIAN_POINT ( 'NONE',  ( -50.66096862766640641, 31.69950886434491721, 10.00000000000000000 ) ) ;
#50107=VECTOR ( 'NONE', #9690, 1000.000000000000000 ) ;
#50111=AXIS2_PLACEMENT_3D ( 'NONE', #1538, #40502, #84656 ) ;
#50134=CARTESIAN_POINT ( 'NONE',  ( -56.06787742410712383, 34.75406423768147590, -10.00000000000000000 ) ) ;
#50135=DIRECTION ( 'NONE',  ( -0.8218955677251095215, -0.5696381972391070247, 0.000000000000000000 ) ) ;
#50141=EDGE_LOOP ( 'NONE', ( #59375, #92, #97771, #65261, #70489 ) ) ;
#50145=CARTESIAN_POINT ( 'NONE',  ( 45.66470909604093720, 114.5311720768849995, -10.00000000000000000 ) ) ;
#50146=ORIENTED_EDGE ( 'NONE', *, *, #46009, .T. ) ;
#50155=EDGE_LOOP ( 'NONE', ( #13068, #25458, #35142, #76105 ) ) ;
#50157=CARTESIAN_POINT ( 'NONE',  ( -26.59607535340072104, 23.41021043553327630, 10.00000000000000000 ) ) ;
#50165=ORIENTED_EDGE ( 'NONE', *, *, #4979, .F. ) ;
#50166=CIRCLE ( 'NONE', #42061, 50.00000000000000711 ) ;
#50169=CARTESIAN_POINT ( 'NONE',  ( -72.30469571560091424, 48.86078274006646183, 10.00000000000000000 ) ) ;
#50171=ORIENTED_EDGE ( 'NONE', *, *, #64505, .F. ) ;
#50173=DIRECTION ( 'NONE',  ( -0.9805290675673918876, -0.1963739994383708332, 0.000000000000000000 ) ) ;
#50183=FACE_BOUND ( 'NONE', #61654, .T. ) ;
#50192=PLANE ( 'NONE',  #12465 ) ;
#50195=ORIENTED_EDGE ( 'NONE', *, *, #37497, .T. ) ;
#50199=EDGE_CURVE ( 'NONE', #33351, #6194, #85429, .T. ) ;
#50211=FACE_OUTER_BOUND ( 'NONE', #11064, .T. ) ;
#50214=CARTESIAN_POINT ( 'NONE',  ( -27.23710841895085011, 23.47708815495369450, 10.00000000000000000 ) ) ;
#50215=ORIENTED_EDGE ( 'NONE', *, *, #56431, .F. ) ;
#50219=DIRECTION ( 'NONE',  ( -0.7440200784635719877, -0.6681572590663519273, 0.000000000000000000 ) ) ;
#50220=VECTOR ( 'NONE', #38793, 1000.000000000000000 ) ;
#50230=VECTOR ( 'NONE', #45586, 1000.000000000000227 ) ;
#50238=EDGE_CURVE ( 'NONE', #95379, #37787, #23560, .T. ) ;
#50251=DIRECTION ( 'NONE',  ( -1.000000000000000000, 0.000000000000000000, 0.000000000000000000 ) ) ;
#50252=EDGE_CURVE ( 'NONE', #42468, #84728, #23705, .T. ) ;
#50271=ORIENTED_EDGE ( 'NONE', *, *, #87525, .T. ) ;
#50281=EDGE_LOOP ( 'NONE', ( #51291, #69069, #17398, #85950 ) ) ;
#50282=ORIENTED_EDGE ( 'NONE', *, *, #48604, .F. ) ;
#50304=EDGE_LOOP ( 'NONE', ( #27583, #70009, #62767, #71725 ) ) ;
#50305=CARTESIAN_POINT ( 'NONE',  ( -31.49789205211705934, 23.81092751074078606, 10.00000000000000000 ) ) ;
#50306=AXIS2_PLACEMENT_3D ( 'NONE', #31078, #8299, #44780 ) ;
#50307=ORIENTED_EDGE ( 'NONE', *, *, #19310, .T. ) ;
#50315=EDGE_LOOP ( 'NONE', ( #64515, #3728, #94169, #70101 ) ) ;
#50316=CARTESIAN_POINT ( 'NONE',  ( 15.70095469851434622, 53.54748473301773970, 59.99999999999999289 ) ) ;
#50319=LINE ( 'NONE', #11845, #46167 ) ;
#50322=VERTEX_POINT ( 'NONE', #52229 ) ;
#50328=LINE ( 'NONE', #10850, #60242 ) ;
#50333=CARTESIAN_POINT ( 'NONE',  ( 5.404797899793122973, 27.42564005363386315, 10.00000000000000000 ) ) ;
#50344=DIRECTION ( 'NONE',  ( 0.7891516029629116469, -0.6141984594095518668, 0.000000000000000000 ) ) ;
#50358=CARTESIAN_POINT ( 'NONE',  ( 48.92549481379854370, 97.87922363803308201, -10.00000000000000000 ) ) ;
#50367=EDGE_CURVE ( 'NONE', #53634, #52938, #61815, .T. ) ;
#50368=PLANE ( 'NONE',  #31152 ) ;
#50369=CARTESIAN_POINT ( 'NONE',  ( 26.37028381016231648, 40.32183835407519723, 177.5919119679930134 ) ) ;
#50383=FACE_OUTER_BOUND ( 'NONE', #10561, .T. ) ;
#50385=ORIENTED_EDGE ( 'NONE', *, *, #93104, .F. ) ;
#50387=DIRECTION ( 'NONE',  ( 1.000000000000000000, 0.000000000000000000, 0.000000000000000000 ) ) ;
#50394=EDGE_CURVE ( 'NONE', #70646, #16945, #41007, .T. ) ;
#50401=CARTESIAN_POINT ( 'NONE',  ( -38.35373792487678202, 26.90998726756845727, 10.00000000000000000 ) ) ;
#50404=ORIENTED_EDGE ( 'NONE', *, *, #59666, .F. ) ;
#50407=FACE_OUTER_BOUND ( 'NONE', #51957, .T. ) ;
#50410=CARTESIAN_POINT ( 'NONE',  ( -0.8836234265189104597, 25.35879081310345029, 10.00000000000000000 ) ) ;
#50411=LINE ( 'NONE', #82861, #17177 ) ;
#50419=EDGE_LOOP ( 'NONE', ( #42062, #3968, #87739, #45308 ) ) ;
#50426=ORIENTED_EDGE ( 'NONE', *, *, #25713, .T. ) ;
#50427=EDGE_CURVE ( 'NONE', #80286, #91687, #26836, .T. ) ;
#50433=DIRECTION ( 'NONE',  ( 0.000000000000000000, 0.000000000000000000, 1.000000000000000000 ) ) ;
#50437=LINE ( 'NONE', #41329, #98133 ) ;
#50441=DIRECTION ( 'NONE',  ( 1.000000000000000000, 0.000000000000000000, 0.000000000000000000 ) ) ;
#50442=VERTEX_POINT ( 'NONE', #75954 ) ;
#50444=DIRECTION ( 'NONE',  ( -0.000000000000000000, -0.000000000000000000, 1.000000000000000000 ) ) ;
#50446=EDGE_CURVE ( 'NONE', #68986, #95838, #88522, .T. ) ;
#50459=PLANE ( 'NONE',  #20736 ) ;
#50467=PLANE ( 'NONE',  #41571 ) ;
#50469=DIRECTION ( 'NONE',  ( 1.000000000000000000, 0.000000000000000000, 0.000000000000000000 ) ) ;
#50479=VECTOR ( 'NONE', #50911, 1000.000000000000000 ) ;
#50486=VECTOR ( 'NONE', #43126, 1000.000000000000114 ) ;
#50490=CARTESIAN_POINT ( 'NONE',  ( 4.520885125481575173, 45.87218647215556899, 59.99999999999999289 ) ) ;
#50500=ORIENTED_EDGE ( 'NONE', *, *, #12607, .F. ) ;
#50507=VERTEX_POINT ( 'NONE', #76439 ) ;
#50509=LINE ( 'NONE', #33850, #36 ) ;
#50511=CARTESIAN_POINT ( 'NONE',  ( -36.30795748510355736, 64.30503951426791787, -10.00000000000000000 ) ) ;
#50520=ORIENTED_EDGE ( 'NONE', *, *, #11096, .T. ) ;
#50531=CARTESIAN_POINT ( 'NONE',  ( 46.60452734134890562, 70.48356709729735314, -10.00000000000000000 ) ) ;
#50533=VERTEX_POINT ( 'NONE', #99777 ) ;
#50538=CARTESIAN_POINT ( 'NONE',  ( -19.65312891409030271, 93.06504152958497400, 177.5919119679930134 ) ) ;
#50541=DIRECTION ( 'NONE',  ( 0.7061384650677022812, 0.7080737730998298840, 0.000000000000000000 ) ) ;
#50544=DIRECTION ( 'NONE',  ( 0.9291732088853837945, -0.3696446237802449852, 0.000000000000000000 ) ) ;
#50545=LINE ( 'NONE', #12572, #35400 ) ;
#50548=VERTEX_POINT ( 'NONE', #67364 ) ;
#50549=CYLINDRICAL_SURFACE ( 'NONE', #59256, 70.00000000000002842 ) ;
#50552=VECTOR ( 'NONE', #54117, 1000.000000000000000 ) ;
#50555=EDGE_CURVE ( 'NONE', #8241, #20627, #47557, .T. ) ;
#50556=VECTOR ( 'NONE', #87060, 1000.000000000000114 ) ;
#50561=CARTESIAN_POINT ( 'NONE',  ( -56.34825754162683609, 48.22061105236409873, 59.99999999999999289 ) ) ;
#50565=CARTESIAN_POINT ( 'NONE',  ( 48.72058909919672942, 76.89514952714607432, -10.00000000000000000 ) ) ;
#50568=VECTOR ( 'NONE', #14629, 1000.000000000000000 ) ;
#50571=CARTESIAN_POINT ( 'NONE',  ( -44.74834796241764678, 29.05375577536863929, -10.00000000000000000 ) ) ;
#50575=CARTESIAN_POINT ( 'NONE',  ( 34.19524549848080852, 69.75853580221966865, 59.99999999999999289 ) ) ;
#50580=CARTESIAN_POINT ( 'NONE',  ( 11.76667899187106059, 31.90941714274742225, -10.00000000000000000 ) ) ;
#50588=DIRECTION ( 'NONE',  ( -0.000000000000000000, 0.000000000000000000, -1.000000000000000000 ) ) ;
#50614=LINE ( 'NONE', #65814, #466 ) ;
#50619=EDGE_CURVE ( 'NONE', #1972, #11268, #1974, .T. ) ;
#50621=LINE ( 'NONE', #70054, #61329 ) ;
#50629=CARTESIAN_POINT ( 'NONE',  ( -18.11093984425370351, 79.64604002188578136, 14.00762583401780859 ) ) ;
#50633=AXIS2_PLACEMENT_3D ( 'NONE', #88996, #57006, #18535 ) ;
#50652=EDGE_CURVE ( 'NONE', #84728, #56928, #78484, .T. ) ;
#50656=ORIENTED_EDGE ( 'NONE', *, *, #13474, .F. ) ;
#50659=CARTESIAN_POINT ( 'NONE',  ( 45.57373283677819131, 114.7827874512442889, -10.00000000000000000 ) ) ;
#50665=ORIENTED_EDGE ( 'NONE', *, *, #22839, .F. ) ;
#50669=FACE_BOUND ( 'NONE', #9301, .T. ) ;
#50676=EDGE_LOOP ( 'NONE', ( #42441, #47555, #94669, #25108 ) ) ;
#50681=ORIENTED_EDGE ( 'NONE', *, *, #910, .T. ) ;
#50697=VECTOR ( 'NONE', #62206, 999.9999999999998863 ) ;
#50701=CARTESIAN_POINT ( 'NONE',  ( 20.94669640352213236, 37.57748520232516398, -10.00000000000000000 ) ) ;
#50703=DIRECTION ( 'NONE',  ( -0.8098206029990988597, 0.5866775868892349921, 0.000000000000000000 ) ) ;
#50709=AXIS2_PLACEMENT_3D ( 'NONE', #8306, #92926, #7295 ) ;
#50727=EDGE_CURVE ( 'NONE', #89238, #35590, #41963, .T. ) ;
#50746=EDGE_CURVE ( 'NONE', #4283, #47151, #1102, .T. ) ;
#50752=LINE ( 'NONE', #72601, #61139 ) ;
#50756=DIRECTION ( 'NONE',  ( 0.9819794923402652698, -0.1889875038809575303, 0.000000000000000000 ) ) ;
#50761=PLANE ( 'NONE',  #40848 ) ;
#50773=VECTOR ( 'NONE', #65855, 1000.000000000000000 ) ;
#50782=EDGE_LOOP ( 'NONE', ( #94073, #99572, #43954, #34233 ) ) ;
#50785=AXIS2_PLACEMENT_3D ( 'NONE', #49920, #42791, #66115 ) ;
#50799=CYLINDRICAL_SURFACE ( 'NONE', #28226, 70.00000000000002842 ) ;
#50801=CARTESIAN_POINT ( 'NONE',  ( 2.064617007569734319, 27.83817977871672511, -10.00000000000000000 ) ) ;
#50803=PLANE ( 'NONE',  #60598 ) ;
#50805=CARTESIAN_POINT ( 'NONE',  ( 6.117390533544194930, 29.33055864014943026, -10.00000000000000000 ) ) ;
#50809=ORIENTED_EDGE ( 'NONE', *, *, #91483, .F. ) ;
#50816=ORIENTED_EDGE ( 'NONE', *, *, #90683, .F. ) ;
#50817=ORIENTED_EDGE ( 'NONE', *, *, #80093, .F. ) ;
#50820=LINE ( 'NONE', #81769, #49583 ) ;
#50841=CARTESIAN_POINT ( 'NONE',  ( 20.46409116061435185, 58.39290319439324861, 59.99999999999999289 ) ) ;
#50844=DIRECTION ( 'NONE',  ( -0.000000000000000000, 0.000000000000000000, 1.000000000000000000 ) ) ;
#50845=CARTESIAN_POINT ( 'NONE',  ( 25.98835327777827686, 41.64452202306097206, -10.00000000000000000 ) ) ;
#50852=VERTEX_POINT ( 'NONE', #69493 ) ;
#50856=PLANE ( 'NONE',  #49600 ) ;
#50876=EDGE_CURVE ( 'NONE', #88538, #45464, #21299, .T. ) ;
#50881=ORIENTED_EDGE ( 'NONE', *, *, #78956, .T. ) ;
#50884=DIRECTION ( 'NONE',  ( 1.000000000000000000, 0.000000000000000000, -0.000000000000000000 ) ) ;
#50887=VERTEX_POINT ( 'NONE', #19811 ) ;
#50889=CARTESIAN_POINT ( 'NONE',  ( 48.81784752633560487, 86.82484054835779830, 10.00000000000000000 ) ) ;
#50902=DIRECTION ( 'NONE',  ( -0.001635407438350360964, -0.9999986627203610867, 0.000000000000000000 ) ) ;
#50907=DIRECTION ( 'NONE',  ( 1.000000000000000000, 0.000000000000000000, 0.000000000000000000 ) ) ;
#50911=DIRECTION ( 'NONE',  ( -0.000000000000000000, 0.000000000000000000, 1.000000000000000000 ) ) ;
#50916=EDGE_LOOP ( 'NONE', ( #84820, #36464, #40918, #58378 ) ) ;
#50918=CIRCLE ( 'NONE', #63865, 70.00000000000001421 ) ;
#50920=CARTESIAN_POINT ( 'NONE',  ( 49.63464994930630070, 103.0251469596019120, 177.5919119679930134 ) ) ;
#50922=VERTEX_POINT ( 'NONE', #81634 ) ;
#50926=DIRECTION ( 'NONE',  ( 0.8951289669282637140, -0.4458072818673325943, 0.000000000000000000 ) ) ;
#50935=ORIENTED_EDGE ( 'NONE', *, *, #51085, .T. ) ;
#50941=EDGE_CURVE ( 'NONE', #44888, #56418, #94926, .T. ) ;
#50949=CARTESIAN_POINT ( 'NONE',  ( 38.36706665919591330, 84.31990413814679641, 59.99999999999999289 ) ) ;
#50956=CARTESIAN_POINT ( 'NONE',  ( 26.15794687706369004, 39.79426100978996317, -10.00000000000000000 ) ) ;
#50960=CARTESIAN_POINT ( 'NONE',  ( -19.65312891409030271, 93.06504152958497400, -10.00000000000000888 ) ) ;
#50966=EDGE_CURVE ( 'NONE', #24509, #80425, #13694, .T. ) ;
#50970=DIRECTION ( 'NONE',  ( -0.7492053821869066876, -0.6623377501714446947, 0.000000000000000000 ) ) ;
#50982=VECTOR ( 'NONE', #33107, 1000.000000000000000 ) ;
#50984=EDGE_CURVE ( 'NONE', #52516, #76128, #70894, .T. ) ;
#50998=EDGE_LOOP ( 'NONE', ( #89984, #28745, #24049, #60020 ) ) ;
#51000=CARTESIAN_POINT ( 'NONE',  ( -29.91485116994501325, 25.08783183303773967, 10.00000000000000000 ) ) ;
#51003=EDGE_CURVE ( 'NONE', #3615, #8702, #3502, .T. ) ;
#51004=EDGE_CURVE ( 'NONE', #16059, #66385, #57663, .T. ) ;
#51007=DIRECTION ( 'NONE',  ( -0.8560416229147732592, -0.5169068966820244970, 0.000000000000000000 ) ) ;
#51009=CARTESIAN_POINT ( 'NONE',  ( -19.65312891409030271, 93.06504152958497400, 10.00000000000000888 ) ) ;
#51013=VERTEX_POINT ( 'NONE', #96720 ) ;
#51026=AXIS2_PLACEMENT_3D ( 'NONE', #43719, #98947, #30019 ) ;
#51031=VECTOR ( 'NONE', #15286, 1000.000000000000000 ) ;
#51032=EDGE_LOOP ( 'NONE', ( #78816, #52304, #48168, #76488 ) ) ;
#51049=ORIENTED_EDGE ( 'NONE', *, *, #32096, .T. ) ;
#51056=VECTOR ( 'NONE', #31018, 1000.000000000000227 ) ;
#51060=ORIENTED_EDGE ( 'NONE', *, *, #86050, .F. ) ;
#51062=ADVANCED_FACE ( 'NONE', ( #58168 ), #89152, .F. ) ;
#51068=PLANE ( 'NONE',  #13891 ) ;
#51083=LINE ( 'NONE', #59164, #9507 ) ;
#51085=EDGE_CURVE ( 'NONE', #95597, #31449, #22062, .T. ) ;
#51089=CARTESIAN_POINT ( 'NONE',  ( -22.47745507583526958, 59.95093256704510054, -10.00000000000000000 ) ) ;
#51091=CARTESIAN_POINT ( 'NONE',  ( -57.88150100324660485, 35.92665207732902388, -10.00000000000000000 ) ) ;
#51092=LINE ( 'NONE', #64824, #33060 ) ;
#51093=CARTESIAN_POINT ( 'NONE',  ( 50.40832357593285451, 87.79023373031367328, -10.00000000000000000 ) ) ;
#51100=EDGE_CURVE ( 'NONE', #73348, #41972, #26001, .T. ) ;
#51103=DIRECTION ( 'NONE',  ( -0.3074612162317687525, 0.9515606131578174809, 0.000000000000000000 ) ) ;
#51105=CARTESIAN_POINT ( 'NONE',  ( -19.65312891409030271, 93.06504152958497400, -10.00000000000000888 ) ) ;
#51114=VECTOR ( 'NONE', #5486, 1000.000000000000000 ) ;
#51116=LINE ( 'NONE', #80076, #29537 ) ;
#51121=CARTESIAN_POINT ( 'NONE',  ( -4.429217378738782962, 26.01694505731172313, -10.00000000000000000 ) ) ;
#51123=FACE_OUTER_BOUND ( 'NONE', #45277, .T. ) ;
#51131=ORIENTED_EDGE ( 'NONE', *, *, #43638, .F. ) ;
#51139=ORIENTED_EDGE ( 'NONE', *, *, #17486, .F. ) ;
#51143=DIRECTION ( 'NONE',  ( -0.000000000000000000, 0.000000000000000000, -1.000000000000000000 ) ) ;
#51156=CARTESIAN_POINT ( 'NONE',  ( 47.57035326562169075, 72.63383583914733777, -10.00000000000000000 ) ) ;
#51157=CARTESIAN_POINT ( 'NONE',  ( 48.23560136428436351, 110.1272893647940521, 177.5919119679930134 ) ) ;
#51159=EDGE_CURVE ( 'NONE', #43174, #98545, #35578, .T. ) ;
#51164=AXIS2_PLACEMENT_3D ( 'NONE', #243, #16437, #78257 ) ;
#51167=ORIENTED_EDGE ( 'NONE', *, *, #38061, .T. ) ;
#51170=DIRECTION ( 'NONE',  ( 1.000000000000000000, 0.000000000000000000, 0.000000000000000000 ) ) ;
#51173=CARTESIAN_POINT ( 'NONE',  ( 47.46694519036041982, 73.19305994210745325, 177.5919119679930134 ) ) ;
#51184=EDGE_CURVE ( 'NONE', #56966, #17015, #44155, .T. ) ;
#51186=CARTESIAN_POINT ( 'NONE',  ( 1.638219116881074022, 26.38162155862026736, 177.5919119679930134 ) ) ;
#51187=CYLINDRICAL_SURFACE ( 'NONE', #85297, 70.00000000000002842 ) ;
#51189=ORIENTED_EDGE ( 'NONE', *, *, #86793, .F. ) ;
#51194=EDGE_CURVE ( 'NONE', #57311, #57476, #80741, .T. ) ;
#51195=VECTOR ( 'NONE', #19331, 1000.000000000000114 ) ;
#51198=CARTESIAN_POINT ( 'NONE',  ( 40.34888600819125060, 126.6204015641749834, 10.00000000000000000 ) ) ;
#51214=DIRECTION ( 'NONE',  ( 0.000000000000000000, 0.000000000000000000, 1.000000000000000000 ) ) ;
#51237=VECTOR ( 'NONE', #86888, 1000.000000000000114 ) ;
#51252=EDGE_CURVE ( 'NONE', #69843, #90334, #74, .T. ) ;
#51258=ORIENTED_EDGE ( 'NONE', *, *, #97670, .T. ) ;
#51259=AXIS2_PLACEMENT_3D ( 'NONE', #62267, #14201, #60764 ) ;
#51266=VECTOR ( 'NONE', #5182, 1000.000000000000114 ) ;
#51267=CARTESIAN_POINT ( 'NONE',  ( 48.21858077004885246, 104.0489273421469818, 10.00000000000000000 ) ) ;
#51269=ORIENTED_EDGE ( 'NONE', *, *, #75084, .T. ) ;
#51291=ORIENTED_EDGE ( 'NONE', *, *, #71565, .F. ) ;
#51294=DIRECTION ( 'NONE',  ( -0.4813790724697843970, -0.8765125147926470239, 0.000000000000000000 ) ) ;
#51295=DIRECTION ( 'NONE',  ( -0.3984034379159046013, 0.9172102815912979157, 0.000000000000000000 ) ) ;
#51305=LINE ( 'NONE', #18448, #28281 ) ;
#51308=CARTESIAN_POINT ( 'NONE',  ( 49.09245556086620610, 93.56363653685789927, -10.00000000000000000 ) ) ;
#51309=VECTOR ( 'NONE', #13397, 1000.000000000000000 ) ;
#51318=VERTEX_POINT ( 'NONE', #14035 ) ;
#51320=VECTOR ( 'NONE', #78395, 1000.000000000000000 ) ;
#51323=VECTOR ( 'NONE', #37280, 1000.000000000000000 ) ;
#51336=VECTOR ( 'NONE', #54547, 1000.000000000000114 ) ;
#51337=ORIENTED_EDGE ( 'NONE', *, *, #33649, .T. ) ;
#51348=VECTOR ( 'NONE', #18506, 1000.000000000000114 ) ;
#51365=ORIENTED_EDGE ( 'NONE', *, *, #97697, .F. ) ;
#51374=CARTESIAN_POINT ( 'NONE',  ( 33.47037235539275457, 49.41749479597460493, -10.00000000000000000 ) ) ;
#51381=ADVANCED_FACE ( 'NONE', ( #44425 ), #98661, .F. ) ;
#51395=DIRECTION ( 'NONE',  ( -1.000000000000000000, 0.000000000000000000, 0.000000000000000000 ) ) ;
#51398=DIRECTION ( 'NONE',  ( 0.000000000000000000, 0.000000000000000000, 1.000000000000000000 ) ) ;
#51400=LINE ( 'NONE', #7288, #66014 ) ;
#51403=ADVANCED_FACE ( 'NONE', ( #12555 ), #98156, .F. ) ;
#51405=ORIENTED_EDGE ( 'NONE', *, *, #88562, .T. ) ;
#51410=LINE ( 'NONE', #90469, #36625 ) ;
#51413=LINE ( 'NONE', #21042, #9607 ) ;
#51414=VECTOR ( 'NONE', #47181, 1000.000000000000000 ) ;
#51415=LINE ( 'NONE', #42797, #69055 ) ;
#51421=VERTEX_POINT ( 'NONE', #32217 ) ;
#51426=ORIENTED_EDGE ( 'NONE', *, *, #92487, .F. ) ;
#51430=DIRECTION ( 'NONE',  ( 0.4458072818673325943, 0.8951289669282637140, 0.000000000000000000 ) ) ;
#51434=VERTEX_POINT ( 'NONE', #7939 ) ;
#51437=ORIENTED_EDGE ( 'NONE', *, *, #90256, .T. ) ;
#51453=AXIS2_PLACEMENT_3D ( 'NONE', #4274, #97030, #69058 ) ;
#51455=ADVANCED_FACE ( 'NONE', ( #23109 ), #46922, .F. ) ;
#51458=LINE ( 'NONE', #42351, #65648 ) ;
#51459=AXIS2_PLACEMENT_3D ( 'NONE', #44222, #7222, #31021 ) ;
#51466=EDGE_LOOP ( 'NONE', ( #65823, #63855, #94439, #2457 ) ) ;
#51467=LINE ( 'NONE', #37743, #48426 ) ;
#51472=AXIS2_PLACEMENT_3D ( 'NONE', #73425, #71930, #2534 ) ;
#51480=VECTOR ( 'NONE', #84551, 1000.000000000000000 ) ;
#51483=CARTESIAN_POINT ( 'NONE',  ( 30.34687108590969373, 93.06504152958497400, 60.00000000000000000 ) ) ;
#51485=CARTESIAN_POINT ( 'NONE',  ( -69.42519150082246426, 45.64199051378594874, -10.00000000000000000 ) ) ;
#51490=AXIS2_PLACEMENT_3D ( 'NONE', #90069, #74363, #59602 ) ;
#51495=CARTESIAN_POINT ( 'NONE',  ( 33.63888670793727442, 47.67824751478843126, 10.00000000000000000 ) ) ;
#51511=VERTEX_POINT ( 'NONE', #820 ) ;
#51515=ADVANCED_FACE ( 'NONE', ( #47413 ), #53517, .F. ) ;
#51520=EDGE_LOOP ( 'NONE', ( #3630, #29238, #10404, #88959 ) ) ;
#51522=VECTOR ( 'NONE', #69995, 1000.000000000000227 ) ;
#51529=EDGE_LOOP ( 'NONE', ( #54009, #49545, #80400, #65485 ) ) ;
#51530=AXIS2_PLACEMENT_3D ( 'NONE', #40025, #32451, #39520 ) ;
#51536=VECTOR ( 'NONE', #58524, 1000.000000000000000 ) ;
#51545=VECTOR ( 'NONE', #99869, 1000.000000000000114 ) ;
#51547=DIRECTION ( 'NONE',  ( -0.000000000000000000, -0.000000000000000000, -1.000000000000000000 ) ) ;
#51549=DIRECTION ( 'NONE',  ( -0.9954322480537365347, -0.09547062131715938760, 0.000000000000000000 ) ) ;
#51556=ORIENTED_EDGE ( 'NONE', *, *, #61708, .F. ) ;
#51557=DIRECTION ( 'NONE',  ( 0.000000000000000000, 0.000000000000000000, 1.000000000000000000 ) ) ;
#51560=ORIENTED_EDGE ( 'NONE', *, *, #70067, .T. ) ;
#51561=AXIS2_PLACEMENT_3D ( 'NONE', #45600, #91753, #22316 ) ;
#51562=ORIENTED_EDGE ( 'NONE', *, *, #38452, .T. ) ;
#51568=LINE ( 'NONE', #21670, #41922 ) ;
#51571=EDGE_CURVE ( 'NONE', #74292, #34443, #49921, .T. ) ;
#51572=ORIENTED_EDGE ( 'NONE', *, *, #83461, .F. ) ;
#51582=CARTESIAN_POINT ( 'NONE',  ( 32.30839531297598910, 123.0650415295850593, 25.00000000000000000 ) ) ;
#51585=ADVANCED_FACE ( 'NONE', ( #55993 ), #63121, .T. ) ;
#51593=DIRECTION ( 'NONE',  ( -0.6625377181876236365, -0.7490285521785782219, 0.000000000000000000 ) ) ;
#51596=VECTOR ( 'NONE', #23025, 1000.000000000000114 ) ;
#51601=CIRCLE ( 'NONE', #4670, 70.00000000000001421 ) ;
#51604=AXIS2_PLACEMENT_3D ( 'NONE', #58553, #12486, #92484 ) ;
#51610=FACE_OUTER_BOUND ( 'NONE', #83492, .T. ) ;
#51637=CARTESIAN_POINT ( 'NONE',  ( -19.65312891409030271, 93.06504152958497400, -25.00000000000000000 ) ) ;
#51647=EDGE_CURVE ( 'NONE', #7148, #26012, #89953, .T. ) ;
#51650=CARTESIAN_POINT ( 'NONE',  ( -80.27490717900100492, 58.06504152958491005, -10.00000000000000888 ) ) ;
#51651=CARTESIAN_POINT ( 'NONE',  ( 49.10122569834316408, 93.29622288527660601, 10.00000000000000000 ) ) ;
#51652=DIRECTION ( 'NONE',  ( 1.000000000000000000, 0.000000000000000000, 0.000000000000000000 ) ) ;
#51655=CARTESIAN_POINT ( 'NONE',  ( 48.91227514082039107, 78.96591507484177441, 177.5919119679930134 ) ) ;
#51657=ORIENTED_EDGE ( 'NONE', *, *, #66927, .T. ) ;
#51659=LINE ( 'NONE', #74485, #55873 ) ;
#51662=EDGE_CURVE ( 'NONE', #3834, #43292, #88999, .T. ) ;
#51667=LINE ( 'NONE', #91191, #2757 ) ;
#51669=EDGE_LOOP ( 'NONE', ( #66654, #33755, #13943, #94338 ) ) ;
#51677=LINE ( 'NONE', #35467, #93660 ) ;
#51680=VECTOR ( 'NONE', #96039, 1000.000000000000114 ) ;
#51685=ORIENTED_EDGE ( 'NONE', *, *, #39701, .T. ) ;
#51686=AXIS2_PLACEMENT_3D ( 'NONE', #48774, #27475, #50251 ) ;
#51689=VERTEX_POINT ( 'NONE', #30608 ) ;
#51690=EDGE_CURVE ( 'NONE', #26616, #71493, #99591, .T. ) ;
#51700=EDGE_CURVE ( 'NONE', #77384, #10835, #15379, .T. ) ;
#51705=ORIENTED_EDGE ( 'NONE', *, *, #21665, .F. ) ;
#51706=LINE ( 'NONE', #75011, #46886 ) ;
#51710=EDGE_CURVE ( 'NONE', #59362, #62248, #71119, .T. ) ;
#51712=DIRECTION ( 'NONE',  ( -0.9576970189910627429, -0.2877784213863714968, 0.000000000000000000 ) ) ;
#51713=VECTOR ( 'NONE', #67720, 1000.000000000000000 ) ;
#51716=DIRECTION ( 'NONE',  ( -0.000000000000000000, 0.000000000000000000, 1.000000000000000000 ) ) ;
#51725=CARTESIAN_POINT ( 'NONE',  ( -19.65312891409030271, 93.06504152958497400, 177.5919119679930134 ) ) ;
#51726=ORIENTED_EDGE ( 'NONE', *, *, #80152, .T. ) ;
#51727=CARTESIAN_POINT ( 'NONE',  ( 34.97213163436671124, 51.32435524152969464, -10.00000000000000000 ) ) ;
#51746=ORIENTED_EDGE ( 'NONE', *, *, #17475, .T. ) ;
#51755=LINE ( 'NONE', #70302, #80876 ) ;
#51769=LINE ( 'NONE', #7137, #33616 ) ;
#51777=LINE ( 'NONE', #46131, #53123 ) ;
#51785=CARTESIAN_POINT ( 'NONE',  ( 48.38981961164311940, 109.5014996615669105, 10.00000000000000000 ) ) ;
#51786=EDGE_CURVE ( 'NONE', #55413, #95379, #97797, .T. ) ;
#51791=EDGE_CURVE ( 'NONE', #44322, #21181, #44050, .T. ) ;
#51794=ORIENTED_EDGE ( 'NONE', *, *, #57037, .F. ) ;
#51796=CARTESIAN_POINT ( 'NONE',  ( 32.80507291521585955, 117.6754530847557874, 59.99999999999999289 ) ) ;
#51798=ORIENTED_EDGE ( 'NONE', *, *, #56258, .F. ) ;
#51802=ORIENTED_EDGE ( 'NONE', *, *, #54833, .F. ) ;
#51811=ORIENTED_EDGE ( 'NONE', *, *, #36752, .F. ) ;
#51819=LINE ( 'NONE', #5217, #78742 ) ;
#51827=LINE ( 'NONE', #37104, #7352 ) ;
#51829=CARTESIAN_POINT ( 'NONE',  ( -15.61417992190811788, 23.18166087982996970, -10.00000000000000000 ) ) ;
#51832=CARTESIAN_POINT ( 'NONE',  ( 44.95821123098112082, 116.5722627105190270, -10.00000000000000000 ) ) ;
#51840=CARTESIAN_POINT ( 'NONE',  ( -75.14068524134967220, 52.46521621197197760, 10.00000000000000000 ) ) ;
#51842=EDGE_LOOP ( 'NONE', ( #63717, #38954, #53629, #17640 ) ) ;
#51855=CARTESIAN_POINT ( 'NONE',  ( -52.57320609282758994, 32.70376883311633520, -10.00000000000000000 ) ) ;
#51875=CARTESIAN_POINT ( 'NONE',  ( -19.65312891409030271, 93.06504152958497400, 10.00000000000000888 ) ) ;
#51883=DIRECTION ( 'NONE',  ( -0.7135562106085678868, 0.7005979833698787740, 0.000000000000000000 ) ) ;
#51888=DIRECTION ( 'NONE',  ( -0.6201213960746324583, 0.7845058662179964504, 0.000000000000000000 ) ) ;
#51892=ORIENTED_EDGE ( 'NONE', *, *, #28321, .T. ) ;
#51895=CARTESIAN_POINT ( 'NONE',  ( 29.30989995549245464, 44.80713248141895377, 10.00000000000000000 ) ) ;
#51899=DIRECTION ( 'NONE',  ( 0.2165469281463284490, -0.9762722099447412871, 0.000000000000000000 ) ) ;
#51906=LINE ( 'NONE', #82846, #87440 ) ;
#51907=VECTOR ( 'NONE', #51398, 1000.000000000000000 ) ;
#51915=DIRECTION ( 'NONE',  ( 0.1162373735601320568, 0.9932214622066130039, 0.000000000000000000 ) ) ;
#51926=ADVANCED_FACE ( 'NONE', ( #93804 ), #63857, .F. ) ;
#51929=DIRECTION ( 'NONE',  ( -0.9481851146622203297, -0.3177184104407421716, 0.000000000000000000 ) ) ;
#51930=ORIENTED_EDGE ( 'NONE', *, *, #70214, .F. ) ;
#51933=CARTESIAN_POINT ( 'NONE',  ( 48.53010236944518851, 101.9116055364396090, -10.00000000000000000 ) ) ;
#51938=PLANE ( 'NONE',  #39795 ) ;
#51942=ORIENTED_EDGE ( 'NONE', *, *, #54440, .T. ) ;
#51945=ORIENTED_EDGE ( 'NONE', *, *, #1316, .T. ) ;
#51948=ORIENTED_EDGE ( 'NONE', *, *, #7869, .T. ) ;
#51949=CARTESIAN_POINT ( 'NONE',  ( -18.95853632553436086, 41.33786475637849378, 59.99999999999999289 ) ) ;
#51957=EDGE_LOOP ( 'NONE', ( #17264, #39704, #32461, #5857 ) ) ;
#51960=ORIENTED_EDGE ( 'NONE', *, *, #99830, .T. ) ;
#51962=DIRECTION ( 'NONE',  ( 0.000000000000000000, 0.000000000000000000, 1.000000000000000000 ) ) ;
#51966=FACE_OUTER_BOUND ( 'NONE', #27529, .T. ) ;
#51970=VERTEX_POINT ( 'NONE', #50157 ) ;
#51972=CARTESIAN_POINT ( 'NONE',  ( -19.65312891409030271, 93.06504152958497400, 59.99999999999999289 ) ) ;
#51979=DIRECTION ( 'NONE',  ( 0.000000000000000000, 0.000000000000000000, 1.000000000000000000 ) ) ;
#51982=CARTESIAN_POINT ( 'NONE',  ( -19.65312891409030271, 93.06504152958497400, 177.5919119679930134 ) ) ;
#51983=DIRECTION ( 'NONE',  ( -1.000000000000000000, -9.785293164109648193E-14, 0.000000000000000000 ) ) ;
#51993=CARTESIAN_POINT ( 'NONE',  ( 9.830230629461709668, 30.95267373526312227, 10.00000000000000000 ) ) ;
#52003=LINE ( 'NONE', #46368, #4423 ) ;
#52017=CARTESIAN_POINT ( 'NONE',  ( -23.73952538801239598, 24.43184193311134678, 10.00000000000000000 ) ) ;
#52018=CARTESIAN_POINT ( 'NONE',  ( -2.590881078880516331, 25.17631125121048541, 177.5919119679930134 ) ) ;
#52020=EDGE_CURVE ( 'NONE', #62608, #63400, #51659, .T. ) ;
#52023=LINE ( 'NONE', #38160, #47225 ) ;
#52024=EDGE_LOOP ( 'NONE', ( #77211, #77321, #22998, #39936 ) ) ;
#52029=ADVANCED_FACE ( 'NONE', ( #97774 ), #58247, .F. ) ;
#52044=VECTOR ( 'NONE', #59599, 1000.000000000000227 ) ;
#52050=DIRECTION ( 'NONE',  ( -0.06142469166374898287, -0.9981117208278906805, 0.000000000000000000 ) ) ;
#52057=ORIENTED_EDGE ( 'NONE', *, *, #92557, .T. ) ;
#52060=EDGE_LOOP ( 'NONE', ( #49782, #18665, #4878, #79894 ) ) ;
#52062=DIRECTION ( 'NONE',  ( 0.3371987438498061929, -0.9414334852479556703, 0.000000000000000000 ) ) ;
#52068=DIRECTION ( 'NONE',  ( -1.000000000000000000, 0.000000000000000000, 0.000000000000000000 ) ) ;
#52072=ADVANCED_FACE ( 'NONE', ( #20267 ), #89226, .T. ) ;
#52084=CARTESIAN_POINT ( 'NONE',  ( -19.65312891409030271, 93.06504152958497400, 177.5919119679930134 ) ) ;
#52129=EDGE_CURVE ( 'NONE', #14868, #51421, #51415, .T. ) ;
#52133=FACE_OUTER_BOUND ( 'NONE', #8373, .T. ) ;
#52138=ORIENTED_EDGE ( 'NONE', *, *, #29834, .F. ) ;
#52157=LINE ( 'NONE', #73990, #22991 ) ;
#52158=ORIENTED_EDGE ( 'NONE', *, *, #51252, .T. ) ;
#52165=CARTESIAN_POINT ( 'NONE',  ( 17.55280445478281592, 33.77154675864928635, -10.00000000000000000 ) ) ;
#52186=ORIENTED_EDGE ( 'NONE', *, *, #61524, .F. ) ;
#52187=DIRECTION ( 'NONE',  ( 0.000000000000000000, 0.000000000000000000, 1.000000000000000000 ) ) ;
#52190=CARTESIAN_POINT ( 'NONE',  ( -19.65312891409030271, 93.06504152958497400, 59.99999999999999289 ) ) ;
#52200=EDGE_CURVE ( 'NONE', #20252, #14275, #24502, .T. ) ;
#52204=VECTOR ( 'NONE', #32807, 1000.000000000000000 ) ;
#52205=AXIS2_PLACEMENT_3D ( 'NONE', #58360, #81714, #36054 ) ;
#52212=CARTESIAN_POINT ( 'NONE',  ( -21.31413092498266693, 24.33771760303832465, 10.00000000000000000 ) ) ;
#52228=LINE ( 'NONE', #83173, #25427 ) ;
#52229=CARTESIAN_POINT ( 'NONE',  ( 6.499607544075114873, 41.35827422038750001, 59.99999999999999289 ) ) ;
#52233=EDGE_CURVE ( 'NONE', #92904, #213, #38514, .T. ) ;
#52245=CARTESIAN_POINT ( 'NONE',  ( -56.29836151245349640, 34.88994676555962116, -10.00000000000000000 ) ) ;
#52247=DIRECTION ( 'NONE',  ( -0.9995486091367047354, 0.03004293549037833494, 0.000000000000000000 ) ) ;
#52265=ORIENTED_EDGE ( 'NONE', *, *, #50367, .F. ) ;
#52271=VERTEX_POINT ( 'NONE', #35676 ) ;
#52279=ORIENTED_EDGE ( 'NONE', *, *, #67209, .T. ) ;
#52280=CARTESIAN_POINT ( 'NONE',  ( -56.06787742410712383, 34.75406423768147590, -10.00000000000000000 ) ) ;
#52287=VECTOR ( 'NONE', #70832, 1000.000000000000000 ) ;
#52290=DIRECTION ( 'NONE',  ( -0.8279987035736638967, -0.5607300124661883656, 0.000000000000000000 ) ) ;
#52291=CARTESIAN_POINT ( 'NONE',  ( -19.65312891409030271, 93.06504152958497400, 10.00000000000000888 ) ) ;
#52292=ORIENTED_EDGE ( 'NONE', *, *, #68143, .F. ) ;
#52296=VECTOR ( 'NONE', #19023, 1000.000000000000114 ) ;
#52304=ORIENTED_EDGE ( 'NONE', *, *, #74823, .F. ) ;
#52308=CARTESIAN_POINT ( 'NONE',  ( -54.45295541630240166, 33.76759809053437067, 10.00000000000000000 ) ) ;
#52309=CARTESIAN_POINT ( 'NONE',  ( 21.15788363470973366, 37.74176219324819215, -10.00000000000000000 ) ) ;
#52318=DIRECTION ( 'NONE',  ( -0.9825923819316307872, -0.1857746241280658905, 0.000000000000000000 ) ) ;
#52321=DIRECTION ( 'NONE',  ( 0.9946578707245736783, 0.1032265479692960342, 0.000000000000000000 ) ) ;
#52353=DIRECTION ( 'NONE',  ( -0.06442261589617466477, -0.9979227057047523886, 0.000000000000000000 ) ) ;
#52360=ORIENTED_EDGE ( 'NONE', *, *, #37387, .F. ) ;
#52361=VECTOR ( 'NONE', #95335, 1000.000000000000227 ) ;
#52362=EDGE_CURVE ( 'NONE', #89390, #50887, #64847, .T. ) ;
#52371=LINE ( 'NONE', #60455, #9310 ) ;
#52372=AXIS2_PLACEMENT_3D ( 'NONE', #12158, #27357, #89219 ) ;
#52375=ADVANCED_FACE ( 'NONE', ( #88699 ), #19270, .F. ) ;
#52385=LINE ( 'NONE', #81837, #58722 ) ;
#52399=ORIENTED_EDGE ( 'NONE', *, *, #30655, .F. ) ;
#52409=EDGE_LOOP ( 'NONE', ( #96441, #50404, #91097, #83948 ) ) ;
#52413=EDGE_CURVE ( 'NONE', #42773, #99043, #29716, .T. ) ;
#52414=VERTEX_POINT ( 'NONE', #13535 ) ;
#52416=ORIENTED_EDGE ( 'NONE', *, *, #33375, .T. ) ;
#52424=ORIENTED_EDGE ( 'NONE', *, *, #8357, .F. ) ;
#52429=LINE ( 'NONE', #13942, #65454 ) ;
#52430=EDGE_LOOP ( 'NONE', ( #41417, #42899, #209, #46400 ) ) ;
#52435=DIRECTION ( 'NONE',  ( -0.000000000000000000, -0.000000000000000000, 1.000000000000000000 ) ) ;
#52436=AXIS2_PLACEMENT_3D ( 'NONE', #72085, #71589, #95432 ) ;
#52439=ORIENTED_EDGE ( 'NONE', *, *, #40547, .F. ) ;
#52444=VECTOR ( 'NONE', #59731, 1000.000000000000114 ) ;
#52454=VERTEX_POINT ( 'NONE', #47148 ) ;
#52456=DIRECTION ( 'NONE',  ( -0.9825427565607343094, 0.1860369090531061309, 0.000000000000000000 ) ) ;
#52461=ADVANCED_FACE ( 'NONE', ( #63785 ), #32389, .F. ) ;
#52468=LINE ( 'NONE', #83919, #54425 ) ;
#52474=CYLINDRICAL_SURFACE ( 'NONE', #64554, 70.00000000000002842 ) ;
#52475=DIRECTION ( 'NONE',  ( 0.1384676192453727639, -0.9903669614948382716, 0.000000000000000000 ) ) ;
#52480=DIRECTION ( 'NONE',  ( 0.000000000000000000, -0.000000000000000000, -1.000000000000000000 ) ) ;
#52481=ADVANCED_FACE ( 'NONE', ( #56168 ), #96228, .F. ) ;
#52495=ORIENTED_EDGE ( 'NONE', *, *, #87890, .F. ) ;
#52500=VERTEX_POINT ( 'NONE', #20198 ) ;
#52503=CIRCLE ( 'NONE', #89790, 70.00000000000001421 ) ;
#52510=ORIENTED_EDGE ( 'NONE', *, *, #16007, .F. ) ;
#52515=VECTOR ( 'NONE', #57221, 1000.000000000000000 ) ;
#52516=VERTEX_POINT ( 'NONE', #97705 ) ;
#52517=PLANE ( 'NONE',  #29611 ) ;
#52518=PLANE ( 'NONE',  #20081 ) ;
#52529=LINE ( 'NONE', #83984, #47457 ) ;
#52550=DIRECTION ( 'NONE',  ( -0.9923183454821322691, -0.1237105541964931832, 0.000000000000000000 ) ) ;
#52555=DIRECTION ( 'NONE',  ( -0.000000000000000000, -0.000000000000000000, -1.000000000000000000 ) ) ;
#52564=VERTEX_POINT ( 'NONE', #4999 ) ;
#52566=CARTESIAN_POINT ( 'NONE',  ( -42.72532191160158987, 28.29708160126037697, -10.00000000000000000 ) ) ;
#52570=EDGE_CURVE ( 'NONE', #72875, #1030, #48013, .T. ) ;
#52572=AXIS2_PLACEMENT_3D ( 'NONE', #60499, #68117, #13448 ) ;
#52573=DIRECTION ( 'NONE',  ( -1.000000000000000000, 0.000000000000000000, 0.000000000000000000 ) ) ;
#52574=ADVANCED_FACE ( 'NONE', ( #35876 ), #57674, .F. ) ;
#52575=LINE ( 'NONE', #44977, #88417 ) ;
#52582=DIRECTION ( 'NONE',  ( -0.7763215174174871169, 0.6303371332823493045, 0.000000000000000000 ) ) ;
#52584=AXIS2_PLACEMENT_3D ( 'NONE', #41660, #80728, #4162 ) ;
#52586=DIRECTION ( 'NONE',  ( -0.9506327454577433445, -0.3103181967972122313, 0.000000000000000000 ) ) ;
#52594=DIRECTION ( 'NONE',  ( 1.000000000000000000, 0.000000000000000000, 0.000000000000000000 ) ) ;
#52596=DIRECTION ( 'NONE',  ( -0.07193265315671491800, 0.9974094913373522386, 0.000000000000000000 ) ) ;
#52599=AXIS2_PLACEMENT_3D ( 'NONE', #12231, #4113, #28404 ) ;
#52616=ORIENTED_EDGE ( 'NONE', *, *, #33215, .T. ) ;
#52623=CARTESIAN_POINT ( 'NONE',  ( 9.827979128326980174, 29.57595373812807082, 10.00000000000000000 ) ) ;
#52626=LINE ( 'NONE', #83584, #7721 ) ;
#52628=EDGE_CURVE ( 'NONE', #34863, #59430, #90119, .T. ) ;
#52636=CARTESIAN_POINT ( 'NONE',  ( -64.74139798177010618, 41.16849083240310847, 10.00000000000000000 ) ) ;
#52638=AXIS2_PLACEMENT_3D ( 'NONE', #67368, #61256, #35965 ) ;
#52642=CARTESIAN_POINT ( 'NONE',  ( -59.66199281916092900, 60.27061997932485582, 59.99999999999999289 ) ) ;
#52648=ADVANCED_FACE ( 'NONE', ( #34389 ), #51068, .F. ) ;
#52654=ORIENTED_EDGE ( 'NONE', *, *, #54389, .T. ) ;
#52662=FACE_BOUND ( 'NONE', #66990, .T. ) ;
#52670=VERTEX_POINT ( 'NONE', #50575 ) ;
#52671=CARTESIAN_POINT ( 'NONE',  ( -65.10162659358719850, 39.48459004765182812, -10.00000000000000000 ) ) ;
#52686=VECTOR ( 'NONE', #1879, 999.9999999999998863 ) ;
#52692=CARTESIAN_POINT ( 'NONE',  ( 47.84007798744509898, 106.1754093786579318, -10.00000000000000000 ) ) ;
#52700=AXIS2_PLACEMENT_3D ( 'NONE', #53099, #89662, #20725 ) ;
#52707=AXIS2_PLACEMENT_3D ( 'NONE', #62179, #85558, #54574 ) ;
#52733=LINE ( 'NONE', #22350, #6115 ) ;
#52743=ADVANCED_FACE ( 'NONE', ( #65287 ), #3987, .F. ) ;
#52747=CARTESIAN_POINT ( 'NONE',  ( -71.61465314115659453, 63.06504152958490295, 25.00000000000000000 ) ) ;
#52752=FACE_OUTER_BOUND ( 'NONE', #98802, .T. ) ;
#52759=ORIENTED_EDGE ( 'NONE', *, *, #67637, .T. ) ;
#52765=EDGE_CURVE ( 'NONE', #99548, #48481, #4484, .T. ) ;
#52776=CARTESIAN_POINT ( 'NONE',  ( -6.926766666751215773, 73.70349067594094095, 14.94635119574900450 ) ) ;
#52779=CARTESIAN_POINT ( 'NONE',  ( 27.76992210170819675, 43.29297894285233639, -10.00000000000000000 ) ) ;
#52781=VECTOR ( 'NONE', #11599, 1000.000000000000227 ) ;
#52788=CARTESIAN_POINT ( 'NONE',  ( 18.86034532297697908, 34.61239144260638767, 177.5919119679930134 ) ) ;
#52795=CARTESIAN_POINT ( 'NONE',  ( -19.65312891409030271, 93.06504152958497400, 10.00000000000000888 ) ) ;
#52800=ORIENTED_EDGE ( 'NONE', *, *, #17035, .F. ) ;
#52804=ADVANCED_FACE ( 'NONE', ( #67781 ), #29290, .F. ) ;
#52823=AXIS2_PLACEMENT_3D ( 'NONE', #94988, #77242, #63536 ) ;
#52824=FACE_OUTER_BOUND ( 'NONE', #66620, .T. ) ;
#52825=VECTOR ( 'NONE', #68514, 1000.000000000000000 ) ;
#52826=ORIENTED_EDGE ( 'NONE', *, *, #89306, .T. ) ;
#52834=VECTOR ( 'NONE', #23144, 1000.000000000000000 ) ;
#52835=CYLINDRICAL_SURFACE ( 'NONE', #40251, 49.99999999999999289 ) ;
#52838=CARTESIAN_POINT ( 'NONE',  ( -16.99542894172669349, 24.36904009834038476, -10.00000000000000000 ) ) ;
#52842=ORIENTED_EDGE ( 'NONE', *, *, #13925, .T. ) ;
#52846=LINE ( 'NONE', #21460, #5934 ) ;
#52856=DIRECTION ( 'NONE',  ( 0.4805540241036304616, 0.8769651246872975925, 0.000000000000000000 ) ) ;
#52865=DIRECTION ( 'NONE',  ( -0.04056776950002415755, 0.9991767892008865948, 0.000000000000000000 ) ) ;
#52870=VERTEX_POINT ( 'NONE', #24667 ) ;
#52878=ADVANCED_FACE ( 'NONE', ( #10481 ), #56568, .F. ) ;
#52881=EDGE_CURVE ( 'NONE', #3988, #4641, #8477, .T. ) ;
#52893=FACE_OUTER_BOUND ( 'NONE', #32508, .T. ) ;
#52895=ORIENTED_EDGE ( 'NONE', *, *, #62985, .T. ) ;
#52898=DIRECTION ( 'NONE',  ( 0.000000000000000000, 0.000000000000000000, 1.000000000000000000 ) ) ;
#52902=ORIENTED_EDGE ( 'NONE', *, *, #18879, .T. ) ;
#52908=ORIENTED_EDGE ( 'NONE', *, *, #36937, .T. ) ;
#52913=VERTEX_POINT ( 'NONE', #66664 ) ;
#52915=CARTESIAN_POINT ( 'NONE',  ( -19.65312891409030271, 93.06504152958497400, 177.5919119679930134 ) ) ;
#52918=VECTOR ( 'NONE', #50094, 1000.000000000000000 ) ;
#52920=AXIS2_PLACEMENT_3D ( 'NONE', #81439, #82933, #98107 ) ;
#52938=VERTEX_POINT ( 'NONE', #10997 ) ;
#52940=EDGE_CURVE ( 'NONE', #67772, #22139, #81912, .T. ) ;
#52941=VECTOR ( 'NONE', #89213, 1000.000000000000000 ) ;
#52943=CARTESIAN_POINT ( 'NONE',  ( -58.10760318826260118, 36.06970723555269842, -10.00000000000000000 ) ) ;
#52947=EDGE_CURVE ( 'NONE', #100252, #51318, #10724, .T. ) ;
#52958=CARTESIAN_POINT ( 'NONE',  ( 47.54560441532652959, 78.55524412553474178, -10.00000000000000000 ) ) ;
#52961=CARTESIAN_POINT ( 'NONE',  ( 17.38248943320504836, 35.13769309531819829, -10.00000000000000000 ) ) ;
#52964=DIRECTION ( 'NONE',  ( 1.000000000000000000, 0.000000000000000000, 0.000000000000000000 ) ) ;
#52974=VECTOR ( 'NONE', #28575, 1000.000000000000000 ) ;
#52983=AXIS2_PLACEMENT_3D ( 'NONE', #80869, #58008, #34702 ) ;
#52997=ORIENTED_EDGE ( 'NONE', *, *, #39960, .T. ) ;
#53000=CARTESIAN_POINT ( 'NONE',  ( -19.65312891409030271, 93.06504152958497400, -10.00000000000000888 ) ) ;
#53009=AXIS2_PLACEMENT_3D ( 'NONE', #44867, #5888, #67180 ) ;
#53010=ORIENTED_EDGE ( 'NONE', *, *, #6634, .T. ) ;
#53012=EDGE_LOOP ( 'NONE', ( #57739, #71402, #37712, #94055 ) ) ;
#53015=VERTEX_POINT ( 'NONE', #4886 ) ;
#53016=ADVANCED_FACE ( 'NONE', ( #74795 ), #35768, .T. ) ;
#53026=CARTESIAN_POINT ( 'NONE',  ( -59.91704162537831735, 50.38415623799413368, 59.99999999999999289 ) ) ;
#53034=CARTESIAN_POINT ( 'NONE',  ( -19.62460808985983363, 93.20396705361855538, 59.99999999999999289 ) ) ;
#53038=CIRCLE ( 'NONE', #14212, 70.00000000000001421 ) ;
#53048=VECTOR ( 'NONE', #42350, 1000.000000000000227 ) ;
#53056=CARTESIAN_POINT ( 'NONE',  ( 43.35468487962021555, 120.5828561944265687, 10.00000000000000000 ) ) ;
#53060=ORIENTED_EDGE ( 'NONE', *, *, #51662, .F. ) ;
#53065=VECTOR ( 'NONE', #66807, 1000.000000000000000 ) ;
#53078=CARTESIAN_POINT ( 'NONE',  ( -19.65312891409030271, 93.06504152958497400, 10.00000000000000888 ) ) ;
#53087=CARTESIAN_POINT ( 'NONE',  ( 40.82928596147627331, 60.38352576601455723, -10.00000000000000000 ) ) ;
#53099=CARTESIAN_POINT ( 'NONE',  ( 21.15788363470973366, 37.74176219324819215, -10.00000000000000000 ) ) ;
#53107=VECTOR ( 'NONE', #30944, 1000.000000000000000 ) ;
#53108=PLANE ( 'NONE',  #62687 ) ;
#53118=VECTOR ( 'NONE', #78609, 1000.000000000000000 ) ;
#53122=DIRECTION ( 'NONE',  ( 1.000000000000000000, 0.000000000000000000, 0.000000000000000000 ) ) ;
#53123=VECTOR ( 'NONE', #31440, 1000.000000000000114 ) ;
#53135=LINE ( 'NONE', #21252, #87880 ) ;
#53139=LINE ( 'NONE', #98772, #86191 ) ;
#53141=ORIENTED_EDGE ( 'NONE', *, *, #42937, .T. ) ;
#53146=ORIENTED_EDGE ( 'NONE', *, *, #40273, .T. ) ;
#53147=PLANE ( 'NONE',  #85439 ) ;
#53155=DIRECTION ( 'NONE',  ( 1.000000000000000000, 0.000000000000000000, 0.000000000000000000 ) ) ;
#53157=CARTESIAN_POINT ( 'NONE',  ( 40.96864935082037817, 128.0650415295850735, 10.00000000000000888 ) ) ;
#53171=ORIENTED_EDGE ( 'NONE', *, *, #14609, .T. ) ;
#53172=PLANE ( 'NONE',  #52638 ) ;
#53173=ORIENTED_EDGE ( 'NONE', *, *, #28011, .F. ) ;
#53175=FACE_BOUND ( 'NONE', #85142, .T. ) ;
#53179=PLANE ( 'NONE',  #9458 ) ;
#53183=LINE ( 'NONE', #38469, #5838 ) ;
#53184=CIRCLE ( 'NONE', #37042, 0.1418229129680863287 ) ;
#53188=DIRECTION ( 'NONE',  ( -0.5372068985985075651, -0.8434505012732950169, 0.000000000000000000 ) ) ;
#53195=CARTESIAN_POINT ( 'NONE',  ( -19.51267218670369985, 93.08467941069811502, 59.99999999999999289 ) ) ;
#53203=AXIS2_PLACEMENT_3D ( 'NONE', #98024, #34707, #50902 ) ;
#53210=VERTEX_POINT ( 'NONE', #96494 ) ;
#53214=CIRCLE ( 'NONE', #87290, 70.00000000000001421 ) ;
#53219=LINE ( 'NONE', #84170, #24065 ) ;
#53224=DIRECTION ( 'NONE',  ( -0.5435407515102096410, 0.8393827800519358950, 0.000000000000000000 ) ) ;
#53241=AXIS2_PLACEMENT_3D ( 'NONE', #87356, #2687, #9276 ) ;
#53257=VECTOR ( 'NONE', #20585, 1000.000000000000000 ) ;
#53262=DIRECTION ( 'NONE',  ( -0.000000000000000000, -0.000000000000000000, -1.000000000000000000 ) ) ;
#53264=CARTESIAN_POINT ( 'NONE',  ( -19.65312891409030271, 93.06504152958497400, 177.5919119679930134 ) ) ;
#53266=EDGE_CURVE ( 'NONE', #48579, #45907, #73663, .T. ) ;
#53267=EDGE_LOOP ( 'NONE', ( #38120, #14022, #9074, #29116 ) ) ;
#53268=VECTOR ( 'NONE', #15125, 1000.000000000000000 ) ;
#53277=ORIENTED_EDGE ( 'NONE', *, *, #45087, .F. ) ;
#53279=EDGE_CURVE ( 'NONE', #32899, #48736, #56941, .T. ) ;
#53280=AXIS2_PLACEMENT_3D ( 'NONE', #68680, #53481, #14977 ) ;
#53288=CARTESIAN_POINT ( 'NONE',  ( -9.661182929849102763, 72.23920645719188371, 14.90246908070922061 ) ) ;
#53290=DIRECTION ( 'NONE',  ( -0.8816062427480089170, -0.4719856276919233706, 0.000000000000000000 ) ) ;
#53293=ORIENTED_EDGE ( 'NONE', *, *, #62968, .F. ) ;
#53298=CARTESIAN_POINT ( 'NONE',  ( -19.51633657099221963, 93.10247939160333885, 59.99999999999999289 ) ) ;
#53303=LINE ( 'NONE', #30507, #27308 ) ;
#53314=EDGE_LOOP ( 'NONE', ( #4693, #32877, #80634, #24988 ) ) ;
#53317=CARTESIAN_POINT ( 'NONE',  ( -38.35373792487678202, 26.90998726756845727, -10.00000000000000000 ) ) ;
#53321=VECTOR ( 'NONE', #25726, 1000.000000000000000 ) ;
#53322=CARTESIAN_POINT ( 'NONE',  ( -19.65312891409030271, 93.06504152958497400, 10.00000000000000888 ) ) ;
#53328=AXIS2_PLACEMENT_3D ( 'NONE', #22058, #40236, #8852 ) ;
#53336=EDGE_CURVE ( 'NONE', #24759, #23902, #47851, .T. ) ;
#53339=CARTESIAN_POINT ( 'NONE',  ( -12.10640029135213247, 60.69888763781672480, -10.00000000000000000 ) ) ;
#53342=DIRECTION ( 'NONE',  ( -0.000000000000000000, -0.000000000000000000, -1.000000000000000000 ) ) ;
#53356=CIRCLE ( 'NONE', #50111, 49.99999999999999289 ) ;
#53366=CARTESIAN_POINT ( 'NONE',  ( -76.99869489832862257, 52.47050021824117749, 10.00000000000000000 ) ) ;
#53369=CARTESIAN_POINT ( 'NONE',  ( 47.54560441532652959, 78.55524412553474178, 10.00000000000000000 ) ) ;
#53371=ORIENTED_EDGE ( 'NONE', *, *, #53823, .F. ) ;
#53377=CARTESIAN_POINT ( 'NONE',  ( -28.78056054657191964, 23.66266410781090457, 177.5919119679930134 ) ) ;
#53379=EDGE_CURVE ( 'NONE', #74122, #11056, #11869, .T. ) ;
#53381=LINE ( 'NONE', #44774, #91100 ) ;
#53385=FACE_OUTER_BOUND ( 'NONE', #61617, .T. ) ;
#53386=FACE_OUTER_BOUND ( 'NONE', #41463, .T. ) ;
#53388=ORIENTED_EDGE ( 'NONE', *, *, #45758, .T. ) ;
#53393=AXIS2_PLACEMENT_3D ( 'NONE', #57530, #58040, #3850 ) ;
#53400=VERTEX_POINT ( 'NONE', #97000 ) ;
#53407=ORIENTED_EDGE ( 'NONE', *, *, #76295, .F. ) ;
#53426=DIRECTION ( 'NONE',  ( -0.2805612043866717586, -0.9598361373656965068, 0.000000000000000000 ) ) ;
#53433=FACE_OUTER_BOUND ( 'NONE', #22168, .T. ) ;
#53437=CARTESIAN_POINT ( 'NONE',  ( 50.26447705663007071, 96.46038765672592774, 177.5919119679930134 ) ) ;
#53439=LINE ( 'NONE', #31627, #58111 ) ;
#53444=EDGE_LOOP ( 'NONE', ( #83965, #37218, #79262, #26241 ) ) ;
#53445=ORIENTED_EDGE ( 'NONE', *, *, #69772, .F. ) ;
#53450=CARTESIAN_POINT ( 'NONE',  ( -19.72794058414494245, 93.18552784692582236, 59.99999999999999289 ) ) ;
#53453=CARTESIAN_POINT ( 'NONE',  ( 40.48539884740146277, 126.3902902409112556, 10.00000000000000000 ) ) ;
#53457=DIRECTION ( 'NONE',  ( 0.2471055264905481497, -0.9689885751534065284, 0.000000000000000000 ) ) ;
#53466=ADVANCED_FACE ( 'NONE', ( #52824 ), #36627, .F. ) ;
#53470=CARTESIAN_POINT ( 'NONE',  ( -19.65312891409030271, 93.06504152958497400, 10.00000000000000888 ) ) ;
#53472=EDGE_CURVE ( 'NONE', #25048, #36314, #65664, .T. ) ;
#53474=DIRECTION ( 'NONE',  ( 0.2500151307524129951, -0.9682419296822740717, 0.000000000000000000 ) ) ;
#53481=DIRECTION ( 'NONE',  ( 0.000000000000000000, 0.000000000000000000, 1.000000000000000000 ) ) ;
#53484=CARTESIAN_POINT ( 'NONE',  ( -63.67680148659454886, 65.89705432001115071, 59.99999999999999289 ) ) ;
#53489=LINE ( 'NONE', #75828, #31321 ) ;
#53495=EDGE_CURVE ( 'NONE', #39796, #526, #20460, .T. ) ;
#53500=CARTESIAN_POINT ( 'NONE',  ( -19.60272883349852435, 92.93247618524840448, 59.99999999999999289 ) ) ;
#53502=EDGE_CURVE ( 'NONE', #861, #74959, #75651, .T. ) ;
#53508=CARTESIAN_POINT ( 'NONE',  ( -19.65312891409030271, 93.06504152958497400, -10.00000000000000888 ) ) ;
#53512=EDGE_CURVE ( 'NONE', #15461, #12944, #15529, .T. ) ;
#53515=DIRECTION ( 'NONE',  ( -0.000000000000000000, 0.000000000000000000, -1.000000000000000000 ) ) ;
#53517=PLANE ( 'NONE',  #43157 ) ;
#53521=DIRECTION ( 'NONE',  ( -0.5000000000000012212, 0.8660254037844378194, -0.000000000000000000 ) ) ;
#53524=VERTEX_POINT ( 'NONE', #5251 ) ;
#53529=FACE_OUTER_BOUND ( 'NONE', #50916, .T. ) ;
#53539=DIRECTION ( 'NONE',  ( -1.000000000000000000, 0.000000000000000000, 0.000000000000000000 ) ) ;
#53546=DIRECTION ( 'NONE',  ( 1.000000000000000000, 0.000000000000000000, 0.000000000000000000 ) ) ;
#53549=CARTESIAN_POINT ( 'NONE',  ( -29.91485116994501325, 25.08783183303773967, -10.00000000000000000 ) ) ;
#53552=VECTOR ( 'NONE', #53853, 1000.000000000000114 ) ;
#53554=CARTESIAN_POINT ( 'NONE',  ( -72.39633208959961053, 47.04162880533179703, 177.5919119679930134 ) ) ;
#53555=DIRECTION ( 'NONE',  ( -0.000000000000000000, -0.000000000000000000, -1.000000000000000000 ) ) ;
#53559=DIRECTION ( 'NONE',  ( -1.000000000000000000, 0.000000000000000000, 0.000000000000000000 ) ) ;
#53560=LINE ( 'NONE', #68762, #80816 ) ;
#53568=DIRECTION ( 'NONE',  ( 0.000000000000000000, 0.000000000000000000, 1.000000000000000000 ) ) ;
#53578=DIRECTION ( 'NONE',  ( 0.000000000000000000, 0.000000000000000000, 1.000000000000000000 ) ) ;
#53579=EDGE_CURVE ( 'NONE', #36145, #43174, #91370, .T. ) ;
#53585=CARTESIAN_POINT ( 'NONE',  ( -36.52772323645827868, 26.41323893245353105, 10.00000000000000000 ) ) ;
#53591=EDGE_CURVE ( 'NONE', #86862, #28142, #83779, .T. ) ;
#53598=CARTESIAN_POINT ( 'NONE',  ( 48.95103868752456577, 97.61288834769685252, -10.00000000000000000 ) ) ;
#53610=LINE ( 'NONE', #54101, #25063 ) ;
#53614=ADVANCED_FACE ( 'NONE', ( #22435 ), #28534, .F. ) ;
#53627=DIRECTION ( 'NONE',  ( 0.000000000000000000, 0.000000000000000000, -1.000000000000000000 ) ) ;
#53629=ORIENTED_EDGE ( 'NONE', *, *, #59693, .F. ) ;
#53631=CARTESIAN_POINT ( 'NONE',  ( -37.96271243472389756, 25.23297040071578223, 10.00000000000000000 ) ) ;
#53632=DIRECTION ( 'NONE',  ( -0.4803199113995137437, 0.8770933717188629242, 0.000000000000000000 ) ) ;
#53634=VERTEX_POINT ( 'NONE', #20971 ) ;
#53635=LINE ( 'NONE', #85084, #7727 ) ;
#53636=DIRECTION ( 'NONE',  ( -0.5891075386695772131, -0.8080546441192405505, 0.000000000000000000 ) ) ;
#53654=EDGE_LOOP ( 'NONE', ( #87777, #69174, #33131, #7944 ) ) ;
#53655=FACE_BOUND ( 'NONE', #31941, .T. ) ;
#53668=ADVANCED_FACE ( 'NONE', ( #41490 ), #40976, .F. ) ;
#53675=CARTESIAN_POINT ( 'NONE',  ( 24.55112987542764458, 40.41347472807389352, 10.00000000000000000 ) ) ;
#53676=ORIENTED_EDGE ( 'NONE', *, *, #99265, .F. ) ;
#53682=DIRECTION ( 'NONE',  ( -0.000000000000000000, -0.000000000000000000, -1.000000000000000000 ) ) ;
#53685=CARTESIAN_POINT ( 'NONE',  ( -21.58168810074490551, 24.33735145887882112, -10.00000000000000000 ) ) ;
#53689=ORIENTED_EDGE ( 'NONE', *, *, #81984, .F. ) ;
#53698=CARTESIAN_POINT ( 'NONE',  ( -19.65312891409030271, 93.06504152958497400, -20.00000000000000355 ) ) ;
#53705=FACE_OUTER_BOUND ( 'NONE', #36359, .T. ) ;
#53712=VECTOR ( 'NONE', #27641, 1000.000000000000000 ) ;
#53716=DIRECTION ( 'NONE',  ( 0.5344452582589497291, -0.8452030915256549815, 0.000000000000000000 ) ) ;
#53738=ORIENTED_EDGE ( 'NONE', *, *, #44824, .T. ) ;
#53739=CARTESIAN_POINT ( 'NONE',  ( -17.26243516413818924, 24.35187462261283997, -10.00000000000000000 ) ) ;
#53744=DIRECTION ( 'NONE',  ( 0.2701803667135113662, 0.9628097264997651505, 0.000000000000000000 ) ) ;
#53748=ORIENTED_EDGE ( 'NONE', *, *, #44937, .F. ) ;
#53752=PLANE ( 'NONE',  #45908 ) ;
#53760=EDGE_CURVE ( 'NONE', #65497, #27171, #20713, .T. ) ;
#53761=EDGE_LOOP ( 'NONE', ( #28203, #70634, #92224, #27994 ) ) ;
#53763=CARTESIAN_POINT ( 'NONE',  ( -20.01016364259690405, 23.06595206263087050, -10.00000000000000000 ) ) ;
#53768=CARTESIAN_POINT ( 'NONE',  ( -10.31370568705291291, 72.11042850481820210, 14.81003180042302425 ) ) ;
#53775=DIRECTION ( 'NONE',  ( -0.7352104281592295454, 0.6778389383370672094, 0.000000000000000000 ) ) ;
#53778=CARTESIAN_POINT ( 'NONE',  ( 5.871984111234073822, 29.22396284167520619, -10.00000000000000000 ) ) ;
#53785=LINE ( 'NONE', #52308, #6248 ) ;
#53786=LINE ( 'NONE', #83247, #91379 ) ;
#53798=ORIENTED_EDGE ( 'NONE', *, *, #11962, .F. ) ;
#53804=AXIS2_PLACEMENT_3D ( 'NONE', #55409, #40720, #31614 ) ;
#53805=LINE ( 'NONE', #83268, #64267 ) ;
#53807=CARTESIAN_POINT ( 'NONE',  ( 49.09245556086620610, 93.56363653685789927, 10.00000000000000000 ) ) ;
#53817=CARTESIAN_POINT ( 'NONE',  ( 50.18541494347881837, 88.31343213334855591, 10.00000000000000000 ) ) ;
#53820=ADVANCED_FACE ( 'NONE', ( #54561 ), #38374, .F. ) ;
#53823=EDGE_CURVE ( 'NONE', #81228, #58030, #36890, .T. ) ;
#53824=DIRECTION ( 'NONE',  ( 0.9995565931350004485, 0.02977611660964677581, 0.000000000000000000 ) ) ;
#53825=ORIENTED_EDGE ( 'NONE', *, *, #27427, .F. ) ;
#53826=EDGE_CURVE ( 'NONE', #28514, #74953, #98724, .T. ) ;
#53853=DIRECTION ( 'NONE',  ( 0.4174706225611763410, 0.9086904199442095154, 0.000000000000000000 ) ) ;
#53857=ORIENTED_EDGE ( 'NONE', *, *, #47887, .F. ) ;
#53859=DIRECTION ( 'NONE',  ( 0.000000000000000000, 0.000000000000000000, 1.000000000000000000 ) ) ;
#53863=CARTESIAN_POINT ( 'NONE',  ( 40.08283240419611815, 56.57374221892477095, 177.5919119679930134 ) ) ;
#53871=EDGE_LOOP ( 'NONE', ( #96380, #65887, #333, #47912 ) ) ;
#53873=DIRECTION ( 'NONE',  ( -0.1857746241280658905, 0.9825923819316307872, 0.000000000000000000 ) ) ;
#53883=ORIENTED_EDGE ( 'NONE', *, *, #83623, .F. ) ;
#53893=ORIENTED_EDGE ( 'NONE', *, *, #38220, .F. ) ;
#53907=CARTESIAN_POINT ( 'NONE',  ( 44.44844410339183582, 68.22168590943847732, -10.00000000000000000 ) ) ;
#53908=LINE ( 'NONE', #69622, #9523 ) ;
#53938=CARTESIAN_POINT ( 'NONE',  ( -19.65312891409030271, 93.06504152958497400, -10.00000000000000888 ) ) ;
#53947=EDGE_CURVE ( 'NONE', #15950, #73688, #54354, .T. ) ;
#53961=VERTEX_POINT ( 'NONE', #68287 ) ;
#53981=ORIENTED_EDGE ( 'NONE', *, *, #42302, .T. ) ;
#53982=DIRECTION ( 'NONE',  ( 0.9834470158338940449, 0.1811959355156967932, 0.000000000000000000 ) ) ;
#53984=DIRECTION ( 'NONE',  ( 0.9979227057047517224, -0.06442261589618512863, 0.000000000000000000 ) ) ;
#53988=ORIENTED_EDGE ( 'NONE', *, *, #93756, .T. ) ;
#53991=EDGE_LOOP ( 'NONE', ( #3176, #41858, #61958, #87676 ) ) ;
#53994=ORIENTED_EDGE ( 'NONE', *, *, #29323, .F. ) ;
#54000=ADVANCED_FACE ( 'NONE', ( #37872 ), #68782, .F. ) ;
#54004=LINE ( 'NONE', #63503, #56236 ) ;
#54008=EDGE_LOOP ( 'NONE', ( #56621, #49044, #21530, #97449 ) ) ;
#54009=ORIENTED_EDGE ( 'NONE', *, *, #97551, .F. ) ;
#54013=DIRECTION ( 'NONE',  ( 0.7278481391575631898, -0.6857383512134002101, 0.000000000000000000 ) ) ;
#54016=CARTESIAN_POINT ( 'NONE',  ( 21.22187778180244422, 61.35672868576827454, 59.99999999999999289 ) ) ;
#54019=EDGE_CURVE ( 'NONE', #49232, #93683, #84043, .T. ) ;
#54027=ORIENTED_EDGE ( 'NONE', *, *, #57179, .T. ) ;
#54031=CARTESIAN_POINT ( 'NONE',  ( 29.12701137275935181, 44.61184105132205957, 10.00000000000000000 ) ) ;
#54039=ORIENTED_EDGE ( 'NONE', *, *, #84658, .T. ) ;
#54045=LINE ( 'NONE', #83016, #68813 ) ;
#54052=CARTESIAN_POINT ( 'NONE',  ( -19.65312891409030271, 93.06504152958497400, -10.00000000000000888 ) ) ;
#54053=EDGE_CURVE ( 'NONE', #33736, #79982, #34999, .T. ) ;
#54056=CARTESIAN_POINT ( 'NONE',  ( -71.07364842061384991, 47.42355933771584375, -10.00000000000000000 ) ) ;
#54061=CARTESIAN_POINT ( 'NONE',  ( -19.65312891409030271, 93.06504152958497400, 177.5919119679930134 ) ) ;
#54068=DIRECTION ( 'NONE',  ( -0.5280678506503699854, -0.8492021815265776707, 0.000000000000000000 ) ) ;
#54070=ADVANCED_FACE ( 'NONE', ( #10493 ), #47482, .T. ) ;
#54073=CARTESIAN_POINT ( 'NONE',  ( 43.35468487962021555, 120.5828561944265687, -10.00000000000000000 ) ) ;
#54077=CARTESIAN_POINT ( 'NONE',  ( 49.32130651720206771, 81.12656353050643077, 10.00000000000000000 ) ) ;
#54078=EDGE_CURVE ( 'NONE', #79909, #95521, #16586, .T. ) ;
#54101=CARTESIAN_POINT ( 'NONE',  ( -72.30469571560091424, 48.86078274006646183, -10.00000000000000000 ) ) ;
#54107=CARTESIAN_POINT ( 'NONE',  ( -66.76220315631053381, 40.93860057710854505, 10.00000000000000000 ) ) ;
#54113=VERTEX_POINT ( 'NONE', #33287 ) ;
#54114=ORIENTED_EDGE ( 'NONE', *, *, #7018, .T. ) ;
#54117=DIRECTION ( 'NONE',  ( -0.8718556560469457040, -0.4897629171537489778, 0.000000000000000000 ) ) ;
#54118=VERTEX_POINT ( 'NONE', #8494 ) ;
#54120=DIRECTION ( 'NONE',  ( 0.000000000000000000, 0.000000000000000000, 1.000000000000000000 ) ) ;
#54141=DIRECTION ( 'NONE',  ( 0.000000000000000000, 0.000000000000000000, 1.000000000000000000 ) ) ;
#54142=VERTEX_POINT ( 'NONE', #2920 ) ;
#54147=EDGE_CURVE ( 'NONE', #27723, #40468, #70573, .T. ) ;
#54173=VERTEX_POINT ( 'NONE', #39364 ) ;
#54187=CARTESIAN_POINT ( 'NONE',  ( 11.76667899187106059, 31.90941714274742225, -10.00000000000000000 ) ) ;
#54191=EDGE_CURVE ( 'NONE', #78972, #54142, #77079, .T. ) ;
#54195=PLANE ( 'NONE',  #88447 ) ;
#54198=ORIENTED_EDGE ( 'NONE', *, *, #25170, .T. ) ;
#54212=VECTOR ( 'NONE', #99406, 999.9999999999998863 ) ;
#54218=EDGE_CURVE ( 'NONE', #79838, #5025, #21583, .T. ) ;
#54229=CARTESIAN_POINT ( 'NONE',  ( 22.87549206224920084, 39.05096577487528720, -10.00000000000000000 ) ) ;
#54232=DIRECTION ( 'NONE',  ( -0.9628097264997621529, 0.2701803667135219689, 0.000000000000000000 ) ) ;
#54244=CARTESIAN_POINT ( 'NONE',  ( -66.76220315631053381, 40.93860057710854505, -10.00000000000000000 ) ) ;
#54246=DIRECTION ( 'NONE',  ( 0.000000000000000000, 0.000000000000000000, 1.000000000000000000 ) ) ;
#54249=EDGE_CURVE ( 'NONE', #213, #74292, #52468, .T. ) ;
#54251=CARTESIAN_POINT ( 'NONE',  ( -19.65312891409030271, 93.06504152958497400, 10.00000000000000888 ) ) ;
#54253=ORIENTED_EDGE ( 'NONE', *, *, #65131, .F. ) ;
#54256=EDGE_LOOP ( 'NONE', ( #97916, #18407, #45667, #76254 ) ) ;
#54260=ORIENTED_EDGE ( 'NONE', *, *, #76046, .T. ) ;
#54262=CARTESIAN_POINT ( 'NONE',  ( -12.28396743053746398, 72.06898478986710188, 14.42833059486102698 ) ) ;
#54263=DIRECTION ( 'NONE',  ( -1.000000000000000000, 0.000000000000000000, 0.000000000000000000 ) ) ;
#54264=LINE ( 'NONE', #67493, #3054 ) ;
#54265=AXIS2_PLACEMENT_3D ( 'NONE', #9593, #55153, #25791 ) ;
#54269=ORIENTED_EDGE ( 'NONE', *, *, #9792, .F. ) ;
#54289=DIRECTION ( 'NONE',  ( -0.9985601716053730259, 0.05364311403570636710, 0.000000000000000000 ) ) ;
#54298=EDGE_CURVE ( 'NONE', #83576, #27174, #30168, .T. ) ;
#54305=LINE ( 'NONE', #62925, #43352 ) ;
#54314=DIRECTION ( 'NONE',  ( -0.9890802632347809320, 0.1473778574936430164, 0.000000000000000000 ) ) ;
#54318=CARTESIAN_POINT ( 'NONE',  ( 41.10245927640360009, 127.8322459559854138, 10.00000000000000000 ) ) ;
#54326=CARTESIAN_POINT ( 'NONE',  ( 8.106622824862185439, 30.17147933776455204, -10.00000000000000000 ) ) ;
#54327=LINE ( 'NONE', #71072, #12539 ) ;
#54328=LINE ( 'NONE', #29080, #70151 ) ;
#54342=ADVANCED_FACE ( 'NONE', ( #94503 ), #17464, .T. ) ;
#54345=PLANE ( 'NONE',  #75997 ) ;
#54347=ORIENTED_EDGE ( 'NONE', *, *, #63440, .F. ) ;
#54354=CIRCLE ( 'NONE', #23552, 0.1418229129681522482 ) ;
#54356=DIRECTION ( 'NONE',  ( 0.000000000000000000, 0.000000000000000000, 1.000000000000000000 ) ) ;
#54367=CARTESIAN_POINT ( 'NONE',  ( -66.21217304253431735, 40.79406095866392690, -10.00000000000000000 ) ) ;
#54370=FACE_OUTER_BOUND ( 'NONE', #40140, .T. ) ;
#54374=EDGE_LOOP ( 'NONE', ( #74415, #25415, #90236, #80230 ) ) ;
#54377=DIRECTION ( 'NONE',  ( 0.8261602328994307465, -0.5634352399127678934, 0.000000000000000000 ) ) ;
#54379=ORIENTED_EDGE ( 'NONE', *, *, #80546, .T. ) ;
#54381=VERTEX_POINT ( 'NONE', #37578 ) ;
#54389=EDGE_CURVE ( 'NONE', #42173, #99081, #22395, .T. ) ;
#54390=LINE ( 'NONE', #7827, #43062 ) ;
#54391=EDGE_CURVE ( 'NONE', #16766, #34323, #92825, .T. ) ;
#54394=DIRECTION ( 'NONE',  ( 0.000000000000000000, 0.000000000000000000, 1.000000000000000000 ) ) ;
#54395=ORIENTED_EDGE ( 'NONE', *, *, #17475, .F. ) ;
#54407=VECTOR ( 'NONE', #28137, 1000.000000000000000 ) ;
#54414=DIRECTION ( 'NONE',  ( -0.9184028970038772277, -0.3956464567955659817, 0.000000000000000000 ) ) ;
#54418=CARTESIAN_POINT ( 'NONE',  ( 30.62489312496363425, 46.16797101519271962, -10.00000000000000000 ) ) ;
#54425=VECTOR ( 'NONE', #44368, 1000.000000000000227 ) ;
#54427=CARTESIAN_POINT ( 'NONE',  ( 42.45923888023187232, 122.5484010731363043, -10.00000000000000000 ) ) ;
#54429=CARTESIAN_POINT ( 'NONE',  ( -71.61465314115659453, 63.06504152958490295, 203.6502102582797420 ) ) ;
#54440=EDGE_CURVE ( 'NONE', #21181, #99967, #15781, .T. ) ;
#54441=CARTESIAN_POINT ( 'NONE',  ( 40.41628377845469089, 57.12529113016345406, -10.00000000000000000 ) ) ;
#54452=CARTESIAN_POINT ( 'NONE',  ( 30.62489312496363425, 46.16797101519271962, -10.00000000000000000 ) ) ;
#54466=VECTOR ( 'NONE', #29379, 1000.000000000000114 ) ;
#54470=ORIENTED_EDGE ( 'NONE', *, *, #67320, .T. ) ;
#54471=CARTESIAN_POINT ( 'NONE',  ( -19.16796693315586708, 34.39132293302410659, 59.99999999999999289 ) ) ;
#54473=AXIS2_PLACEMENT_3D ( 'NONE', #21752, #6053, #29853 ) ;
#54482=AXIS2_PLACEMENT_3D ( 'NONE', #75426, #21710, #52594 ) ;
#54483=EDGE_LOOP ( 'NONE', ( #73241, #64751, #44679, #1184 ) ) ;
#54493=DIRECTION ( 'NONE',  ( -1.000000000000000000, 0.000000000000000000, 0.000000000000000000 ) ) ;
#54496=AXIS2_PLACEMENT_3D ( 'NONE', #12467, #43336, #35748 ) ;
#54500=ORIENTED_EDGE ( 'NONE', *, *, #75963, .F. ) ;
#54508=CARTESIAN_POINT ( 'NONE',  ( -50.41871976035449165, 31.58591985673634639, 10.00000000000000000 ) ) ;
#54514=CARTESIAN_POINT ( 'NONE',  ( -50.36082798260553517, 30.16005589317048674, 177.5919119679930134 ) ) ;
#54520=ORIENTED_EDGE ( 'NONE', *, *, #86609, .F. ) ;
#54521=ORIENTED_EDGE ( 'NONE', *, *, #53826, .F. ) ;
#54522=LINE ( 'NONE', #55038, #85416 ) ;
#54528=CARTESIAN_POINT ( 'NONE',  ( 27.94679880624369162, 69.70277699303075281, 59.99999999999999289 ) ) ;
#54535=ORIENTED_EDGE ( 'NONE', *, *, #99403, .F. ) ;
#54544=DIRECTION ( 'NONE',  ( -0.9738769792773346312, -0.2270762630343691746, 0.000000000000000000 ) ) ;
#54547=DIRECTION ( 'NONE',  ( -0.9538480676139692305, 0.3002896333693469422, 0.000000000000000000 ) ) ;
#54561=FACE_OUTER_BOUND ( 'NONE', #70033, .T. ) ;
#54574=DIRECTION ( 'NONE',  ( -1.000000000000000000, 0.000000000000000000, 0.000000000000000000 ) ) ;
#54581=DIRECTION ( 'NONE',  ( -1.000000000000000000, 0.000000000000000000, 0.000000000000000000 ) ) ;
#54604=ORIENTED_EDGE ( 'NONE', *, *, #7786, .F. ) ;
#54605=LINE ( 'NONE', #68819, #57065 ) ;
#54615=DIRECTION ( 'NONE',  ( -0.4272584830711198545, -0.9041295198387040433, 0.000000000000000000 ) ) ;
#54618=AXIS2_PLACEMENT_3D ( 'NONE', #84164, #68403, #45107 ) ;
#54619=ORIENTED_EDGE ( 'NONE', *, *, #41038, .T. ) ;
#54620=AXIS2_PLACEMENT_3D ( 'NONE', #81850, #12424, #74240 ) ;
#54625=ADVANCED_FACE ( 'NONE', ( #41070 ), #63891, .F. ) ;
#54628=PLANE ( 'NONE',  #49727 ) ;
#54647=VERTEX_POINT ( 'NONE', #64902 ) ;
#54651=EDGE_CURVE ( 'NONE', #76712, #30963, #10794, .T. ) ;
#54654=DIRECTION ( 'NONE',  ( -0.8278489937552534483, 0.5609510170580086497, 0.000000000000000000 ) ) ;
#54655=CARTESIAN_POINT ( 'NONE',  ( -19.65312891409030271, 93.06504152958497400, -20.00000000000000355 ) ) ;
#54657=CARTESIAN_POINT ( 'NONE',  ( 32.18695666311190706, 46.02670049433632471, 177.5919119679930134 ) ) ;
#54659=EDGE_LOOP ( 'NONE', ( #1336, #95468, #84425, #51365 ) ) ;
#54683=ORIENTED_EDGE ( 'NONE', *, *, #68900, .F. ) ;
#54686=VECTOR ( 'NONE', #35522, 1000.000000000000114 ) ;
#54688=AXIS2_PLACEMENT_3D ( 'NONE', #90233, #35483, #44061 ) ;
#54705=AXIS2_PLACEMENT_3D ( 'NONE', #10338, #63021, #717 ) ;
#54716=CARTESIAN_POINT ( 'NONE',  ( 37.48526053816526371, 54.83666944042810343, -10.00000000000000000 ) ) ;
#54717=EDGE_CURVE ( 'NONE', #91687, #19465, #76495, .T. ) ;
#54722=AXIS2_PLACEMENT_3D ( 'NONE', #73355, #96683, #27251 ) ;
#54729=CARTESIAN_POINT ( 'NONE',  ( 3.854092266844447501, 28.45370138451379560, -10.00000000000000000 ) ) ;
#54730=CARTESIAN_POINT ( 'NONE',  ( -78.94662368502558536, 55.85910816071121587, 10.00000000000000000 ) ) ;
#54735=VECTOR ( 'NONE', #50588, 1000.000000000000000 ) ;
#54737=ORIENTED_EDGE ( 'NONE', *, *, #27995, .F. ) ;
#54742=ADVANCED_FACE ( 'NONE', ( #46560 ), #38963, .F. ) ;
#54743=VERTEX_POINT ( 'NONE', #60752 ) ;
#54744=CARTESIAN_POINT ( 'NONE',  ( 49.03918259513507394, 79.59780946358316100, -10.00000000000000000 ) ) ;
#54749=ORIENTED_EDGE ( 'NONE', *, *, #57118, .F. ) ;
#54750=ADVANCED_FACE ( 'NONE', ( #45566 ), #37958, .F. ) ;
#54753=VERTEX_POINT ( 'NONE', #49085 ) ;
#54765=EDGE_CURVE ( 'NONE', #50442, #77615, #93208, .T. ) ;
#54768=AXIS2_PLACEMENT_3D ( 'NONE', #59098, #90072, #20642 ) ;
#54771=VERTEX_POINT ( 'NONE', #59137 ) ;
#54772=EDGE_CURVE ( 'NONE', #41280, #79632, #65272, .T. ) ;
#54779=CARTESIAN_POINT ( 'NONE',  ( -17.81096996955940526, 76.60683456116618117, 13.45353793954188681 ) ) ;
#54784=ORIENTED_EDGE ( 'NONE', *, *, #24320, .T. ) ;
#54785=AXIS2_PLACEMENT_3D ( 'NONE', #26717, #17621, #95163 ) ;
#54797=CARTESIAN_POINT ( 'NONE',  ( 37.48526053816526371, 54.83666944042810343, -10.00000000000000000 ) ) ;
#54819=DIRECTION ( 'NONE',  ( -1.000000000000000000, 0.000000000000000000, 0.000000000000000000 ) ) ;
#54824=CARTESIAN_POINT ( 'NONE',  ( -19.58090909066553920, 93.18709903958436769, 59.99999999999999289 ) ) ;
#54827=CARTESIAN_POINT ( 'NONE',  ( 36.25628400652970384, 53.06077264917335867, -10.00000000000000000 ) ) ;
#54832=ORIENTED_EDGE ( 'NONE', *, *, #31190, .T. ) ;
#54833=EDGE_CURVE ( 'NONE', #6372, #5348, #64787, .T. ) ;
#54837=VECTOR ( 'NONE', #57308, 1000.000000000000114 ) ;
#54839=VECTOR ( 'NONE', #81284, 1000.000000000000114 ) ;
#54844=DIRECTION ( 'NONE',  ( -1.000000000000000000, 0.000000000000000000, 0.000000000000000000 ) ) ;
#54854=AXIS2_PLACEMENT_3D ( 'NONE', #69943, #560, #62336 ) ;
#54857=DIRECTION ( 'NONE',  ( -1.000000000000000000, 0.000000000000000000, 0.000000000000000000 ) ) ;
#54866=VERTEX_POINT ( 'NONE', #50561 ) ;
#54867=DIRECTION ( 'NONE',  ( -0.9538480676139692305, 0.3002896333693469422, 0.000000000000000000 ) ) ;
#54868=DIRECTION ( 'NONE',  ( -0.000000000000000000, -0.000000000000000000, -1.000000000000000000 ) ) ;
#54871=VECTOR ( 'NONE', #35178, 1000.000000000000000 ) ;
#54896=CARTESIAN_POINT ( 'NONE',  ( 9.830230629461709668, 30.95267373526312227, -10.00000000000000000 ) ) ;
#54898=CARTESIAN_POINT ( 'NONE',  ( 47.54560441532652959, 78.55524412553472757, -10.00000000000000000 ) ) ;
#54901=VERTEX_POINT ( 'NONE', #14573 ) ;
#54904=ORIENTED_EDGE ( 'NONE', *, *, #9513, .F. ) ;
#54913=AXIS2_PLACEMENT_3D ( 'NONE', #36530, #67431, #6647 ) ;
#54916=DIRECTION ( 'NONE',  ( -0.9505498757754612393, 0.3105719460338542959, 0.000000000000000000 ) ) ;
#54920=AXIS2_PLACEMENT_3D ( 'NONE', #95913, #19392, #34078 ) ;
#54934=CARTESIAN_POINT ( 'NONE',  ( -7.521556465916529710, 24.12430647450515053, -10.00000000000000000 ) ) ;
#54939=PLANE ( 'NONE',  #97213 ) ;
#54940=PLANE ( 'NONE',  #75779 ) ;
#54943=AXIS2_PLACEMENT_3D ( 'NONE', #11190, #72992, #46996 ) ;
#54945=VERTEX_POINT ( 'NONE', #21186 ) ;
#54946=ORIENTED_EDGE ( 'NONE', *, *, #24972, .F. ) ;
#54952=LINE ( 'NONE', #17459, #80618 ) ;
#54956=VERTEX_POINT ( 'NONE', #23142 ) ;
#54961=CARTESIAN_POINT ( 'NONE',  ( 48.81784752633560487, 86.82484054835779830, -10.00000000000000000 ) ) ;
#54963=CARTESIAN_POINT ( 'NONE',  ( 41.51553799054924099, 59.02985107750643579, -10.00000000000000000 ) ) ;
#54968=EDGE_CURVE ( 'NONE', #33594, #24915, #45449, .T. ) ;
#54980=AXIS2_PLACEMENT_3D ( 'NONE', #12571, #58152, #50544 ) ;
#54981=CARTESIAN_POINT ( 'NONE',  ( 49.07456115661582174, 91.13648234292965356, -10.00000000000000000 ) ) ;
#54988=CARTESIAN_POINT ( 'NONE',  ( -58.00277386063316243, 34.50477571329874138, 177.5919119679930134 ) ) ;
#55007=ORIENTED_EDGE ( 'NONE', *, *, #27411, .T. ) ;
#55015=ORIENTED_EDGE ( 'NONE', *, *, #16284, .T. ) ;
#55017=VERTEX_POINT ( 'NONE', #45936 ) ;
#55022=ORIENTED_EDGE ( 'NONE', *, *, #89571, .F. ) ;
#55029=CARTESIAN_POINT ( 'NONE',  ( 41.71240375114938814, 62.05720181600818108, 10.00000000000000000 ) ) ;
#55034=EDGE_CURVE ( 'NONE', #92904, #20754, #38344, .T. ) ;
#55035=VERTEX_POINT ( 'NONE', #53056 ) ;
#55036=LINE ( 'NONE', #70240, #3996 ) ;
#55038=CARTESIAN_POINT ( 'NONE',  ( -35.39636583819505233, 63.79609003141229095, -10.00000000000000000 ) ) ;
#55040=CARTESIAN_POINT ( 'NONE',  ( 49.09245556086621320, 93.56363653685789927, -10.00000000000000000 ) ) ;
#55042=CARTESIAN_POINT ( 'NONE',  ( -19.65312891409030271, 93.06504152958497400, 25.00000000000000000 ) ) ;
#55054=DIRECTION ( 'NONE',  ( 0.000000000000000000, -0.000000000000000000, 1.000000000000000000 ) ) ;
#55058=CARTESIAN_POINT ( 'NONE',  ( 48.17894221477870786, 74.75545800895066861, -10.00000000000000000 ) ) ;
#55067=AXIS2_PLACEMENT_3D ( 'NONE', #81168, #35006, #65906 ) ;
#55076=DIRECTION ( 'NONE',  ( -0.9979398670145503969, -0.06415622980647761597, 0.000000000000000000 ) ) ;
#55087=EDGE_CURVE ( 'NONE', #70938, #88538, #36357, .T. ) ;
#55089=EDGE_CURVE ( 'NONE', #5812, #62259, #67770, .T. ) ;
#55091=CARTESIAN_POINT ( 'NONE',  ( 27.81597692694000656, 72.50130484473876891, 59.99999999999999289 ) ) ;
#55114=ORIENTED_EDGE ( 'NONE', *, *, #88231, .T. ) ;
#55120=ORIENTED_EDGE ( 'NONE', *, *, #11455, .T. ) ;
#55124=ORIENTED_EDGE ( 'NONE', *, *, #73409, .T. ) ;
#55128=VERTEX_POINT ( 'NONE', #46957 ) ;
#55131=ORIENTED_EDGE ( 'NONE', *, *, #54249, .T. ) ;
#55133=DIRECTION ( 'NONE',  ( -1.000000000000000000, 0.000000000000000000, 0.000000000000000000 ) ) ;
#55149=ORIENTED_EDGE ( 'NONE', *, *, #81005, .T. ) ;
#55153=DIRECTION ( 'NONE',  ( 0.000000000000000000, 0.000000000000000000, 1.000000000000000000 ) ) ;
#55154=CARTESIAN_POINT ( 'NONE',  ( 25.88687446534342129, 117.6066667404749069, 59.99999999999999289 ) ) ;
#55155=DIRECTION ( 'NONE',  ( -0.7299047266382376886, 0.6835488936653759673, 0.000000000000000000 ) ) ;
#55159=VERTEX_POINT ( 'NONE', #54528 ) ;
#55172=ORIENTED_EDGE ( 'NONE', *, *, #48465, .F. ) ;
#55181=CARTESIAN_POINT ( 'NONE',  ( 7.819191540449072164, 28.68125778831126382, 10.00000000000000000 ) ) ;
#55194=EDGE_CURVE ( 'NONE', #59100, #33383, #5230, .T. ) ;
#55197=DIRECTION ( 'NONE',  ( -0.4525327339300165286, 0.8917477921037005872, 0.000000000000000000 ) ) ;
#55202=ORIENTED_EDGE ( 'NONE', *, *, #24676, .F. ) ;
#55203=EDGE_CURVE ( 'NONE', #86003, #80773, #18574, .T. ) ;
#55224=CARTESIAN_POINT ( 'NONE',  ( -19.65312891409030271, 93.06504152958497400, 177.5919119679930134 ) ) ;
#55225=CARTESIAN_POINT ( 'NONE',  ( -78.71521058394759507, 57.86724000996476747, -10.00000000000000000 ) ) ;
#55226=DIRECTION ( 'NONE',  ( -0.5634352399127678934, -0.8261602328994307465, 0.000000000000000000 ) ) ;
#55233=VERTEX_POINT ( 'NONE', #51832 ) ;
#55237=DIRECTION ( 'NONE',  ( -0.9682419296822741828, -0.2500151307524129951, 0.000000000000000000 ) ) ;
#55246=VERTEX_POINT ( 'NONE', #12851 ) ;
#55247=CARTESIAN_POINT ( 'NONE',  ( -59.87889494062799400, 37.30571521936384016, -10.00000000000000000 ) ) ;
#55260=VERTEX_POINT ( 'NONE', #89865 ) ;
#55264=EDGE_CURVE ( 'NONE', #38929, #43160, #37109, .T. ) ;
#55272=EDGE_LOOP ( 'NONE', ( #94068, #30988, #92452, #12727 ) ) ;
#55274=DIRECTION ( 'NONE',  ( -0.5696381972391160176, 0.8218955677251033043, 0.000000000000000000 ) ) ;
#55278=CARTESIAN_POINT ( 'NONE',  ( -19.65312891409030271, 93.06504152958497400, -10.00000000000000888 ) ) ;
#55279=EDGE_CURVE ( 'NONE', #11410, #86862, #66524, .T. ) ;
#55299=EDGE_LOOP ( 'NONE', ( #3338, #70083, #20904, #8950 ) ) ;
#55303=LINE ( 'NONE', #62403, #5585 ) ;
#55308=CARTESIAN_POINT ( 'NONE',  ( 38.65784837781280459, 56.65029301956751340, -10.00000000000000000 ) ) ;
#55310=VECTOR ( 'NONE', #65358, 999.9999999999998863 ) ;
#55315=EDGE_CURVE ( 'NONE', #73229, #81234, #57631, .T. ) ;
#55318=CARTESIAN_POINT ( 'NONE',  ( -61.64759997997268925, 36.73658404823907375, -10.00000000000000000 ) ) ;
#55327=EDGE_CURVE ( 'NONE', #12886, #77358, #68013, .T. ) ;
#55332=DIRECTION ( 'NONE',  ( -1.000000000000000000, 0.000000000000000000, 0.000000000000000000 ) ) ;
#55344=LINE ( 'NONE', #55831, #45766 ) ;
#55345=LINE ( 'NONE', #39636, #85490 ) ;
#55361=DIRECTION ( 'NONE',  ( -1.000000000000000000, 0.000000000000000000, 0.000000000000000000 ) ) ;
#55362=CARTESIAN_POINT ( 'NONE',  ( -52.32156893544652121, 31.15564784356141814, 177.5919119679930134 ) ) ;
#55363=CARTESIAN_POINT ( 'NONE',  ( -19.15453390681661716, 24.31945705462846163, 10.00000000000000000 ) ) ;
#55368=ORIENTED_EDGE ( 'NONE', *, *, #33051, .F. ) ;
#55379=ORIENTED_EDGE ( 'NONE', *, *, #10883, .F. ) ;
#55387=VERTEX_POINT ( 'NONE', #70503 ) ;
#55396=CARTESIAN_POINT ( 'NONE',  ( -19.65312891409030271, 93.06504152958497400, 177.5919119679930134 ) ) ;
#55398=VECTOR ( 'NONE', #12139, 1000.000000000000000 ) ;
#55399=FACE_OUTER_BOUND ( 'NONE', #77837, .T. ) ;
#55409=CARTESIAN_POINT ( 'NONE',  ( -11.40312891409031693, 78.77562236714182120, 59.99999999999999289 ) ) ;
#55410=EDGE_CURVE ( 'NONE', #40696, #28346, #4350, .T. ) ;
#55412=CARTESIAN_POINT ( 'NONE',  ( 50.32263495959776378, 94.90690751109829648, -10.00000000000000000 ) ) ;
#55413=VERTEX_POINT ( 'NONE', #33517 ) ;
#55425=ORIENTED_EDGE ( 'NONE', *, *, #75166, .T. ) ;
#55439=EDGE_LOOP ( 'NONE', ( #73479, #52416, #33478, #73154 ) ) ;
#55441=EDGE_CURVE ( 'NONE', #3474, #81396, #39892, .T. ) ;
#55452=ADVANCED_FACE ( 'NONE', ( #80156 ), #10222, .F. ) ;
#55458=ORIENTED_EDGE ( 'NONE', *, *, #28389, .F. ) ;
#55464=DIRECTION ( 'NONE',  ( 0.05364311403570637404, 0.9985601716053731369, 0.000000000000000000 ) ) ;
#55466=FACE_OUTER_BOUND ( 'NONE', #10113, .T. ) ;
#55477=CARTESIAN_POINT ( 'NONE',  ( -59.82327302696292293, 35.73826312759339174, 10.00000000000000000 ) ) ;
#55482=LINE ( 'NONE', #69702, #4864 ) ;
#55488=DIRECTION ( 'NONE',  ( 0.3984034379158949979, -0.9172102815913020235, 0.000000000000000000 ) ) ;
#55494=ORIENTED_EDGE ( 'NONE', *, *, #71138, .T. ) ;
#55498=DIRECTION ( 'NONE',  ( -0.4055404667435467125, 0.9140770918436946779, 0.000000000000000000 ) ) ;
#55500=DIRECTION ( 'NONE',  ( -0.6201213960746324583, 0.7845058662179964504, 0.000000000000000000 ) ) ;
#55502=ORIENTED_EDGE ( 'NONE', *, *, #5138, .T. ) ;
#55504=ORIENTED_EDGE ( 'NONE', *, *, #84999, .F. ) ;
#55507=CARTESIAN_POINT ( 'NONE',  ( -10.54235908185773418, 24.92402704602492847, -10.00000000000000000 ) ) ;
#55516=CARTESIAN_POINT ( 'NONE',  ( -58.11485369836745463, 56.56539583079995737, 59.99999999999999289 ) ) ;
#55526=LINE ( 'NONE', #93585, #9372 ) ;
#55535=ADVANCED_FACE ( 'NONE', ( #66404 ), #51187, .T. ) ;
#55539=LINE ( 'NONE', #32258, #81945 ) ;
#55565=CARTESIAN_POINT ( 'NONE',  ( -19.79482558122098013, 93.07102426866003952, 59.99999999999999289 ) ) ;
#55574=EDGE_CURVE ( 'NONE', #61794, #7924, #96348, .T. ) ;
#55579=CARTESIAN_POINT ( 'NONE',  ( 22.87549206224920084, 39.05096577487528720, 10.00000000000000000 ) ) ;
#55599=AXIS2_PLACEMENT_3D ( 'NONE', #73981, #43556, #4565 ) ;
#55604=AXIS2_PLACEMENT_3D ( 'NONE', #31064, #30581, #76683 ) ;
#55611=CARTESIAN_POINT ( 'NONE',  ( 7.864685750751951865, 30.05722773587472929, -10.00000000000000000 ) ) ;
#55612=ORIENTED_EDGE ( 'NONE', *, *, #91616, .F. ) ;
#55614=VECTOR ( 'NONE', #71744, 1000.000000000000114 ) ;
#55619=ORIENTED_EDGE ( 'NONE', *, *, #91858, .T. ) ;
#55626=CARTESIAN_POINT ( 'NONE',  ( 48.74043828842092552, 100.0309547576005258, -10.00000000000000000 ) ) ;
#55643=ORIENTED_EDGE ( 'NONE', *, *, #57001, .T. ) ;
#55647=DIRECTION ( 'NONE',  ( 0.1473778574936323582, 0.9890802632347824863, 0.000000000000000000 ) ) ;
#55654=VERTEX_POINT ( 'NONE', #53675 ) ;
#55658=EDGE_CURVE ( 'NONE', #79781, #98426, #83640, .T. ) ;
#55667=CARTESIAN_POINT ( 'NONE',  ( -71.07364842061382149, 47.42355933771584375, -10.00000000000000000 ) ) ;
#55672=FACE_OUTER_BOUND ( 'NONE', #89373, .T. ) ;
#55679=ORIENTED_EDGE ( 'NONE', *, *, #55946, .F. ) ;
#55680=VECTOR ( 'NONE', #19565, 1000.000000000000341 ) ;
#55691=LINE ( 'NONE', #72950, #37131 ) ;
#55702=PLANE ( 'NONE',  #10451 ) ;
#55712=EDGE_CURVE ( 'NONE', #16775, #76974, #84147, .T. ) ;
#55716=DIRECTION ( 'NONE',  ( 0.1237105541964823863, -0.9923183454821336014, 0.000000000000000000 ) ) ;
#55718=DIRECTION ( 'NONE',  ( 0.5895128895116616974, 0.8077589696806909414, 0.000000000000000000 ) ) ;
#55720=CARTESIAN_POINT ( 'NONE',  ( 49.17298586869600996, 105.8308522718264584, 10.00000000000000000 ) ) ;
#55732=CARTESIAN_POINT ( 'NONE',  ( 32.47331203838563596, 45.95596728736418868, 10.00000000000000000 ) ) ;
#55733=DIRECTION ( 'NONE',  ( 1.000000000000000000, 0.000000000000000000, 0.000000000000000000 ) ) ;
#55747=VECTOR ( 'NONE', #85766, 1000.000000000000000 ) ;
#55753=EDGE_LOOP ( 'NONE', ( #41482, #6947, #77304, #89832 ) ) ;
#55755=ADVANCED_FACE ( 'NONE', ( #30391 ), #60272, .T. ) ;
#55763=ORIENTED_EDGE ( 'NONE', *, *, #16681, .F. ) ;
#55766=LINE ( 'NONE', #64400, #37966 ) ;
#55772=ADVANCED_FACE ( 'NONE', ( #8102 ), #30891, .F. ) ;
#55775=LINE ( 'NONE', #17821, #85058 ) ;
#55776=CIRCLE ( 'NONE', #81738, 0.1418229129681591871 ) ;
#55778=LINE ( 'NONE', #86769, #44401 ) ;
#55802=LINE ( 'NONE', #23926, #35065 ) ;
#55807=VECTOR ( 'NONE', #49805, 1000.000000000000000 ) ;
#55814=AXIS2_PLACEMENT_3D ( 'NONE', #44389, #4926, #35805 ) ;
#55831=CARTESIAN_POINT ( 'NONE',  ( -19.59030177132946449, 93.19218903752455674, 59.99999999999999289 ) ) ;
#55843=ORIENTED_EDGE ( 'NONE', *, *, #83815, .F. ) ;
#55859=ORIENTED_EDGE ( 'NONE', *, *, #27783, .T. ) ;
#55860=ORIENTED_EDGE ( 'NONE', *, *, #41272, .F. ) ;
#55865=ORIENTED_EDGE ( 'NONE', *, *, #71380, .F. ) ;
#55866=CARTESIAN_POINT ( 'NONE',  ( -44.74834796241764678, 29.05375577536863929, -10.00000000000000000 ) ) ;
#55869=VERTEX_POINT ( 'NONE', #35104 ) ;
#55871=PLANE ( 'NONE',  #91876 ) ;
#55873=VECTOR ( 'NONE', #81596, 1000.000000000000000 ) ;
#55878=EDGE_CURVE ( 'NONE', #24506, #3124, #89374, .T. ) ;
#55879=CARTESIAN_POINT ( 'NONE',  ( -19.65312891409030271, 93.06504152958497400, 10.00000000000000888 ) ) ;
#55881=VERTEX_POINT ( 'NONE', #81751 ) ;
#55883=VECTOR ( 'NONE', #27750, 1000.000000000000227 ) ;
#55884=ORIENTED_EDGE ( 'NONE', *, *, #43187, .F. ) ;
#55894=ORIENTED_EDGE ( 'NONE', *, *, #99337, .F. ) ;
#55908=CARTESIAN_POINT ( 'NONE',  ( -19.65312891409030271, 93.06504152958497400, 59.99999999999999289 ) ) ;
#55909=EDGE_LOOP ( 'NONE', ( #28579, #5825, #18937, #43271 ) ) ;
#55911=CARTESIAN_POINT ( 'NONE',  ( -52.42927860546615904, 87.56549226992709123, -10.00000000000000000 ) ) ;
#55922=VECTOR ( 'NONE', #94618, 1000.000000000000000 ) ;
#55935=DIRECTION ( 'NONE',  ( -0.000000000000000000, -0.000000000000000000, -1.000000000000000000 ) ) ;
#55936=ORIENTED_EDGE ( 'NONE', *, *, #89456, .T. ) ;
#55943=VECTOR ( 'NONE', #39841, 1000.000000000000000 ) ;
#55946=EDGE_CURVE ( 'NONE', #98647, #59479, #8201, .T. ) ;
#55960=CARTESIAN_POINT ( 'NONE',  ( -52.31886624268647523, 30.86069821571189919, -10.00000000000000000 ) ) ;
#55969=CARTESIAN_POINT ( 'NONE',  ( 43.33680334696484948, 124.1889737374328462, -10.00000000000000000 ) ) ;
#55978=CARTESIAN_POINT ( 'NONE',  ( -19.65312891409030271, 93.06504152958497400, -10.00000000000000888 ) ) ;
#55986=CARTESIAN_POINT ( 'NONE',  ( -41.22173478680166880, 38.49732326316120634, 59.99999999999999289 ) ) ;
#55993=FACE_OUTER_BOUND ( 'NONE', #19589, .T. ) ;
#55996=VECTOR ( 'NONE', #58053, 1000.000000000000000 ) ;
#55999=EDGE_CURVE ( 'NONE', #12449, #42468, #78614, .T. ) ;
#56000=ORIENTED_EDGE ( 'NONE', *, *, #20158, .F. ) ;
#56002=VECTOR ( 'NONE', #66632, 1000.000000000000000 ) ;
#56012=DIRECTION ( 'NONE',  ( -0.03004293549037828290, -0.9995486091367047354, 0.000000000000000000 ) ) ;
#56022=ADVANCED_FACE ( 'NONE', ( #95850 ), #41585, .F. ) ;
#56025=AXIS2_PLACEMENT_3D ( 'NONE', #94828, #49207, #72008 ) ;
#56033=VECTOR ( 'NONE', #37033, 1000.000000000000000 ) ;
#56035=CARTESIAN_POINT ( 'NONE',  ( -11.38800805193611154, 34.97435025094601713, 59.99999999999999289 ) ) ;
#56039=ORIENTED_EDGE ( 'NONE', *, *, #37565, .T. ) ;
#56056=DIRECTION ( 'NONE',  ( 1.000000000000000000, -1.784287003861858500E-15, 0.000000000000000000 ) ) ;
#56068=AXIS2_PLACEMENT_3D ( 'NONE', #2994, #72384, #81015 ) ;
#56075=DIRECTION ( 'NONE',  ( 0.7548338719222560389, -0.6559160203858837024, 0.000000000000000000 ) ) ;
#56076=VECTOR ( 'NONE', #87646, 1000.000000000000227 ) ;
#56077=CARTESIAN_POINT ( 'NONE',  ( -54.21831688459418785, 33.63902229265146104, -10.00000000000000000 ) ) ;
#56088=LINE ( 'NONE', #58103, #3718 ) ;
#56089=DIRECTION ( 'NONE',  ( -0.8769651246872975925, 0.4805540241036304061, 0.000000000000000000 ) ) ;
#56091=AXIS2_PLACEMENT_3D ( 'NONE', #36757, #61547, #30666 ) ;
#56098=DIRECTION ( 'NONE',  ( -0.9991767892008870389, -0.04056776950001317328, 0.000000000000000000 ) ) ;
#56104=AXIS2_PLACEMENT_3D ( 'NONE', #82498, #36327, #60110 ) ;
#56105=EDGE_CURVE ( 'NONE', #55035, #8715, #3135, .T. ) ;
#56109=LINE ( 'NONE', #39900, #31242 ) ;
#56115=CARTESIAN_POINT ( 'NONE',  ( 39.20103187901341357, 54.69033006916458106, 10.00000000000000000 ) ) ;
#56118=DIRECTION ( 'NONE',  ( 0.9862134920484671996, 0.1654779384134575648, 0.000000000000000000 ) ) ;
#56120=DIRECTION ( 'NONE',  ( -0.9997716407803077798, 0.02136975178731310987, 0.000000000000000000 ) ) ;
#56122=LINE ( 'NONE', #47039, #19207 ) ;
#56123=ORIENTED_EDGE ( 'NONE', *, *, #7869, .F. ) ;
#56126=LINE ( 'NONE', #63750, #99601 ) ;
#56127=PLANE ( 'NONE',  #98354 ) ;
#56132=ADVANCED_FACE ( 'NONE', ( #19330 ), #50192, .F. ) ;
#56141=PLANE ( 'NONE',  #90415 ) ;
#56143=ORIENTED_EDGE ( 'NONE', *, *, #5384, .T. ) ;
#56147=VERTEX_POINT ( 'NONE', #44067 ) ;
#56153=CARTESIAN_POINT ( 'NONE',  ( -63.30067564770008914, 39.94154026010144065, -10.00000000000000000 ) ) ;
#56168=FACE_OUTER_BOUND ( 'NONE', #18647, .T. ) ;
#56169=EDGE_LOOP ( 'NONE', ( #38559, #27350, #33092, #52997 ) ) ;
#56170=AXIS2_PLACEMENT_3D ( 'NONE', #95499, #12342, #18452 ) ;
#56177=CARTESIAN_POINT ( 'NONE',  ( 19.12011368430507829, 34.47266676343468106, -10.00000000000000000 ) ) ;
#56178=EDGE_CURVE ( 'NONE', #36317, #61038, #20808, .T. ) ;
#56179=DIRECTION ( 'NONE',  ( 0.000000000000000000, 0.000000000000000000, 1.000000000000000000 ) ) ;
#56189=LINE ( 'NONE', #77526, #47794 ) ;
#56199=CARTESIAN_POINT ( 'NONE',  ( 27.80861752939100029, 41.25950758903265836, -10.00000000000000000 ) ) ;
#56200=CARTESIAN_POINT ( 'NONE',  ( -60.01996847620949183, 50.48172571078520576, 59.99999999999999289 ) ) ;
#56219=DIRECTION ( 'NONE',  ( -0.3177184104407422272, 0.9481851146622204407, 0.000000000000000000 ) ) ;
#56223=VECTOR ( 'NONE', #11875, 1000.000000000000114 ) ;
#56236=VECTOR ( 'NONE', #29734, 1000.000000000000000 ) ;
#56245=ORIENTED_EDGE ( 'NONE', *, *, #26269, .T. ) ;
#56250=ORIENTED_EDGE ( 'NONE', *, *, #47540, .T. ) ;
#56255=VERTEX_POINT ( 'NONE', #24154 ) ;
#56257=VECTOR ( 'NONE', #60572, 1000.000000000000114 ) ;
#56258=EDGE_CURVE ( 'NONE', #33736, #213, #94588, .T. ) ;
#56269=ORIENTED_EDGE ( 'NONE', *, *, #44500, .T. ) ;
#56271=ORIENTED_EDGE ( 'NONE', *, *, #54651, .F. ) ;
#56289=DIRECTION ( 'NONE',  ( 1.000000000000000000, 0.000000000000000000, 0.000000000000000000 ) ) ;
#56302=LINE ( 'NONE', #64923, #80537 ) ;
#56318=DIRECTION ( 'NONE',  ( -0.5346708562974005208, -0.8450603975019800318, 0.000000000000000000 ) ) ;
#56327=DIRECTION ( 'NONE',  ( 0.000000000000000000, -0.000000000000000000, 1.000000000000000000 ) ) ;
#56329=VECTOR ( 'NONE', #19368, 1000.000000000000000 ) ;
#56332=ORIENTED_EDGE ( 'NONE', *, *, #56105, .T. ) ;
#56341=CARTESIAN_POINT ( 'NONE',  ( 27.76992210170819675, 43.29297894285233639, 10.00000000000000000 ) ) ;
#56345=CYLINDRICAL_SURFACE ( 'NONE', #51686, 70.00000000000002842 ) ;
#56352=VECTOR ( 'NONE', #58411, 1000.000000000000114 ) ;
#56364=ORIENTED_EDGE ( 'NONE', *, *, #55946, .T. ) ;
#56366=LINE ( 'NONE', #47267, #87631 ) ;
#56384=ORIENTED_EDGE ( 'NONE', *, *, #30739, .T. ) ;
#56387=VERTEX_POINT ( 'NONE', #96601 ) ;
#56390=VERTEX_POINT ( 'NONE', #82410 ) ;
#56396=ORIENTED_EDGE ( 'NONE', *, *, #55087, .T. ) ;
#56397=DIRECTION ( 'NONE',  ( 0.7694697644498922351, -0.6386832404231594928, 0.000000000000000000 ) ) ;
#56406=VERTEX_POINT ( 'NONE', #2882 ) ;
#56418=VERTEX_POINT ( 'NONE', #65644 ) ;
#56426=ORIENTED_EDGE ( 'NONE', *, *, #18384, .F. ) ;
#56431=EDGE_CURVE ( 'NONE', #77218, #16945, #1091, .T. ) ;
#56435=CARTESIAN_POINT ( 'NONE',  ( -51.75017079496728201, 30.85748650210272359, 177.5919119679930134 ) ) ;
#56443=VECTOR ( 'NONE', #1789, 1000.000000000000114 ) ;
#56449=AXIS2_PLACEMENT_3D ( 'NONE', #22561, #75788, #29177 ) ;
#56456=DIRECTION ( 'NONE',  ( -0.9923183454821322691, -0.1237105541964931832, 0.000000000000000000 ) ) ;
#56457=CIRCLE ( 'NONE', #83986, 50.00000000000000711 ) ;
#56465=AXIS2_PLACEMENT_3D ( 'NONE', #42255, #87458, #71700 ) ;
#56477=ORIENTED_EDGE ( 'NONE', *, *, #99337, .T. ) ;
#56488=ORIENTED_EDGE ( 'NONE', *, *, #33829, .T. ) ;
#56492=DIRECTION ( 'NONE',  ( 0.000000000000000000, 0.000000000000000000, 1.000000000000000000 ) ) ;
#56504=CARTESIAN_POINT ( 'NONE',  ( -6.887318171848119341, 24.23892674679880699, 10.00000000000000000 ) ) ;
#56507=ORIENTED_EDGE ( 'NONE', *, *, #89366, .F. ) ;
#56510=DIRECTION ( 'NONE',  ( 0.000000000000000000, 0.000000000000000000, 1.000000000000000000 ) ) ;
#56511=VERTEX_POINT ( 'NONE', #51949 ) ;
#56516=VECTOR ( 'NONE', #99573, 1000.000000000000000 ) ;
#56534=CARTESIAN_POINT ( 'NONE',  ( -71.07364842061382149, 47.42355933771584375, 10.00000000000000000 ) ) ;
#56536=LINE ( 'NONE', #18057, #58234 ) ;
#56541=ORIENTED_EDGE ( 'NONE', *, *, #88562, .F. ) ;
#56550=CARTESIAN_POINT ( 'NONE',  ( -77.74869931532474254, 54.01501336371526918, -10.00000000000000000 ) ) ;
#56554=CARTESIAN_POINT ( 'NONE',  ( 6.335516158286851329, 48.33503367028950493, 59.99999999999999289 ) ) ;
#56556=ORIENTED_EDGE ( 'NONE', *, *, #63291, .T. ) ;
#56560=PLANE ( 'NONE',  #30550 ) ;
#56568=PLANE ( 'NONE',  #26837 ) ;
#56569=VERTEX_POINT ( 'NONE', #16923 ) ;
#56571=DIRECTION ( 'NONE',  ( -0.7440200784635719877, -0.6681572590663519273, 0.000000000000000000 ) ) ;
#56572=EDGE_CURVE ( 'NONE', #98426, #28484, #85902, .T. ) ;
#56574=EDGE_CURVE ( 'NONE', #11342, #63646, #70115, .T. ) ;
#56582=CARTESIAN_POINT ( 'NONE',  ( -19.65312891409030271, 93.06504152958497400, -10.00000000000000888 ) ) ;
#56584=FACE_OUTER_BOUND ( 'NONE', #44065, .T. ) ;
#56585=PLANE ( 'NONE',  #37670 ) ;
#56586=LINE ( 'NONE', #87574, #42117 ) ;
#56588=CARTESIAN_POINT ( 'NONE',  ( 42.65610334793076674, 64.00004027534475881, -10.00000000000000000 ) ) ;
#56591=EDGE_CURVE ( 'NONE', #56255, #66534, #46476, .T. ) ;
#56592=CARTESIAN_POINT ( 'NONE',  ( -66.35579582111500940, 58.76611569233396182, 59.99999999999999289 ) ) ;
#56596=VECTOR ( 'NONE', #10639, 1000.000000000000000 ) ;
#56604=ADVANCED_FACE ( 'NONE', ( #40208 ), #48340, .F. ) ;
#56611=CARTESIAN_POINT ( 'NONE',  ( -32.30932376655839988, 25.48519649537502119, 10.00000000000000000 ) ) ;
#56621=ORIENTED_EDGE ( 'NONE', *, *, #19310, .F. ) ;
#56634=CYLINDRICAL_SURFACE ( 'NONE', #95267, 70.00000000000002842 ) ;
#56644=FACE_OUTER_BOUND ( 'NONE', #19831, .T. ) ;
#56648=LINE ( 'NONE', #95201, #24963 ) ;
#56660=ORIENTED_EDGE ( 'NONE', *, *, #39316, .F. ) ;
#56664=ORIENTED_EDGE ( 'NONE', *, *, #82172, .F. ) ;
#56669=DIRECTION ( 'NONE',  ( -0.000000000000000000, 0.000000000000000000, -1.000000000000000000 ) ) ;
#56673=ORIENTED_EDGE ( 'NONE', *, *, #94253, .T. ) ;
#56674=VECTOR ( 'NONE', #83141, 1000.000000000000227 ) ;
#56675=ORIENTED_EDGE ( 'NONE', *, *, #14115, .F. ) ;
#56691=ADVANCED_FACE ( 'NONE', ( #57420 ), #65527, .T. ) ;
#56711=CARTESIAN_POINT ( 'NONE',  ( 30.34687108590970794, 93.06504152958497400, -25.00000000000000000 ) ) ;
#56716=EDGE_CURVE ( 'NONE', #73949, #84464, #11850, .T. ) ;
#56722=CARTESIAN_POINT ( 'NONE',  ( -42.93703707550763937, 69.35047530159833684, -10.00000000000000000 ) ) ;
#56733=FACE_OUTER_BOUND ( 'NONE', #61787, .T. ) ;
#56734=AXIS2_PLACEMENT_3D ( 'NONE', #58375, #89351, #19904 ) ;
#56741=CARTESIAN_POINT ( 'NONE',  ( -13.57166651430987514, 85.17168110439646966, 14.94339635218015694 ) ) ;
#56743=FACE_OUTER_BOUND ( 'NONE', #23496, .T. ) ;
#56747=DIRECTION ( 'NONE',  ( -0.8916269620120498285, 0.4527707594502571875, 0.000000000000000000 ) ) ;
#56755=CARTESIAN_POINT ( 'NONE',  ( 44.85937643310610667, 116.8208962945185050, -10.00000000000000000 ) ) ;
#56760=LINE ( 'NONE', #3101, #71174 ) ;
#56761=CARTESIAN_POINT ( 'NONE',  ( 48.05312180239142350, 111.8345470171556428, -10.00000000000000000 ) ) ;
#56764=DIRECTION ( 'NONE',  ( -0.8770933717188628131, -0.4803199113995136327, 0.000000000000000000 ) ) ;
#56765=CARTESIAN_POINT ( 'NONE',  ( -29.91485116994501325, 25.08783183303773967, -10.00000000000000000 ) ) ;
#56787=ORIENTED_EDGE ( 'NONE', *, *, #48102, .T. ) ;
#56790=DIRECTION ( 'NONE',  ( 0.000000000000000000, -0.000000000000000000, -1.000000000000000000 ) ) ;
#56795=CARTESIAN_POINT ( 'NONE',  ( 44.44844410339184293, 68.22168590943847732, -10.00000000000000000 ) ) ;
#56804=EDGE_LOOP ( 'NONE', ( #70987, #47280, #92112, #74341 ) ) ;
#56806=DIRECTION ( 'NONE',  ( 0.9505498757754579087, -0.3105719460338643989, 0.000000000000000000 ) ) ;
#56817=CARTESIAN_POINT ( 'NONE',  ( -56.14442822474984496, 33.32908021129815523, 10.00000000000000000 ) ) ;
#56843=FACE_OUTER_BOUND ( 'NONE', #72649, .T. ) ;
#56844=CARTESIAN_POINT ( 'NONE',  ( 18.86588705934989108, 49.77739081350934924, 59.99999999999999289 ) ) ;
#56855=CARTESIAN_POINT ( 'NONE',  ( 24.35067441160642687, 40.23626134430271861, -10.00000000000000000 ) ) ;
#56877=VECTOR ( 'NONE', #44636, 1000.000000000000114 ) ;
#56879=ORIENTED_EDGE ( 'NONE', *, *, #75038, .F. ) ;
#56880=VERTEX_POINT ( 'NONE', #22905 ) ;
#56881=DIRECTION ( 'NONE',  ( 1.000000000000000000, 0.000000000000000000, 0.000000000000000000 ) ) ;
#56885=LINE ( 'NONE', #1716, #82417 ) ;
#56890=ORIENTED_EDGE ( 'NONE', *, *, #50555, .T. ) ;
#56893=CARTESIAN_POINT ( 'NONE',  ( 13.75631770279071020, 31.55236904046464375, 10.00000000000000000 ) ) ;
#56896=LINE ( 'NONE', #1731, #13150 ) ;
#56898=ORIENTED_EDGE ( 'NONE', *, *, #47829, .T. ) ;
#56903=ORIENTED_EDGE ( 'NONE', *, *, #15929, .T. ) ;
#56912=CARTESIAN_POINT ( 'NONE',  ( 26.18314342202568668, 41.82794442100486521, -10.00000000000000000 ) ) ;
#56922=DIRECTION ( 'NONE',  ( 0.9598361373656965068, -0.2805612043866717586, 0.000000000000000000 ) ) ;
#56923=EDGE_CURVE ( 'NONE', #9815, #45024, #17345, .T. ) ;
#56926=EDGE_CURVE ( 'NONE', #35722, #74770, #36799, .T. ) ;
#56928=VERTEX_POINT ( 'NONE', #77108 ) ;
#56933=EDGE_CURVE ( 'NONE', #2112, #71283, #56302, .T. ) ;
#56941=LINE ( 'NONE', #11386, #18743 ) ;
#56942=ORIENTED_EDGE ( 'NONE', *, *, #27729, .T. ) ;
#56949=CARTESIAN_POINT ( 'NONE',  ( 5.871984111234073822, 29.22396284167519198, -10.00000000000000000 ) ) ;
#56950=CARTESIAN_POINT ( 'NONE',  ( 48.58227110419247907, 77.44677708231240842, -10.00000000000000000 ) ) ;
#56957=CYLINDRICAL_SURFACE ( 'NONE', #56465, 70.00000000000002842 ) ;
#56966=VERTEX_POINT ( 'NONE', #74026 ) ;
#56969=PLANE ( 'NONE',  #28813 ) ;
#56973=CARTESIAN_POINT ( 'NONE',  ( -50.66096862766640641, 31.69950886434491721, -10.00000000000000000 ) ) ;
#56980=ADVANCED_FACE ( 'NONE', ( #33522 ), #34510, .F. ) ;
#56995=ORIENTED_EDGE ( 'NONE', *, *, #47659, .T. ) ;
#56998=FACE_OUTER_BOUND ( 'NONE', #88594, .T. ) ;
#57001=EDGE_CURVE ( 'NONE', #59397, #9269, #1161, .T. ) ;
#57006=DIRECTION ( 'NONE',  ( -0.7352104281592222179, 0.6778389383370750920, 0.000000000000000000 ) ) ;
#57014=ORIENTED_EDGE ( 'NONE', *, *, #90829, .F. ) ;
#57017=VERTEX_POINT ( 'NONE', #65411 ) ;
#57037=EDGE_CURVE ( 'NONE', #6693, #20542, #4107, .T. ) ;
#57039=DIRECTION ( 'NONE',  ( -0.000000000000000000, -0.000000000000000000, 1.000000000000000000 ) ) ;
#57043=DIRECTION ( 'NONE',  ( 1.000000000000000000, 0.000000000000000000, 0.000000000000000000 ) ) ;
#57046=CARTESIAN_POINT ( 'NONE',  ( -19.65312891409030271, 93.06504152958497400, 177.5919119679930134 ) ) ;
#57047=LINE ( 'NONE', #1870, #95057 ) ;
#57051=ORIENTED_EDGE ( 'NONE', *, *, #80736, .T. ) ;
#57062=ORIENTED_EDGE ( 'NONE', *, *, #41945, .F. ) ;
#57064=DIRECTION ( 'NONE',  ( 1.000000000000000000, 0.000000000000000000, -0.000000000000000000 ) ) ;
#57065=VECTOR ( 'NONE', #69822, 1000.000000000000114 ) ;
#57066=PLANE ( 'NONE',  #67801 ) ;
#57067=CARTESIAN_POINT ( 'NONE',  ( -48.34856483818852979, 28.93234566034054822, 10.00000000000000000 ) ) ;
#57076=PLANE ( 'NONE',  #2751 ) ;
#57094=DIRECTION ( 'NONE',  ( -0.9292718480896766664, -0.3693965786901617920, 0.000000000000000000 ) ) ;
#57106=EDGE_CURVE ( 'NONE', #100024, #67772, #25448, .T. ) ;
#57113=DIRECTION ( 'NONE',  ( 0.000000000000000000, 0.000000000000000000, 1.000000000000000000 ) ) ;
#57115=ORIENTED_EDGE ( 'NONE', *, *, #25022, .F. ) ;
#57118=EDGE_CURVE ( 'NONE', #97948, #96856, #42591, .T. ) ;
#57121=ORIENTED_EDGE ( 'NONE', *, *, #73874, .F. ) ;
#57126=ORIENTED_EDGE ( 'NONE', *, *, #74547, .T. ) ;
#57150=DIRECTION ( 'NONE',  ( -0.000000000000000000, -0.000000000000000000, -1.000000000000000000 ) ) ;
#57153=ORIENTED_EDGE ( 'NONE', *, *, #24101, .F. ) ;
#57156=CARTESIAN_POINT ( 'NONE',  ( -77.42978507651396569, 55.80833764325424085, 10.00000000000000000 ) ) ;
#57164=CARTESIAN_POINT ( 'NONE',  ( -6.281727404287059890, 25.63055774385195917, -10.00000000000000000 ) ) ;
#57165=VERTEX_POINT ( 'NONE', #38979 ) ;
#57168=DIRECTION ( 'NONE',  ( 1.000000000000000000, -2.478176394252581023E-14, 0.000000000000000000 ) ) ;
#57179=EDGE_CURVE ( 'NONE', #29884, #54945, #39966, .T. ) ;
#57182=CARTESIAN_POINT ( 'NONE',  ( -48.47243291925848752, 30.64988553008148031, -10.00000000000000000 ) ) ;
#57184=CARTESIAN_POINT ( 'NONE',  ( -19.65312891409030271, 93.06504152958497400, 59.99999999999999289 ) ) ;
#57192=VECTOR ( 'NONE', #89566, 1000.000000000000114 ) ;
#57203=CIRCLE ( 'NONE', #28213, 70.00000000000001421 ) ;
#57205=VECTOR ( 'NONE', #97515, 1000.000000000000000 ) ;
#57207=ORIENTED_EDGE ( 'NONE', *, *, #9039, .T. ) ;
#57213=EDGE_CURVE ( 'NONE', #86151, #72984, #85654, .T. ) ;
#57217=CARTESIAN_POINT ( 'NONE',  ( 32.30839531297598910, 123.0650415295850593, 40.00000000000000000 ) ) ;
#57219=CARTESIAN_POINT ( 'NONE',  ( -19.65312891409030271, 93.06504152958497400, 177.5919119679930134 ) ) ;
#57221=DIRECTION ( 'NONE',  ( -0.000000000000000000, 0.000000000000000000, 1.000000000000000000 ) ) ;
#57226=DIRECTION ( 'NONE',  ( -0.000000000000000000, 0.000000000000000000, 1.000000000000000000 ) ) ;
#57227=CARTESIAN_POINT ( 'NONE',  ( -50.66096862766640641, 31.69950886434491721, -10.00000000000000000 ) ) ;
#57230=VERTEX_POINT ( 'NONE', #68881 ) ;
#57231=CARTESIAN_POINT ( 'NONE',  ( -15.54040582425010086, 84.12771141922644347, 14.97918986780710959 ) ) ;
#57247=CARTESIAN_POINT ( 'NONE',  ( 43.24043327773039636, 120.8247932685368227, 10.00000000000000000 ) ) ;
#57249=ORIENTED_EDGE ( 'NONE', *, *, #68501, .T. ) ;
#57256=VERTEX_POINT ( 'NONE', #52566 ) ;
#57268=DIRECTION ( 'NONE',  ( -0.6602847420308683990, -0.7510153523339117010, 0.000000000000000000 ) ) ;
#57274=FACE_BOUND ( 'NONE', #38063, .T. ) ;
#57288=DIRECTION ( 'NONE',  ( 0.000000000000000000, 0.000000000000000000, 1.000000000000000000 ) ) ;
#57292=ADVANCED_FACE ( 'NONE', ( #5489 ), #98709, .F. ) ;
#57307=CARTESIAN_POINT ( 'NONE',  ( -29.91485116994501681, 25.08783183303773257, -10.00000000000000000 ) ) ;
#57308=DIRECTION ( 'NONE',  ( 0.2471055264905481497, -0.9689885751534065284, 0.000000000000000000 ) ) ;
#57311=VERTEX_POINT ( 'NONE', #85531 ) ;
#57314=CARTESIAN_POINT ( 'NONE',  ( 25.34687108590969729, 93.06504152958497400, -45.00000000000001421 ) ) ;
#57339=LINE ( 'NONE', #9773, #59396 ) ;
#57359=EDGE_CURVE ( 'NONE', #60221, #23598, #77894, .T. ) ;
#57361=DIRECTION ( 'NONE',  ( 0.08498217737243618508, 0.9963824715083258177, 0.000000000000000000 ) ) ;
#57363=PLANE ( 'NONE',  #73113 ) ;
#57373=EDGE_CURVE ( 'NONE', #30767, #52870, #82128, .T. ) ;
#57377=LINE ( 'NONE', #88351, #2463 ) ;
#57380=EDGE_LOOP ( 'NONE', ( #95777, #80384, #95710, #10435 ) ) ;
#57383=CARTESIAN_POINT ( 'NONE',  ( 1.233819684896646951, 25.98176417558038764, 10.00000000000000000 ) ) ;
#57385=ORIENTED_EDGE ( 'NONE', *, *, #80492, .F. ) ;
#57388=EDGE_LOOP ( 'NONE', ( #58995, #11321, #11170, #8935 ) ) ;
#57396=CARTESIAN_POINT ( 'NONE',  ( 50.34596055286377947, 92.70800680107760172, 177.5919119679930134 ) ) ;
#57420=FACE_OUTER_BOUND ( 'NONE', #87612, .T. ) ;
#57423=CARTESIAN_POINT ( 'NONE',  ( -19.65312891409030271, 93.06504152958497400, 25.00000000000000000 ) ) ;
#57427=ORIENTED_EDGE ( 'NONE', *, *, #15768, .F. ) ;
#57429=DIRECTION ( 'NONE',  ( -0.1654779384134575371, 0.9862134920484671996, 0.000000000000000000 ) ) ;
#57442=ORIENTED_EDGE ( 'NONE', *, *, #27387, .T. ) ;
#57459=CARTESIAN_POINT ( 'NONE',  ( 42.33744422746375591, 122.7866300363639169, -10.00000000000000000 ) ) ;
#57476=VERTEX_POINT ( 'NONE', #27373 ) ;
#57489=VECTOR ( 'NONE', #2097, 1000.000000000000000 ) ;
#57490=DIRECTION ( 'NONE',  ( -1.000000000000000000, 0.000000000000000000, 0.000000000000000000 ) ) ;
#57504=LINE ( 'NONE', #82856, #16031 ) ;
#57506=ORIENTED_EDGE ( 'NONE', *, *, #79300, .F. ) ;
#57507=CARTESIAN_POINT ( 'NONE',  ( -21.58168810074490551, 24.33735145887882112, 10.00000000000000000 ) ) ;
#57508=LINE ( 'NONE', #50410, #68567 ) ;
#57517=DIRECTION ( 'NONE',  ( -0.9628097264997621529, 0.2701803667135219689, 0.000000000000000000 ) ) ;
#57519=CYLINDRICAL_SURFACE ( 'NONE', #93510, 70.00000000000002842 ) ;
#57523=ORIENTED_EDGE ( 'NONE', *, *, #78238, .T. ) ;
#57530=CARTESIAN_POINT ( 'NONE',  ( 37.33196394253075567, 103.5643028465244555, 59.99999999999999289 ) ) ;
#57534=VERTEX_POINT ( 'NONE', #73482 ) ;
#57535=VECTOR ( 'NONE', #35985, 1000.000000000000114 ) ;
#57544=VECTOR ( 'NONE', #27898, 1000.000000000000000 ) ;
#57548=VERTEX_POINT ( 'NONE', #35955 ) ;
#57553=DIRECTION ( 'NONE',  ( 0.000000000000000000, 0.000000000000000000, 1.000000000000000000 ) ) ;
#57566=CARTESIAN_POINT ( 'NONE',  ( 25.98835327777827686, 41.64452202306098627, 10.00000000000000000 ) ) ;
#57570=CARTESIAN_POINT ( 'NONE',  ( -47.71918240028242764, 48.07787485988725251, 59.99999999999999289 ) ) ;
#57587=DIRECTION ( 'NONE',  ( -0.000000000000000000, 0.000000000000000000, -1.000000000000000000 ) ) ;
#57588=FACE_OUTER_BOUND ( 'NONE', #69860, .T. ) ;
#57596=CARTESIAN_POINT ( 'NONE',  ( -61.39381520214497812, 38.43978098112751951, -10.00000000000000000 ) ) ;
#57599=PLANE ( 'NONE',  #59625 ) ;
#57601=ORIENTED_EDGE ( 'NONE', *, *, #90760, .T. ) ;
#57608=AXIS2_PLACEMENT_3D ( 'NONE', #50805, #51295, #12329 ) ;
#57610=CARTESIAN_POINT ( 'NONE',  ( -48.71813016832984289, 30.75580926756359901, -10.00000000000000000 ) ) ;
#57611=CARTESIAN_POINT ( 'NONE',  ( 32.30839531297598910, 123.0650415295850593, -10.00000000000000888 ) ) ;
#57621=EDGE_CURVE ( 'NONE', #566, #42468, #38378, .T. ) ;
#57628=DIRECTION ( 'NONE',  ( -0.000000000000000000, -0.000000000000000000, -1.000000000000000000 ) ) ;
#57629=VERTEX_POINT ( 'NONE', #76948 ) ;
#57631=CIRCLE ( 'NONE', #9113, 70.00000000000001421 ) ;
#57632=DIRECTION ( 'NONE',  ( -0.8868092729070087277, -0.4621356007560363244, 0.000000000000000000 ) ) ;
#57636=ORIENTED_EDGE ( 'NONE', *, *, #95305, .F. ) ;
#57637=VERTEX_POINT ( 'NONE', #90718 ) ;
#57640=CARTESIAN_POINT ( 'NONE',  ( -38.61298035630893111, 26.97617139035147460, 10.00000000000000000 ) ) ;
#57643=CARTESIAN_POINT ( 'NONE',  ( -16.99542894172669349, 24.36904009834038476, -10.00000000000000000 ) ) ;
#57647=CARTESIAN_POINT ( 'NONE',  ( -11.52846477932265756, 34.95471236983288321, 59.99999999999999289 ) ) ;
#57650=CARTESIAN_POINT ( 'NONE',  ( -19.65312891409030271, 93.06504152958497400, 59.99999999999999289 ) ) ;
#57661=ORIENTED_EDGE ( 'NONE', *, *, #14043, .T. ) ;
#57663=LINE ( 'NONE', #73391, #9122 ) ;
#57668=VECTOR ( 'NONE', #5492, 1000.000000000000000 ) ;
#57670=CARTESIAN_POINT ( 'NONE',  ( 5.181765596169280563, 27.61866642244642733, 10.00000000000000000 ) ) ;
#57674=PLANE ( 'NONE',  #78775 ) ;
#57681=VECTOR ( 'NONE', #44323, 1000.000000000000227 ) ;
#57683=EDGE_CURVE ( 'NONE', #76974, #79042, #79504, .T. ) ;
#57685=DIRECTION ( 'NONE',  ( -1.000000000000000000, 0.000000000000000000, 0.000000000000000000 ) ) ;
#57691=EDGE_CURVE ( 'NONE', #62885, #2192, #4412, .T. ) ;
#57705=ORIENTED_EDGE ( 'NONE', *, *, #20140, .F. ) ;
#57710=LINE ( 'NONE', #18738, #89525 ) ;
#57717=ADVANCED_FACE ( 'NONE', ( #17665 ), #961, .T. ) ;
#57718=EDGE_CURVE ( 'NONE', #77450, #42396, #63758, .T. ) ;
#57725=VERTEX_POINT ( 'NONE', #25776 ) ;
#57726=CARTESIAN_POINT ( 'NONE',  ( -5.084612219170204561, 81.16070385630965234, 13.43819141829553665 ) ) ;
#57733=CARTESIAN_POINT ( 'NONE',  ( 0.4893710859096792598, 78.77562236714182120, 52.49999999999999289 ) ) ;
#57737=VECTOR ( 'NONE', #56790, 1000.000000000000000 ) ;
#57739=ORIENTED_EDGE ( 'NONE', *, *, #2985, .F. ) ;
#57740=AXIS2_PLACEMENT_3D ( 'NONE', #30474, #22376, #60852 ) ;
#57745=EDGE_CURVE ( 'NONE', #23843, #54771, #67535, .T. ) ;
#57747=ORIENTED_EDGE ( 'NONE', *, *, #19232, .T. ) ;
#57750=LINE ( 'NONE', #79615, #12970 ) ;
#57751=DIRECTION ( 'NONE',  ( -0.06142469166374902451, -0.9981117208278906805, 0.000000000000000000 ) ) ;
#57752=EDGE_LOOP ( 'NONE', ( #63037, #85883, #66806, #3730 ) ) ;
#57759=DIRECTION ( 'NONE',  ( -1.000000000000000000, 0.000000000000000000, 0.000000000000000000 ) ) ;
#57771=ORIENTED_EDGE ( 'NONE', *, *, #87641, .F. ) ;
#57773=FACE_BOUND ( 'NONE', #23752, .T. ) ;
#57776=LINE ( 'NONE', #51173, #35219 ) ;
#57782=AXIS2_PLACEMENT_3D ( 'NONE', #16352, #47246, #78166 ) ;
#57799=DIRECTION ( 'NONE',  ( -0.000000000000000000, -0.000000000000000000, 1.000000000000000000 ) ) ;
#57800=EDGE_CURVE ( 'NONE', #62226, #57476, #49550, .T. ) ;
#57801=LINE ( 'NONE', #89757, #61910 ) ;
#57802=CARTESIAN_POINT ( 'NONE',  ( 17.00529913897481293, 33.43149683636511327, -10.00000000000000000 ) ) ;
#57808=DIRECTION ( 'NONE',  ( -0.3666034970181814012, 0.9303772761487891785, 0.000000000000000000 ) ) ;
#57811=PLANE ( 'NONE',  #85548 ) ;
#57815=AXIS2_PLACEMENT_3D ( 'NONE', #44380, #98621, #13994 ) ;
#57817=LINE ( 'NONE', #26935, #12382 ) ;
#57822=DIRECTION ( 'NONE',  ( 0.1473778574936323582, 0.9890802632347824863, 0.000000000000000000 ) ) ;
#57836=CARTESIAN_POINT ( 'NONE',  ( -69.40242143070358338, 43.82067236826411261, 10.00000000000000000 ) ) ;
#57837=VECTOR ( 'NONE', #6935, 1000.000000000000227 ) ;
#57842=EDGE_CURVE ( 'NONE', #511, #34323, #14105, .T. ) ;
#57873=EDGE_CURVE ( 'NONE', #99391, #21781, #37331, .T. ) ;
#57875=ORIENTED_EDGE ( 'NONE', *, *, #4979, .T. ) ;
#57881=ORIENTED_EDGE ( 'NONE', *, *, #45583, .T. ) ;
#57887=VECTOR ( 'NONE', #49884, 1000.000000000000000 ) ;
#57892=DIRECTION ( 'NONE',  ( -0.7300871660154473197, -0.6833540297821713017, 0.000000000000000000 ) ) ;
#57894=AXIS2_PLACEMENT_3D ( 'NONE', #63666, #94605, #73776 ) ;
#57896=ORIENTED_EDGE ( 'NONE', *, *, #33447, .T. ) ;
#57900=CARTESIAN_POINT ( 'NONE',  ( -76.49344163160110099, 52.20945622995200353, 10.00000000000000000 ) ) ;
#57906=ORIENTED_EDGE ( 'NONE', *, *, #77673, .T. ) ;
#57908=ORIENTED_EDGE ( 'NONE', *, *, #87119, .F. ) ;
#57909=CIRCLE ( 'NONE', #78988, 70.00000000000001421 ) ;
#57912=CARTESIAN_POINT ( 'NONE',  ( -19.77743847219115736, 93.13331211188449288, 59.99999999999999289 ) ) ;
#57914=CARTESIAN_POINT ( 'NONE',  ( -73.81593683174928344, 48.72104262922893270, 177.5919119679930134 ) ) ;
#57917=VECTOR ( 'NONE', #29473, 1000.000000000000114 ) ;
#57923=ORIENTED_EDGE ( 'NONE', *, *, #40794, .T. ) ;
#57928=LINE ( 'NONE', #4225, #81368 ) ;
#57934=CIRCLE ( 'NONE', #90385, 0.1418229129681557177 ) ;
#57947=ORIENTED_EDGE ( 'NONE', *, *, #75812, .T. ) ;
#57949=EDGE_CURVE ( 'NONE', #84697, #71153, #6453, .T. ) ;
#57961=AXIS2_PLACEMENT_3D ( 'NONE', #52958, #52456, #28662 ) ;
#57963=VECTOR ( 'NONE', #14297, 1000.000000000000000 ) ;
#57965=VECTOR ( 'NONE', #41339, 1000.000000000000000 ) ;
#57984=VECTOR ( 'NONE', #62495, 1000.000000000000000 ) ;
#57987=EDGE_CURVE ( 'NONE', #20542, #57548, #9441, .T. ) ;
#58000=CARTESIAN_POINT ( 'NONE',  ( -71.61465314115659453, 63.06504152958490295, 20.00000000000001776 ) ) ;
#58004=CIRCLE ( 'NONE', #1398, 70.00000000000001421 ) ;
#58008=DIRECTION ( 'NONE',  ( -0.000000000000000000, -0.000000000000000000, -1.000000000000000000 ) ) ;
#58014=PLANE ( 'NONE',  #50633 ) ;
#58025=ORIENTED_EDGE ( 'NONE', *, *, #98597, .T. ) ;
#58030=VERTEX_POINT ( 'NONE', #54508 ) ;
#58033=ORIENTED_EDGE ( 'NONE', *, *, #55089, .T. ) ;
#58040=DIRECTION ( 'NONE',  ( 0.000000000000000000, 0.000000000000000000, 1.000000000000000000 ) ) ;
#58041=AXIS2_PLACEMENT_3D ( 'NONE', #91174, #21250, #69334 ) ;
#58048=VECTOR ( 'NONE', #46399, 1000.000000000000114 ) ;
#58051=CARTESIAN_POINT ( 'NONE',  ( -7.194219815981691468, 36.47589951538922293, 59.99999999999999289 ) ) ;
#58053=DIRECTION ( 'NONE',  ( 0.000000000000000000, -0.000000000000000000, -1.000000000000000000 ) ) ;
#58059=VECTOR ( 'NONE', #37562, 1000.000000000000114 ) ;
#58060=VERTEX_POINT ( 'NONE', #65136 ) ;
#58061=DIRECTION ( 'NONE',  ( 0.000000000000000000, 0.000000000000000000, 1.000000000000000000 ) ) ;
#58063=ORIENTED_EDGE ( 'NONE', *, *, #82041, .T. ) ;
#58071=AXIS2_PLACEMENT_3D ( 'NONE', #83168, #7622, #15712 ) ;
#58094=CARTESIAN_POINT ( 'NONE',  ( -76.23101443460923576, 54.01191295053621388, 10.00000000000000000 ) ) ;
#58100=AXIS2_PLACEMENT_3D ( 'NONE', #3457, #41931, #11555 ) ;
#58103=CARTESIAN_POINT ( 'NONE',  ( -19.58619053749203331, 92.94000956414772929, 59.99999999999999289 ) ) ;
#58109=EDGE_LOOP ( 'NONE', ( #70582, #54619, #56269, #56507 ) ) ;
#58111=VECTOR ( 'NONE', #251, 1000.000000000000000 ) ;
#58129=ORIENTED_EDGE ( 'NONE', *, *, #48708, .T. ) ;
#58132=DIRECTION ( 'NONE',  ( -1.000000000000000000, 0.000000000000000000, 0.000000000000000000 ) ) ;
#58136=VECTOR ( 'NONE', #59453, 1000.000000000000000 ) ;
#58141=VERTEX_POINT ( 'NONE', #36718 ) ;
#58149=DIRECTION ( 'NONE',  ( -0.8450603975019854719, 0.5346708562973919721, 0.000000000000000000 ) ) ;
#58152=DIRECTION ( 'NONE',  ( -0.3696446237802450407, -0.9291732088853839056, 0.000000000000000000 ) ) ;
#58168=FACE_OUTER_BOUND ( 'NONE', #33331, .T. ) ;
#58169=DIRECTION ( 'NONE',  ( -0.9874311856918890351, 0.1580495287025880657, 0.000000000000000000 ) ) ;
#58171=VECTOR ( 'NONE', #7383, 1000.000000000000227 ) ;
#58191=VECTOR ( 'NONE', #21107, 1000.000000000000000 ) ;
#58204=VECTOR ( 'NONE', #51214, 1000.000000000000000 ) ;
#58212=ORIENTED_EDGE ( 'NONE', *, *, #28118, .T. ) ;
#58220=CARTESIAN_POINT ( 'NONE',  ( 23.64814127513158226, 118.0650415295850451, -45.00000000000001421 ) ) ;
#58223=DIRECTION ( 'NONE',  ( 0.000000000000000000, 0.000000000000000000, 1.000000000000000000 ) ) ;
#58225=CARTESIAN_POINT ( 'NONE',  ( -19.65312891409030271, 93.06504152958497400, 10.00000000000000888 ) ) ;
#58227=PLANE ( 'NONE',  #26426 ) ;
#58232=LINE ( 'NONE', #34444, #52941 ) ;
#58234=VECTOR ( 'NONE', #79887, 1000.000000000000227 ) ;
#58247=PLANE ( 'NONE',  #76935 ) ;
#58258=LINE ( 'NONE', #25368, #50773 ) ;
#58260=VERTEX_POINT ( 'NONE', #86882 ) ;
#58274=ORIENTED_EDGE ( 'NONE', *, *, #8360, .F. ) ;
#58276=FACE_BOUND ( 'NONE', #75587, .T. ) ;
#58281=CARTESIAN_POINT ( 'NONE',  ( -42.72532191160158987, 28.29708160126036987, -10.00000000000000000 ) ) ;
#58283=VERTEX_POINT ( 'NONE', #16413 ) ;
#58287=ORIENTED_EDGE ( 'NONE', *, *, #75084, .F. ) ;
#58291=LINE ( 'NONE', #43072, #43216 ) ;
#58309=FACE_OUTER_BOUND ( 'NONE', #93042, .T. ) ;
#58312=CARTESIAN_POINT ( 'NONE',  ( -21.31413092498266693, 24.33771760303832465, 10.00000000000000000 ) ) ;
#58315=DIRECTION ( 'NONE',  ( 1.000000000000000000, 0.000000000000000000, 0.000000000000000000 ) ) ;
#58320=CARTESIAN_POINT ( 'NONE',  ( 38.52196584993465223, 56.41980893122115504, -10.00000000000000000 ) ) ;
#58323=AXIS2_PLACEMENT_3D ( 'NONE', #17448, #66049, #34159 ) ;
#58337=DIRECTION ( 'NONE',  ( 1.000000000000000000, 0.000000000000000000, -0.000000000000000000 ) ) ;
#58342=FACE_OUTER_BOUND ( 'NONE', #97442, .T. ) ;
#58355=DIRECTION ( 'NONE',  ( 0.000000000000000000, 0.000000000000000000, 1.000000000000000000 ) ) ;
#58360=CARTESIAN_POINT ( 'NONE',  ( -19.65312891409030271, 93.06504152958497400, -10.00000000000000888 ) ) ;
#58363=EDGE_LOOP ( 'NONE', ( #90690, #82280, #92200, #53060 ) ) ;
#58366=DIRECTION ( 'NONE',  ( 0.6602847420308605164, 0.7510153523339188064, 0.000000000000000000 ) ) ;
#58375=CARTESIAN_POINT ( 'NONE',  ( -19.65312891409030271, 93.06504152958497400, 177.5919119679930134 ) ) ;
#58378=ORIENTED_EDGE ( 'NONE', *, *, #73954, .T. ) ;
#58383=FACE_OUTER_BOUND ( 'NONE', #7226, .T. ) ;
#58394=ADVANCED_FACE ( 'NONE', ( #69486 ), #23375, .F. ) ;
#58397=CARTESIAN_POINT ( 'NONE',  ( 24.46206622376873696, 38.38158625946101665, -10.00000000000000000 ) ) ;
#58405=CARTESIAN_POINT ( 'NONE',  ( 4.268087542569434234, 45.74354613382861601, 59.99999999999999289 ) ) ;
#58410=DIRECTION ( 'NONE',  ( 0.2165469281463284490, -0.9762722099447412871, 0.000000000000000000 ) ) ;
#58411=DIRECTION ( 'NONE',  ( 0.1266907948509091442, -0.9919422576440851680, 0.000000000000000000 ) ) ;
#58414=ORIENTED_EDGE ( 'NONE', *, *, #65985, .F. ) ;
#58416=EDGE_CURVE ( 'NONE', #73348, #91080, #83736, .T. ) ;
#58425=CARTESIAN_POINT ( 'NONE',  ( -19.78671505388745899, 93.01741294681296779, 59.99999999999999289 ) ) ;
#58430=EDGE_CURVE ( 'NONE', #91738, #25484, #7733, .T. ) ;
#58436=ORIENTED_EDGE ( 'NONE', *, *, #86739, .T. ) ;
#58439=EDGE_CURVE ( 'NONE', #53634, #3488, #12472, .T. ) ;
#58442=LINE ( 'NONE', #82798, #56223 ) ;
#58443=CARTESIAN_POINT ( 'NONE',  ( -61.39381520214497101, 38.43978098112751951, 10.00000000000000000 ) ) ;
#58446=CYLINDRICAL_SURFACE ( 'NONE', #31955, 49.99999999999999289 ) ;
#58463=AXIS2_PLACEMENT_3D ( 'NONE', #98169, #37329, #22142 ) ;
#58478=LINE ( 'NONE', #12411, #10303 ) ;
#58479=ORIENTED_EDGE ( 'NONE', *, *, #20877, .F. ) ;
#58489=ORIENTED_EDGE ( 'NONE', *, *, #31168, .F. ) ;
#58502=DIRECTION ( 'NONE',  ( -0.001635407438361268905, -0.9999986627203610867, 0.000000000000000000 ) ) ;
#58503=VERTEX_POINT ( 'NONE', #88752 ) ;
#58508=ORIENTED_EDGE ( 'NONE', *, *, #62275, .T. ) ;
#58515=ORIENTED_EDGE ( 'NONE', *, *, #43248, .F. ) ;
#58524=DIRECTION ( 'NONE',  ( -0.1239754375649670948, -0.9922852870422774751, 0.000000000000000000 ) ) ;
#58533=VERTEX_POINT ( 'NONE', #43578 ) ;
#58543=DIRECTION ( 'NONE',  ( 0.4999999999999999445, -0.8660254037844385966, 0.000000000000000000 ) ) ;
#58544=ADVANCED_FACE ( 'NONE', ( #26898 ), #90232, .F. ) ;
#58548=EDGE_CURVE ( 'NONE', #45907, #57548, #57776, .T. ) ;
#58550=CARTESIAN_POINT ( 'NONE',  ( -19.65312891409030271, 93.06504152958497400, -10.00000000000000888 ) ) ;
#58551=LINE ( 'NONE', #65164, #85498 ) ;
#58553=CARTESIAN_POINT ( 'NONE',  ( -19.65312891409030271, 93.06504152958497400, -10.00000000000000888 ) ) ;
#58554=LINE ( 'NONE', #89526, #8020 ) ;
#58558=ADVANCED_FACE ( 'NONE', ( #21294 ), #80639, .F. ) ;
#58574=CARTESIAN_POINT ( 'NONE',  ( -19.65312891409030271, 93.06504152958497400, -45.00000000000001421 ) ) ;
#58577=CARTESIAN_POINT ( 'NONE',  ( -19.65312891409030271, 93.06504152958497400, -10.00000000000000888 ) ) ;
#58606=VERTEX_POINT ( 'NONE', #61762 ) ;
#58611=ORIENTED_EDGE ( 'NONE', *, *, #71694, .F. ) ;
#58618=DIRECTION ( 'NONE',  ( -0.000000000000000000, 0.000000000000000000, -1.000000000000000000 ) ) ;
#58636=PLANE ( 'NONE',  #54980 ) ;
#58639=CARTESIAN_POINT ( 'NONE',  ( -19.65312891409030271, 93.06504152958497400, 177.5919119679930134 ) ) ;
#58644=ORIENTED_EDGE ( 'NONE', *, *, #67817, .T. ) ;
#58647=CIRCLE ( 'NONE', #451, 70.00000000000001421 ) ;
#58648=DIRECTION ( 'NONE',  ( -1.000000000000000000, -9.785293164110126558E-14, 0.000000000000000000 ) ) ;
#58655=ADVANCED_FACE ( 'NONE', ( #95227 ), #49082, .F. ) ;
#58657=ORIENTED_EDGE ( 'NONE', *, *, #86847, .F. ) ;
#58664=DIRECTION ( 'NONE',  ( 0.9985601716053736920, -0.05364311403569550080, 0.000000000000000000 ) ) ;
#58669=EDGE_CURVE ( 'NONE', #45905, #99910, #80015, .T. ) ;
#58670=DIRECTION ( 'NONE',  ( -0.5372068985985075651, -0.8434505012732950169, 0.000000000000000000 ) ) ;
#58680=CARTESIAN_POINT ( 'NONE',  ( 48.48788556946983874, 102.1758113618167982, 10.00000000000000000 ) ) ;
#58684=CARTESIAN_POINT ( 'NONE',  ( -2.330697855141256269, 26.52822386297705393, -10.00000000000000000 ) ) ;
#58687=DIRECTION ( 'NONE',  ( -0.1344185706417126702, 0.9909246428798905715, 0.000000000000000000 ) ) ;
#58693=ORIENTED_EDGE ( 'NONE', *, *, #100054, .T. ) ;
#58696=LINE ( 'NONE', #20231, #3063 ) ;
#58717=VERTEX_POINT ( 'NONE', #55154 ) ;
#58718=DIRECTION ( 'NONE',  ( -0.9839629614562445115, 0.1783728972749415165, 0.000000000000000000 ) ) ;
#58719=PLANE ( 'NONE',  #74041 ) ;
#58721=ORIENTED_EDGE ( 'NONE', *, *, #13604, .T. ) ;
#58722=VECTOR ( 'NONE', #13890, 1000.000000000000000 ) ;
#58723=DIRECTION ( 'NONE',  ( -0.7694697644498993405, 0.6386832404231509441, 0.000000000000000000 ) ) ;
#58725=CARTESIAN_POINT ( 'NONE',  ( -19.65312891409030271, 93.06504152958497400, 177.5919119679930134 ) ) ;
#58727=DIRECTION ( 'NONE',  ( -0.8035972437015875824, -0.5951734788405910193, 0.000000000000000000 ) ) ;
#58728=FACE_OUTER_BOUND ( 'NONE', #85528, .T. ) ;
#58732=DIRECTION ( 'NONE',  ( 0.000000000000000000, 0.000000000000000000, 1.000000000000000000 ) ) ;
#58734=ORIENTED_EDGE ( 'NONE', *, *, #70890, .T. ) ;
#58736=ADVANCED_FACE ( 'NONE', ( #86140 ), #40947, .F. ) ;
#58744=DIRECTION ( 'NONE',  ( 0.000000000000000000, 0.000000000000000000, 1.000000000000000000 ) ) ;
#58754=CARTESIAN_POINT ( 'NONE',  ( -76.86719868626529717, 52.73452925779879763, 10.00000000000000000 ) ) ;
#58759=ORIENTED_EDGE ( 'NONE', *, *, #72142, .T. ) ;
#58761=FACE_BOUND ( 'NONE', #40565, .T. ) ;
#58772=ORIENTED_EDGE ( 'NONE', *, *, #59510, .T. ) ;
#58791=CARTESIAN_POINT ( 'NONE',  ( 34.97213163436671124, 51.32435524152969464, 10.00000000000000000 ) ) ;
#58794=PLANE ( 'NONE',  #98567 ) ;
#58798=CIRCLE ( 'NONE', #75110, 0.1418229129684644985 ) ;
#58800=DIRECTION ( 'NONE',  ( 0.000000000000000000, 0.000000000000000000, 1.000000000000000000 ) ) ;
#58813=EDGE_CURVE ( 'NONE', #8200, #5590, #26775, .T. ) ;
#58850=LINE ( 'NONE', #67469, #67604 ) ;
#58854=ORIENTED_EDGE ( 'NONE', *, *, #8879, .T. ) ;
#58859=ORIENTED_EDGE ( 'NONE', *, *, #19232, .F. ) ;
#58863=VERTEX_POINT ( 'NONE', #57156 ) ;
#58867=AXIS2_PLACEMENT_3D ( 'NONE', #13653, #91180, #75976 ) ;
#58869=ORIENTED_EDGE ( 'NONE', *, *, #89149, .T. ) ;
#58874=EDGE_LOOP ( 'NONE', ( #92420, #36559, #21572, #70587 ) ) ;
#58877=VERTEX_POINT ( 'NONE', #13087 ) ;
#58883=CARTESIAN_POINT ( 'NONE',  ( -1.087500518889665591, 25.57194971796826621, 177.5919119679930134 ) ) ;
#58892=DIRECTION ( 'NONE',  ( 0.000000000000000000, 0.000000000000000000, 1.000000000000000000 ) ) ;
#58893=VERTEX_POINT ( 'NONE', #97208 ) ;
#58903=ORIENTED_EDGE ( 'NONE', *, *, #3427, .T. ) ;
#58913=CARTESIAN_POINT ( 'NONE',  ( -4.731736819106164837, 24.67387208536690224, -10.00000000000000000 ) ) ;
#58915=EDGE_CURVE ( 'NONE', #21781, #79669, #17181, .T. ) ;
#58923=AXIS2_PLACEMENT_3D ( 'NONE', #38249, #270, #84907 ) ;
#58924=DIRECTION ( 'NONE',  ( 0.000000000000000000, 0.000000000000000000, 1.000000000000000000 ) ) ;
#58934=DIRECTION ( 'NONE',  ( -0.7080737730998298840, 0.7061384650677022812, 0.000000000000000000 ) ) ;
#58960=EDGE_LOOP ( 'NONE', ( #45568, #58274, #42186, #95067 ) ) ;
#58971=ADVANCED_FACE ( 'NONE', ( #38341 ), #61643, .F. ) ;
#58976=LINE ( 'NONE', #21511, #30345 ) ;
#58981=EDGE_CURVE ( 'NONE', #53400, #81007, #38207, .T. ) ;
#58991=EDGE_CURVE ( 'NONE', #84837, #39540, #37841, .T. ) ;
#58995=ORIENTED_EDGE ( 'NONE', *, *, #41945, .T. ) ;
#58997=AXIS2_PLACEMENT_3D ( 'NONE', #6716, #91852, #68506 ) ;
#59006=AXIS2_PLACEMENT_3D ( 'NONE', #93900, #25452, #80200 ) ;
#59009=VERTEX_POINT ( 'NONE', #23138 ) ;
#59010=LINE ( 'NONE', #89502, #57681 ) ;
#59030=DIRECTION ( 'NONE',  ( 0.9755587037855241173, -0.2197389712097240766, 0.000000000000000000 ) ) ;
#59031=DIRECTION ( 'NONE',  ( 0.03004293549036790231, 0.9995486091367050685, 0.000000000000000000 ) ) ;
#59039=ORIENTED_EDGE ( 'NONE', *, *, #80791, .F. ) ;
#59041=LINE ( 'NONE', #45351, #14512 ) ;
#59046=CARTESIAN_POINT ( 'NONE',  ( -19.65312891409030271, 93.06504152958497400, -25.00000000000000000 ) ) ;
#59047=CARTESIAN_POINT ( 'NONE',  ( -19.65312891409030271, 93.06504152958497400, 177.5919119679930134 ) ) ;
#59052=EDGE_CURVE ( 'NONE', #13323, #98647, #80370, .T. ) ;
#59061=DIRECTION ( 'NONE',  ( -0.000000000000000000, -0.000000000000000000, -1.000000000000000000 ) ) ;
#59073=DIRECTION ( 'NONE',  ( -0.000000000000000000, -0.000000000000000000, -1.000000000000000000 ) ) ;
#59079=ORIENTED_EDGE ( 'NONE', *, *, #37699, .F. ) ;
#59085=ORIENTED_EDGE ( 'NONE', *, *, #54298, .F. ) ;
#59089=CARTESIAN_POINT ( 'NONE',  ( 44.44844410339183582, 68.22168590943847732, -10.00000000000000000 ) ) ;
#59096=CARTESIAN_POINT ( 'NONE',  ( -21.58168810074490551, 24.33735145887882112, -10.00000000000000000 ) ) ;
#59098=CARTESIAN_POINT ( 'NONE',  ( -50.14960082266475894, 51.27834073637188084, 59.99999999999999289 ) ) ;
#59100=VERTEX_POINT ( 'NONE', #55040 ) ;
#59102=EDGE_CURVE ( 'NONE', #72875, #91554, #95104, .T. ) ;
#59107=VECTOR ( 'NONE', #59268, 1000.000000000000000 ) ;
#59108=ADVANCED_FACE ( 'NONE', ( #24646 ), #62632, .F. ) ;
#59115=DIRECTION ( 'NONE',  ( 0.4525327339300069251, -0.8917477921037054722, 0.000000000000000000 ) ) ;
#59120=PLANE ( 'NONE',  #46378 ) ;
#59137=CARTESIAN_POINT ( 'NONE',  ( -39.52511050156713424, 25.94496742513404541, 10.00000000000000000 ) ) ;
#59138=ORIENTED_EDGE ( 'NONE', *, *, #27206, .T. ) ;
#59161=DIRECTION ( 'NONE',  ( 0.2398044646550112069, 0.9708212084269294273, 0.000000000000000000 ) ) ;
#59164=CARTESIAN_POINT ( 'NONE',  ( 0.4893710859096792598, 78.77562236714182120, 59.99999999999999289 ) ) ;
#59166=EDGE_CURVE ( 'NONE', #45437, #78482, #63149, .T. ) ;
#59167=VECTOR ( 'NONE', #84996, 1000.000000000000000 ) ;
#59168=LINE ( 'NONE', #68786, #6056 ) ;
#59176=CIRCLE ( 'NONE', #15510, 70.00000000000001421 ) ;
#59178=ADVANCED_FACE ( 'NONE', ( #35248 ), #49449, .T. ) ;
#59186=DIRECTION ( 'NONE',  ( 1.000000000000000000, -1.784287003861858500E-15, 0.000000000000000000 ) ) ;
#59194=VECTOR ( 'NONE', #67798, 1000.000000000000000 ) ;
#59195=ORIENTED_EDGE ( 'NONE', *, *, #30736, .T. ) ;
#59199=CARTESIAN_POINT ( 'NONE',  ( -74.22192597045216189, 49.22161114575668250, 177.5919119679930134 ) ) ;
#59201=PLANE ( 'NONE',  #68480 ) ;
#59202=EDGE_CURVE ( 'NONE', #1860, #71477, #43337, .T. ) ;
#59211=LINE ( 'NONE', #90186, #44102 ) ;
#59213=EDGE_CURVE ( 'NONE', #58260, #10169, #80403, .T. ) ;
#59219=ORIENTED_EDGE ( 'NONE', *, *, #56574, .F. ) ;
#59221=DIRECTION ( 'NONE',  ( -0.000000000000000000, -0.000000000000000000, -1.000000000000000000 ) ) ;
#59223=CARTESIAN_POINT ( 'NONE',  ( -63.34358462235559273, 38.37368864812747660, 10.00000000000000000 ) ) ;
#59229=ORIENTED_EDGE ( 'NONE', *, *, #58981, .T. ) ;
#59230=ORIENTED_EDGE ( 'NONE', *, *, #91802, .T. ) ;
#59235=CYLINDRICAL_SURFACE ( 'NONE', #35293, 70.00000000000002842 ) ;
#59236=FACE_OUTER_BOUND ( 'NONE', #8674, .T. ) ;
#59248=ORIENTED_EDGE ( 'NONE', *, *, #16462, .T. ) ;
#59251=DIRECTION ( 'NONE',  ( 0.000000000000000000, 0.000000000000000000, 1.000000000000000000 ) ) ;
#59256=AXIS2_PLACEMENT_3D ( 'NONE', #67759, #37836, #37341 ) ;
#59268=DIRECTION ( 'NONE',  ( 0.000000000000000000, -0.000000000000000000, 1.000000000000000000 ) ) ;
#59270=DIRECTION ( 'NONE',  ( -1.000000000000000000, 0.000000000000000000, 0.000000000000000000 ) ) ;
#59275=VECTOR ( 'NONE', #13498, 1000.000000000000227 ) ;
#59281=CARTESIAN_POINT ( 'NONE',  ( -19.65312891409030271, 93.06504152958497400, 10.00000000000000888 ) ) ;
#59282=DIRECTION ( 'NONE',  ( -1.000000000000000000, 0.000000000000000000, 0.000000000000000000 ) ) ;
#59297=PLANE ( 'NONE',  #59583 ) ;
#59299=ADVANCED_FACE ( 'NONE', ( #75761 ), #43837, .F. ) ;
#59307=CARTESIAN_POINT ( 'NONE',  ( 39.00599428327696216, 91.66936899913777381, 59.99999999999999289 ) ) ;
#59310=CIRCLE ( 'NONE', #15652, 0.1418229129681591871 ) ;
#59322=CARTESIAN_POINT ( 'NONE',  ( -19.65312891409030271, 93.06504152958497400, 177.5919119679930134 ) ) ;
#59324=CARTESIAN_POINT ( 'NONE',  ( -63.39619785071779035, 38.08345695496143435, 10.00000000000000000 ) ) ;
#59347=VERTEX_POINT ( 'NONE', #3263 ) ;
#59350=VECTOR ( 'NONE', #13913, 1000.000000000000000 ) ;
#59362=VERTEX_POINT ( 'NONE', #64541 ) ;
#59369=VERTEX_POINT ( 'NONE', #41216 ) ;
#59373=DIRECTION ( 'NONE',  ( 0.000000000000000000, -0.000000000000000000, -1.000000000000000000 ) ) ;
#59375=ORIENTED_EDGE ( 'NONE', *, *, #65804, .F. ) ;
#59382=LINE ( 'NONE', #90358, #9100 ) ;
#59388=VECTOR ( 'NONE', #90547, 1000.000000000000114 ) ;
#59396=VECTOR ( 'NONE', #41636, 1000.000000000000000 ) ;
#59397=VERTEX_POINT ( 'NONE', #49342 ) ;
#59404=ORIENTED_EDGE ( 'NONE', *, *, #5913, .T. ) ;
#59412=CARTESIAN_POINT ( 'NONE',  ( 47.96820964746023463, 80.67316705762479501, -10.00000000000000000 ) ) ;
#59416=DIRECTION ( 'NONE',  ( 0.000000000000000000, 0.000000000000000000, 1.000000000000000000 ) ) ;
#59417=VECTOR ( 'NONE', #64256, 1000.000000000000227 ) ;
#59425=EDGE_CURVE ( 'NONE', #38681, #53400, #27046, .T. ) ;
#59428=AXIS2_PLACEMENT_3D ( 'NONE', #56199, #48630, #42012 ) ;
#59430=VERTEX_POINT ( 'NONE', #73158 ) ;
#59434=DIRECTION ( 'NONE',  ( 1.000000000000000000, 0.000000000000000000, 0.000000000000000000 ) ) ;
#59439=CARTESIAN_POINT ( 'NONE',  ( -48.71813016832984289, 30.75580926756358480, -10.00000000000000000 ) ) ;
#59443=PLANE ( 'NONE',  #11689 ) ;
#59445=EDGE_LOOP ( 'NONE', ( #47079, #22516, #44055, #40181 ) ) ;
#59449=AXIS2_PLACEMENT_3D ( 'NONE', #34882, #65296, #64807 ) ;
#59453=DIRECTION ( 'NONE',  ( 0.4458072818673325943, 0.8951289669282637140, 0.000000000000000000 ) ) ;
#59464=VERTEX_POINT ( 'NONE', #3751 ) ;
#59466=CIRCLE ( 'NONE', #54620, 70.00000000000001421 ) ;
#59470=CARTESIAN_POINT ( 'NONE',  ( -62.55022349715819274, 61.89794670847138747, 59.99999999999999289 ) ) ;
#59478=DIRECTION ( 'NONE',  ( 0.8868092729070038427, 0.4621356007560455392, 0.000000000000000000 ) ) ;
#59479=VERTEX_POINT ( 'NONE', #89394 ) ;
#59491=ORIENTED_EDGE ( 'NONE', *, *, #86667, .F. ) ;
#59498=ORIENTED_EDGE ( 'NONE', *, *, #95301, .T. ) ;
#59499=ORIENTED_EDGE ( 'NONE', *, *, #98104, .T. ) ;
#59503=ORIENTED_EDGE ( 'NONE', *, *, #6276, .T. ) ;
#59505=DIRECTION ( 'NONE',  ( 0.9919084036772433111, -0.1269555777209603886, 0.000000000000000000 ) ) ;
#59508=VECTOR ( 'NONE', #90553, 1000.000000000000227 ) ;
#59509=CARTESIAN_POINT ( 'NONE',  ( 43.16562282991919375, 123.9487658730721904, -10.00000000000000000 ) ) ;
#59510=EDGE_CURVE ( 'NONE', #934, #63771, #50820, .T. ) ;
#59520=ORIENTED_EDGE ( 'NONE', *, *, #59691, .F. ) ;
#59528=ORIENTED_EDGE ( 'NONE', *, *, #93051, .T. ) ;
#59531=ORIENTED_EDGE ( 'NONE', *, *, #65564, .F. ) ;
#59532=VECTOR ( 'NONE', #20873, 1000.000000000000000 ) ;
#59536=CARTESIAN_POINT ( 'NONE',  ( -54.21831688459418785, 33.63902229265146104, -10.00000000000000000 ) ) ;
#59537=AXIS2_PLACEMENT_3D ( 'NONE', #76593, #37572, #16283 ) ;
#59546=DIRECTION ( 'NONE',  ( -0.3402761906661169178, -0.9403255362191098587, 0.000000000000000000 ) ) ;
#59549=DIRECTION ( 'NONE',  ( 1.000000000000000000, -8.921435019309292501E-15, 0.000000000000000000 ) ) ;
#59577=CARTESIAN_POINT ( 'NONE',  ( 39.25774830830064843, 55.25619937740605536, -10.00000000000000000 ) ) ;
#59582=CARTESIAN_POINT ( 'NONE',  ( -43.77314298070450604, 40.37936670953467910, 59.99999999999999289 ) ) ;
#59583=AXIS2_PLACEMENT_3D ( 'NONE', #37997, #45602, #76535 ) ;
#59589=DIRECTION ( 'NONE',  ( 0.000000000000000000, 0.000000000000000000, 1.000000000000000000 ) ) ;
#59591=CARTESIAN_POINT ( 'NONE',  ( 47.78135487164287554, 106.4364430393875267, 10.00000000000000000 ) ) ;
#59592=ORIENTED_EDGE ( 'NONE', *, *, #13491, .T. ) ;
#59596=DIRECTION ( 'NONE',  ( 0.3301025504114333264, 0.9439450758449176027, 0.000000000000000000 ) ) ;
#59599=DIRECTION ( 'NONE',  ( 0.9795703749556662343, -0.2011016670970565412, 0.000000000000000000 ) ) ;
#59600=VECTOR ( 'NONE', #67509, 1000.000000000000000 ) ;
#59601=ORIENTED_EDGE ( 'NONE', *, *, #72458, .T. ) ;
#59602=DIRECTION ( 'NONE',  ( 1.000000000000000000, 1.038851544470682011E-13, 0.000000000000000000 ) ) ;
#59613=VECTOR ( 'NONE', #10228, 1000.000000000000227 ) ;
#59619=CARTESIAN_POINT ( 'NONE',  ( 40.34888600819125060, 126.6204015641749834, -10.00000000000000000 ) ) ;
#59622=ORIENTED_EDGE ( 'NONE', *, *, #99403, .T. ) ;
#59623=EDGE_LOOP ( 'NONE', ( #1484, #93607, #84572, #89579 ) ) ;
#59625=AXIS2_PLACEMENT_3D ( 'NONE', #88579, #19141, #50015 ) ;
#59630=PLANE ( 'NONE',  #79680 ) ;
#59634=EDGE_CURVE ( 'NONE', #45676, #62226, #14323, .T. ) ;
#59639=ORIENTED_EDGE ( 'NONE', *, *, #23766, .F. ) ;
#59641=CARTESIAN_POINT ( 'NONE',  ( -19.65312891409030271, 93.06504152958497400, 177.5919119679930134 ) ) ;
#59644=VECTOR ( 'NONE', #82681, 1000.000000000000000 ) ;
#59653=ORIENTED_EDGE ( 'NONE', *, *, #75974, .T. ) ;
#59655=CARTESIAN_POINT ( 'NONE',  ( 12.00096474099108690, 32.03863464977599307, -10.00000000000000000 ) ) ;
#59663=ORIENTED_EDGE ( 'NONE', *, *, #31411, .T. ) ;
#59665=DIRECTION ( 'NONE',  ( -0.1344185706417126702, 0.9909246428798905715, 0.000000000000000000 ) ) ;
#59666=EDGE_CURVE ( 'NONE', #74753, #5335, #93349, .T. ) ;
#59669=CARTESIAN_POINT ( 'NONE',  ( 42.45923888023187232, 122.5484010731363043, -10.00000000000000000 ) ) ;
#59676=CIRCLE ( 'NONE', #98554, 0.1418229129681557177 ) ;
#59683=EDGE_CURVE ( 'NONE', #5590, #49899, #18199, .T. ) ;
#59684=VECTOR ( 'NONE', #39106, 1000.000000000000000 ) ;
#59685=EDGE_CURVE ( 'NONE', #34673, #91537, #33909, .T. ) ;
#59691=EDGE_CURVE ( 'NONE', #66505, #28484, #88151, .T. ) ;
#59692=DIRECTION ( 'NONE',  ( 0.4803199113995043623, -0.8770933717188679202, 0.000000000000000000 ) ) ;
#59693=EDGE_CURVE ( 'NONE', #20300, #77610, #8718, .T. ) ;
#59694=DIRECTION ( 'NONE',  ( 0.000000000000000000, -0.000000000000000000, -1.000000000000000000 ) ) ;
#59695=DIRECTION ( 'NONE',  ( -0.9186857246103535823, 0.3949892902309500298, 0.000000000000000000 ) ) ;
#59698=CIRCLE ( 'NONE', #38657, 0.1418229129681539691 ) ;
#59706=VECTOR ( 'NONE', #65582, 1000.000000000000000 ) ;
#59709=CARTESIAN_POINT ( 'NONE',  ( -20.01016364259690050, 23.06595206263088116, 177.5919119679930134 ) ) ;
#59728=ORIENTED_EDGE ( 'NONE', *, *, #45697, .F. ) ;
#59729=DIRECTION ( 'NONE',  ( -0.8660254037844379305, -0.5000000000000011102, 0.000000000000000000 ) ) ;
#59731=DIRECTION ( 'NONE',  ( 0.8080546441192343332, -0.5891075386695858729, 0.000000000000000000 ) ) ;
#59741=LINE ( 'NONE', #73475, #95139 ) ;
#59754=VECTOR ( 'NONE', #32035, 1000.000000000000000 ) ;
#59758=FACE_OUTER_BOUND ( 'NONE', #38985, .T. ) ;
#59760=VECTOR ( 'NONE', #24547, 1000.000000000000000 ) ;
#59761=DIRECTION ( 'NONE',  ( 0.9954067278227227700, -0.09573633691164462611, 0.000000000000000000 ) ) ;
#59773=ORIENTED_EDGE ( 'NONE', *, *, #46049, .F. ) ;
#59776=DIRECTION ( 'NONE',  ( -0.6118251767726359258, -0.7909930170786165782, 0.000000000000000000 ) ) ;
#59777=DIRECTION ( 'NONE',  ( 0.3595896960900372696, 0.9331105242498740626, 0.000000000000000000 ) ) ;
#59807=ADVANCED_FACE ( 'NONE', ( #21683 ), #46451, .F. ) ;
#59808=EDGE_CURVE ( 'NONE', #93198, #68897, #39862, .T. ) ;
#59829=DIRECTION ( 'NONE',  ( -0.6778389383370750920, -0.7352104281592222179, 0.000000000000000000 ) ) ;
#59851=CARTESIAN_POINT ( 'NONE',  ( -12.68721568607400485, 24.67147432707382748, 10.00000000000000000 ) ) ;
#59861=CARTESIAN_POINT ( 'NONE',  ( -23.47208873469913115, 24.42380372261332155, 10.00000000000000000 ) ) ;
#59865=EDGE_LOOP ( 'NONE', ( #67477, #93891, #76224, #84592 ) ) ;
#59868=CARTESIAN_POINT ( 'NONE',  ( -23.47208873469913470, 24.42380372261331800, -10.00000000000000000 ) ) ;
#59870=ORIENTED_EDGE ( 'NONE', *, *, #20842, .T. ) ;
#59873=PLANE ( 'NONE',  #45102 ) ;
#59878=EDGE_LOOP ( 'NONE', ( #62372, #4187, #35096, #65609 ) ) ;
#59879=CARTESIAN_POINT ( 'NONE',  ( 13.90223112049948639, 33.06302660730328569, -10.00000000000000000 ) ) ;
#59880=LINE ( 'NONE', #21400, #10590 ) ;
#59889=ORIENTED_EDGE ( 'NONE', *, *, #84509, .T. ) ;
#59905=DIRECTION ( 'NONE',  ( 0.000000000000000000, 0.000000000000000000, 1.000000000000000000 ) ) ;
#59913=VECTOR ( 'NONE', #12229, 1000.000000000000000 ) ;
#59923=CARTESIAN_POINT ( 'NONE',  ( -23.32062891409032090, 78.77562236714182120, 59.99999999999999289 ) ) ;
#59925=DIRECTION ( 'NONE',  ( 0.000000000000000000, -0.000000000000000000, -1.000000000000000000 ) ) ;
#59932=CARTESIAN_POINT ( 'NONE',  ( -19.65312891409030271, 93.06504152958497400, 59.99999999999999289 ) ) ;
#59936=ORIENTED_EDGE ( 'NONE', *, *, #27387, .F. ) ;
#59945=CARTESIAN_POINT ( 'NONE',  ( 50.20806676147353187, 85.59215312471712878, -10.00000000000000000 ) ) ;
#59964=VERTEX_POINT ( 'NONE', #71173 ) ;
#59965=DIRECTION ( 'NONE',  ( 0.9994538543569184696, -0.03304531753667278027, 0.000000000000000000 ) ) ;
#59979=CARTESIAN_POINT ( 'NONE',  ( -46.49770490450612215, 29.77544742692501600, 10.00000000000000000 ) ) ;
#60001=EDGE_CURVE ( 'NONE', #52454, #70967, #253, .T. ) ;
#60013=DIRECTION ( 'NONE',  ( -0.9514785060800223793, 0.3077152132536332130, 0.000000000000000000 ) ) ;
#60020=ORIENTED_EDGE ( 'NONE', *, *, #15064, .F. ) ;
#60027=PLANE ( 'NONE',  #74895 ) ;
#60043=VERTEX_POINT ( 'NONE', #75594 ) ;
#60045=PLANE ( 'NONE',  #57961 ) ;
#60049=AXIS2_PLACEMENT_3D ( 'NONE', #96918, #81709, #5170 ) ;
#60059=CARTESIAN_POINT ( 'NONE',  ( 48.87252615048947746, 107.3561085985702874, 177.5919119679930134 ) ) ;
#60060=EDGE_CURVE ( 'NONE', #13198, #49332, #60356, .T. ) ;
#60064=DIRECTION ( 'NONE',  ( 0.6313854049612632746, 0.7754691937155863135, 0.000000000000000000 ) ) ;
#60065=LINE ( 'NONE', #21592, #70812 ) ;
#60066=DIRECTION ( 'NONE',  ( -0.7080737730998298840, 0.7061384650677022812, 0.000000000000000000 ) ) ;
#60088=DIRECTION ( 'NONE',  ( -0.7763215174174871169, 0.6303371332823493045, 0.000000000000000000 ) ) ;
#60095=DIRECTION ( 'NONE',  ( 0.8660254037844379305, 0.5000000000000011102, 0.000000000000000000 ) ) ;
#60097=VERTEX_POINT ( 'NONE', #7676 ) ;
#60102=ORIENTED_EDGE ( 'NONE', *, *, #68341, .F. ) ;
#60110=DIRECTION ( 'NONE',  ( 0.4737039832092511671, 0.8806841296921895657, 0.000000000000000000 ) ) ;
#60113=EDGE_CURVE ( 'NONE', #5348, #61424, #10844, .T. ) ;
#60114=DIRECTION ( 'NONE',  ( 0.000000000000000000, 0.000000000000000000, 1.000000000000000000 ) ) ;
#60123=DIRECTION ( 'NONE',  ( 0.000000000000000000, 0.000000000000000000, 1.000000000000000000 ) ) ;
#60125=CARTESIAN_POINT ( 'NONE',  ( 13.75631770279071020, 31.55236904046464375, -10.00000000000000000 ) ) ;
#60136=DIRECTION ( 'NONE',  ( 0.000000000000000000, 0.000000000000000000, 1.000000000000000000 ) ) ;
#60138=EDGE_LOOP ( 'NONE', ( #66904, #59138, #77867, #2471 ) ) ;
#60144=EDGE_LOOP ( 'NONE', ( #3057, #12581, #50282, #19075 ) ) ;
#60147=CARTESIAN_POINT ( 'NONE',  ( 30.34687108590969373, 93.06504152958497400, 60.00000000000000000 ) ) ;
#60149=CARTESIAN_POINT ( 'NONE',  ( 35.47817891544688251, 110.9002400656976022, 59.99999999999999289 ) ) ;
#60160=DIRECTION ( 'NONE',  ( 0.000000000000000000, 0.000000000000000000, 1.000000000000000000 ) ) ;
#60163=CARTESIAN_POINT ( 'NONE',  ( -19.52110968745198250, 93.01322780128255374, 59.99999999999999289 ) ) ;
#60164=DIRECTION ( 'NONE',  ( 0.000000000000000000, -0.000000000000000000, 1.000000000000000000 ) ) ;
#60169=DIRECTION ( 'NONE',  ( -1.000000000000000000, 0.000000000000000000, 0.000000000000000000 ) ) ;
#60171=CARTESIAN_POINT ( 'NONE',  ( 13.90223112049948639, 33.06302660730329279, -10.00000000000000000 ) ) ;
#60174=CARTESIAN_POINT ( 'NONE',  ( -58.10760318826260118, 36.06970723555270553, -10.00000000000000000 ) ) ;
#60179=CARTESIAN_POINT ( 'NONE',  ( -46.49770490450612215, 29.77544742692501600, -10.00000000000000000 ) ) ;
#60184=ADVANCED_FACE ( 'NONE', ( #44659 ), #92806, .F. ) ;
#60192=DIRECTION ( 'NONE',  ( 0.8755176446346986108, -0.4831861483251662648, 0.000000000000000000 ) ) ;
#60194=CARTESIAN_POINT ( 'NONE',  ( 9.830230629461709668, 30.95267373526311516, -10.00000000000000000 ) ) ;
#60202=CARTESIAN_POINT ( 'NONE',  ( 35.32845566053276087, 49.32197259295687530, -10.00000000000000000 ) ) ;
#60209=ORIENTED_EDGE ( 'NONE', *, *, #25364, .F. ) ;
#60213=ORIENTED_EDGE ( 'NONE', *, *, #3885, .F. ) ;
#60221=VERTEX_POINT ( 'NONE', #69962 ) ;
#60231=ORIENTED_EDGE ( 'NONE', *, *, #28811, .T. ) ;
#60232=EDGE_CURVE ( 'NONE', #1644, #84697, #49186, .T. ) ;
#60233=DIRECTION ( 'NONE',  ( -1.000000000000000000, 0.000000000000000000, 0.000000000000000000 ) ) ;
#60242=VECTOR ( 'NONE', #97944, 1000.000000000000114 ) ;
#60246=CARTESIAN_POINT ( 'NONE',  ( 1.638219116881074022, 26.38162155862025671, 10.00000000000000000 ) ) ;
#60252=DIRECTION ( 'NONE',  ( -0.000000000000000000, 0.000000000000000000, -1.000000000000000000 ) ) ;
#60263=CARTESIAN_POINT ( 'NONE',  ( -19.65312891409030271, 93.06504152958497400, -10.00000000000000888 ) ) ;
#60264=DIRECTION ( 'NONE',  ( -0.6647600172776847449, 0.7470569720101488675, 0.000000000000000000 ) ) ;
#60265=ORIENTED_EDGE ( 'NONE', *, *, #38061, .F. ) ;
#60271=DIRECTION ( 'NONE',  ( 0.000000000000000000, 0.000000000000000000, 1.000000000000000000 ) ) ;
#60272=CYLINDRICAL_SURFACE ( 'NONE', #51259, 70.00000000000002842 ) ;
#60284=DIRECTION ( 'NONE',  ( 0.8606332181800098180, -0.5092253565614340838, 0.000000000000000000 ) ) ;
#60294=ADVANCED_FACE ( 'NONE', ( #62352 ), #93820, .T. ) ;
#60305=ADVANCED_FACE ( 'NONE', ( #87256 ), #40559, .F. ) ;
#60334=PRODUCT_CONTEXT ( 'NONE', #46600, 'mechanical' ) ;
#60349=VERTEX_POINT ( 'NONE', #94315 ) ;
#60351=ADVANCED_FACE ( 'NONE', ( #59236 ), #95831, .F. ) ;
#60356=LINE ( 'NONE', #37560, #23674 ) ;
#60358=CARTESIAN_POINT ( 'NONE',  ( -40.67952639183666008, 27.60432558407079640, -10.00000000000000000 ) ) ;
#60359=EDGE_LOOP ( 'NONE', ( #98189, #88116, #17393, #2289 ) ) ;
#60361=ADVANCED_FACE ( 'NONE', ( #81610 ), #74983, .F. ) ;
#60366=CARTESIAN_POINT ( 'NONE',  ( 4.102725850843912170, 28.55253618238880620, -10.00000000000000000 ) ) ;
#60369=FACE_OUTER_BOUND ( 'NONE', #63821, .T. ) ;
#60370=AXIS2_PLACEMENT_3D ( 'NONE', #43526, #26350, #4533 ) ;
#60372=CARTESIAN_POINT ( 'NONE',  ( -7.270353138567037021, 73.42010414804977358, 14.97951234254161257 ) ) ;
#60376=ORIENTED_EDGE ( 'NONE', *, *, #9792, .T. ) ;
#60377=ORIENTED_EDGE ( 'NONE', *, *, #74348, .T. ) ;
#60380=VECTOR ( 'NONE', #24333, 1000.000000000000000 ) ;
#60390=DIRECTION ( 'NONE',  ( 0.000000000000000000, 0.000000000000000000, 1.000000000000000000 ) ) ;
#60391=LINE ( 'NONE', #84746, #72594 ) ;
#60394=ORIENTED_EDGE ( 'NONE', *, *, #8184, .T. ) ;
#60399=CARTESIAN_POINT ( 'NONE',  ( -73.66720466879951346, 50.53642055324488780, 10.00000000000000000 ) ) ;
#60402=ORIENTED_EDGE ( 'NONE', *, *, #40056, .F. ) ;
#60417=CARTESIAN_POINT ( 'NONE',  ( 34.05451400132101014, 48.17084265633775431, 10.00000000000000000 ) ) ;
#60420=LINE ( 'NONE', #14346, #90281 ) ;
#60432=VECTOR ( 'NONE', #99863, 1000.000000000000114 ) ;
#60442=EDGE_CURVE ( 'NONE', #49563, #7148, #34472, .T. ) ;
#60447=VECTOR ( 'NONE', #98786, 1000.000000000000114 ) ;
#60450=AXIS2_PLACEMENT_3D ( 'NONE', #34781, #65683, #33295 ) ;
#60455=CARTESIAN_POINT ( 'NONE',  ( -7.338644212303985448, 23.89290704711799052, 10.00000000000000000 ) ) ;
#60464=ORIENTED_EDGE ( 'NONE', *, *, #63113, .F. ) ;
#60466=CARTESIAN_POINT ( 'NONE',  ( -41.62359735524142224, 26.60228115600144250, 177.5919119679930134 ) ) ;
#60473=ADVANCED_FACE ( 'NONE', ( #37935 ), #45053, .F. ) ;
#60481=VERTEX_POINT ( 'NONE', #76474 ) ;
#60486=VERTEX_POINT ( 'NONE', #98789 ) ;
#60495=ORIENTED_EDGE ( 'NONE', *, *, #22663, .F. ) ;
#60499=CARTESIAN_POINT ( 'NONE',  ( -11.40312891409031693, 78.77562236714182120, 52.49999999999999289 ) ) ;
#60504=DIRECTION ( 'NONE',  ( -1.000000000000000000, 0.000000000000000000, 0.000000000000000000 ) ) ;
#60511=DIRECTION ( 'NONE',  ( -0.9985601716053730259, 0.05364311403570636710, 0.000000000000000000 ) ) ;
#60521=AXIS2_PLACEMENT_3D ( 'NONE', #7496, #36904, #6010 ) ;
#60531=LINE ( 'NONE', #6361, #4128 ) ;
#60540=EDGE_LOOP ( 'NONE', ( #47049, #66489, #41556, #21626 ) ) ;
#60541=DIRECTION ( 'NONE',  ( -1.000000000000000000, 0.000000000000000000, 0.000000000000000000 ) ) ;
#60542=DIRECTION ( 'NONE',  ( 0.6056412518070691808, 0.7957378174433877849, 0.000000000000000000 ) ) ;
#60547=DIRECTION ( 'NONE',  ( -0.7511915808658203852, -0.6600842437418951159, 0.000000000000000000 ) ) ;
#60557=FACE_OUTER_BOUND ( 'NONE', #29846, .T. ) ;
#60566=ADVANCED_FACE ( 'NONE', ( #62235 ), #16158, .F. ) ;
#60567=ADVANCED_FACE ( 'NONE', ( #3957 ), #59120, .F. ) ;
#60572=DIRECTION ( 'NONE',  ( -0.9331105242498700658, 0.3595896960900473172, 0.000000000000000000 ) ) ;
#60592=PLANE ( 'NONE',  #43583 ) ;
#60598=AXIS2_PLACEMENT_3D ( 'NONE', #12327, #97436, #29504 ) ;
#60626=ORIENTED_EDGE ( 'NONE', *, *, #57718, .T. ) ;
#60630=EDGE_CURVE ( 'NONE', #22676, #76712, #34840, .T. ) ;
#60639=CARTESIAN_POINT ( 'NONE',  ( 43.53192288983094471, 62.93782412512172186, 10.00000000000000000 ) ) ;
#60642=EDGE_LOOP ( 'NONE', ( #46973, #8762, #26624, #6540 ) ) ;
#60648=CARTESIAN_POINT ( 'NONE',  ( -34.42581292930597670, 25.91608375674935871, -10.00000000000000000 ) ) ;
#60649=DIRECTION ( 'NONE',  ( 1.000000000000000000, 0.000000000000000000, 0.000000000000000000 ) ) ;
#60658=VECTOR ( 'NONE', #85648, 1000.000000000000000 ) ;
#60665=PLANE ( 'NONE',  #45064 ) ;
#60666=CARTESIAN_POINT ( 'NONE',  ( 5.404797899793122973, 27.42564005363386315, -10.00000000000000000 ) ) ;
#60667=CIRCLE ( 'NONE', #94720, 70.00000000000001421 ) ;
#60688=CIRCLE ( 'NONE', #67229, 0.1418229129681591871 ) ;
#60709=ORIENTED_EDGE ( 'NONE', *, *, #33178, .F. ) ;
#60710=CARTESIAN_POINT ( 'NONE',  ( -16.25778278694858514, 23.14743555886465032, 10.00000000000000000 ) ) ;
#60715=ORIENTED_EDGE ( 'NONE', *, *, #34281, .T. ) ;
#60720=ORIENTED_EDGE ( 'NONE', *, *, #76516, .T. ) ;
#60728=CARTESIAN_POINT ( 'NONE',  ( -69.42519150082246426, 45.64199051378594874, 10.00000000000000000 ) ) ;
#60742=ORIENTED_EDGE ( 'NONE', *, *, #82016, .T. ) ;
#60752=CARTESIAN_POINT ( 'NONE',  ( 37.48526053816526371, 54.83666944042810343, 10.00000000000000000 ) ) ;
#60755=EDGE_CURVE ( 'NONE', #85997, #95115, #89608, .T. ) ;
#60758=ORIENTED_EDGE ( 'NONE', *, *, #25612, .T. ) ;
#60759=EDGE_CURVE ( 'NONE', #10175, #46284, #73370, .T. ) ;
#60762=AXIS2_PLACEMENT_3D ( 'NONE', #40362, #33280, #56056 ) ;
#60763=CARTESIAN_POINT ( 'NONE',  ( -73.81593683174931186, 48.72104262922892559, 10.00000000000000000 ) ) ;
#60764=DIRECTION ( 'NONE',  ( -1.000000000000000000, 0.000000000000000000, 0.000000000000000000 ) ) ;
#60766=VERTEX_POINT ( 'NONE', #89128 ) ;
#60767=FACE_OUTER_BOUND ( 'NONE', #13164, .T. ) ;
#60773=CARTESIAN_POINT ( 'NONE',  ( -34.42581292930597670, 25.91608375674935161, 10.00000000000000000 ) ) ;
#60774=ORIENTED_EDGE ( 'NONE', *, *, #77078, .T. ) ;
#60783=AXIS2_PLACEMENT_3D ( 'NONE', #87683, #24796, #9630 ) ;
#60790=CARTESIAN_POINT ( 'NONE',  ( 50.26447705663006360, 96.46038765672592774, -10.00000000000000000 ) ) ;
#60791=LINE ( 'NONE', #68413, #75814 ) ;
#60798=ORIENTED_EDGE ( 'NONE', *, *, #94019, .F. ) ;
#60812=EDGE_CURVE ( 'NONE', #54901, #14998, #80000, .T. ) ;
#60825=CARTESIAN_POINT ( 'NONE',  ( -58.62427208439001447, 70.56504152958493137, 45.00000000000000711 ) ) ;
#60847=ORIENTED_EDGE ( 'NONE', *, *, #63540, .F. ) ;
#60850=ORIENTED_EDGE ( 'NONE', *, *, #40469, .F. ) ;
#60852=DIRECTION ( 'NONE',  ( -1.000000000000000000, 0.000000000000000000, 0.000000000000000000 ) ) ;
#60864=ORIENTED_EDGE ( 'NONE', *, *, #13996, .T. ) ;
#60867=ADVANCED_FACE ( 'NONE', ( #28245 ), #41444, .F. ) ;
#60869=CARTESIAN_POINT ( 'NONE',  ( 2.945768331249355665, 38.91607694435867160, 59.99999999999999289 ) ) ;
#60899=EDGE_CURVE ( 'NONE', #34934, #44815, #33884, .T. ) ;
#60903=ORIENTED_EDGE ( 'NONE', *, *, #8863, .F. ) ;
#60915=DIRECTION ( 'NONE',  ( -0.8435938723211520163, -0.5369817302126803638, 0.000000000000000000 ) ) ;
#60917=VERTEX_POINT ( 'NONE', #60125 ) ;
#60922=CARTESIAN_POINT ( 'NONE',  ( 49.66226845319755512, 83.29899382260626339, 10.00000000000000000 ) ) ;
#60924=DIRECTION ( 'NONE',  ( 0.000000000000000000, -0.000000000000000000, 1.000000000000000000 ) ) ;
#60931=ORIENTED_EDGE ( 'NONE', *, *, #10382, .T. ) ;
#60936=ADVANCED_FACE ( 'NONE', ( #85488 ), #77343, .T. ) ;
#60937=VECTOR ( 'NONE', #8483, 1000.000000000000000 ) ;
#60940=AXIS2_PLACEMENT_3D ( 'NONE', #79157, #48211, #9738 ) ;
#60942=LINE ( 'NONE', #6761, #41651 ) ;
#60944=EDGE_CURVE ( 'NONE', #81025, #14044, #40318, .T. ) ;
#60951=ORIENTED_EDGE ( 'NONE', *, *, #48102, .F. ) ;
#60962=PLANE ( 'NONE',  #78858 ) ;
#60969=ORIENTED_EDGE ( 'NONE', *, *, #72032, .T. ) ;
#60972=LINE ( 'NONE', #187, #61898 ) ;
#60976=CARTESIAN_POINT ( 'NONE',  ( -51.76626358812258388, 84.50539129967802410, -10.00000000000000000 ) ) ;
#60978=CYLINDRICAL_SURFACE ( 'NONE', #4988, 70.00000000000002842 ) ;
#60989=AXIS2_PLACEMENT_3D ( 'NONE', #14496, #45859, #68675 ) ;
#60995=ORIENTED_EDGE ( 'NONE', *, *, #75477, .T. ) ;
#60997=ORIENTED_EDGE ( 'NONE', *, *, #45322, .F. ) ;
#60999=ORIENTED_EDGE ( 'NONE', *, *, #47220, .F. ) ;
#61001=ORIENTED_EDGE ( 'NONE', *, *, #41483, .T. ) ;
#61003=CIRCLE ( 'NONE', #82114, 0.1418229129680828593 ) ;
#61011=LINE ( 'NONE', #22533, #40220 ) ;
#61017=EDGE_CURVE ( 'NONE', #97001, #29279, #16533, .T. ) ;
#61025=AXIS2_PLACEMENT_3D ( 'NONE', #85299, #62948, #157 ) ;
#61027=PLANE ( 'NONE',  #64549 ) ;
#61038=VERTEX_POINT ( 'NONE', #54016 ) ;
#61040=DIRECTION ( 'NONE',  ( 0.000000000000000000, 0.000000000000000000, 1.000000000000000000 ) ) ;
#61054=EDGE_CURVE ( 'NONE', #78693, #8334, #8443, .T. ) ;
#61055=CARTESIAN_POINT ( 'NONE',  ( -56.12829894168721978, 48.04152121768972705, 59.99999999999999289 ) ) ;
#61056=VECTOR ( 'NONE', #36507, 1000.000000000000000 ) ;
#61059=VECTOR ( 'NONE', #48275, 1000.000000000000000 ) ;
#61060=DIRECTION ( 'NONE',  ( 0.000000000000000000, 0.000000000000000000, 1.000000000000000000 ) ) ;
#61067=CARTESIAN_POINT ( 'NONE',  ( -19.51556777096616457, 93.03053543526598901, 59.99999999999999289 ) ) ;
#61081=DIRECTION ( 'NONE',  ( 0.000000000000000000, -0.000000000000000000, 1.000000000000000000 ) ) ;
#61083=CARTESIAN_POINT ( 'NONE',  ( -19.65312891409030271, 93.06504152958497400, 177.5919119679930134 ) ) ;
#61085=VERTEX_POINT ( 'NONE', #87008 ) ;
#61095=DIRECTION ( 'NONE',  ( 0.000000000000000000, 0.000000000000000000, 1.000000000000000000 ) ) ;
#61096=AXIS2_PLACEMENT_3D ( 'NONE', #67168, #37262, #14948 ) ;
#61100=ORIENTED_EDGE ( 'NONE', *, *, #54772, .F. ) ;
#61102=EDGE_CURVE ( 'NONE', #75897, #91070, #33235, .T. ) ;
#61106=DIRECTION ( 'NONE',  ( 0.9403255362191060840, -0.3402761906661271873, 0.000000000000000000 ) ) ;
#61112=DIRECTION ( 'NONE',  ( -0.8660254037844380415, -0.5000000000000011102, 0.000000000000000000 ) ) ;
#61116=ORIENTED_EDGE ( 'NONE', *, *, #7740, .T. ) ;
#61134=CARTESIAN_POINT ( 'NONE',  ( 44.35815684012577265, 67.96982248125696913, -10.00000000000000000 ) ) ;
#61136=DIRECTION ( 'NONE',  ( -1.000000000000000000, 0.000000000000000000, 0.000000000000000000 ) ) ;
#61137=VECTOR ( 'NONE', #11498, 1000.000000000000000 ) ;
#61138=VERTEX_POINT ( 'NONE', #6801 ) ;
#61139=VECTOR ( 'NONE', #33582, 1000.000000000000227 ) ;
#61145=CARTESIAN_POINT ( 'NONE',  ( 47.32807415326522715, 108.5480133836684900, -10.00000000000000000 ) ) ;
#61150=ORIENTED_EDGE ( 'NONE', *, *, #79651, .T. ) ;
#61151=CARTESIAN_POINT ( 'NONE',  ( -19.65312891409030271, 93.06504152958497400, 59.99999999999999289 ) ) ;
#61152=FACE_OUTER_BOUND ( 'NONE', #49059, .T. ) ;
#61168=LINE ( 'NONE', #84520, #51320 ) ;
#61171=CARTESIAN_POINT ( 'NONE',  ( -19.65312891409030271, 93.06504152958497400, 177.5919119679930134 ) ) ;
#61172=DIRECTION ( 'NONE',  ( 0.9263643838751153270, 0.3766285016932175433, 0.000000000000000000 ) ) ;
#61176=EDGE_CURVE ( 'NONE', #70394, #17777, #26872, .T. ) ;
#61193=VECTOR ( 'NONE', #77102, 1000.000000000000114 ) ;
#61197=VECTOR ( 'NONE', #8153, 1000.000000000000000 ) ;
#61201=AXIS2_PLACEMENT_3D ( 'NONE', #93876, #62408, #54819 ) ;
#61230=DIRECTION ( 'NONE',  ( 1.000000000000000000, 0.000000000000000000, 0.000000000000000000 ) ) ;
#61231=VERTEX_POINT ( 'NONE', #81603 ) ;
#61238=LINE ( 'NONE', #55626, #62656 ) ;
#61251=ORIENTED_EDGE ( 'NONE', *, *, #26198, .T. ) ;
#61253=DIRECTION ( 'NONE',  ( -0.000000000000000000, -0.000000000000000000, -1.000000000000000000 ) ) ;
#61255=ORIENTED_EDGE ( 'NONE', *, *, #9088, .T. ) ;
#61256=DIRECTION ( 'NONE',  ( 0.5280678506503729830, 0.8492021815265757834, 0.000000000000000000 ) ) ;
#61258=FACE_BOUND ( 'NONE', #34579, .T. ) ;
#61278=VECTOR ( 'NONE', #38472, 1000.000000000000000 ) ;
#61302=AXIS2_PLACEMENT_3D ( 'NONE', #16228, #39497, #69913 ) ;
#61309=CARTESIAN_POINT ( 'NONE',  ( 48.77433535142598231, 99.76555324011610537, -10.00000000000000000 ) ) ;
#61318=EDGE_CURVE ( 'NONE', #31684, #71618, #35458, .T. ) ;
#61329=VECTOR ( 'NONE', #16369, 1000.000000000000000 ) ;
#61332=ADVANCED_FACE ( 'NONE', ( #66361 ), #27370, .F. ) ;
#61346=ORIENTED_EDGE ( 'NONE', *, *, #45048, .F. ) ;
#61347=AXIS2_PLACEMENT_3D ( 'NONE', #50956, #35265, #27684 ) ;
#61349=FACE_OUTER_BOUND ( 'NONE', #13472, .T. ) ;
#61355=CARTESIAN_POINT ( 'NONE',  ( -10.80656490723494123, 24.88181024604954672, -10.00000000000000000 ) ) ;
#61357=FACE_OUTER_BOUND ( 'NONE', #100269, .T. ) ;
#61360=AXIS2_PLACEMENT_3D ( 'NONE', #7055, #28361, #29862 ) ;
#61367=CARTESIAN_POINT ( 'NONE',  ( -30.18034446749236821, 25.12100238203590763, -10.00000000000000000 ) ) ;
#61368=ORIENTED_EDGE ( 'NONE', *, *, #47988, .T. ) ;
#61370=VECTOR ( 'NONE', #93276, 1000.000000000000000 ) ;
#61376=ADVANCED_FACE ( 'NONE', ( #27861 ), #11683, .F. ) ;
#61382=CARTESIAN_POINT ( 'NONE',  ( 29.30989995549245464, 44.80713248141895377, 10.00000000000000000 ) ) ;
#61387=LINE ( 'NONE', #38075, #42816 ) ;
#61393=EDGE_CURVE ( 'NONE', #52271, #46169, #51667, .T. ) ;
#61402=ORIENTED_EDGE ( 'NONE', *, *, #98372, .F. ) ;
#61422=CARTESIAN_POINT ( 'NONE',  ( -19.65312891409030271, 93.06504152958497400, -10.00000000000000888 ) ) ;
#61424=VERTEX_POINT ( 'NONE', #75469 ) ;
#61425=LINE ( 'NONE', #47228, #42974 ) ;
#61430=CARTESIAN_POINT ( 'NONE',  ( -6.281727404287059890, 25.63055774385195207, -10.00000000000000000 ) ) ;
#61440=ADVANCED_FACE ( 'NONE', ( #44536 ), #67860, .F. ) ;
#61466=ORIENTED_EDGE ( 'NONE', *, *, #989, .T. ) ;
#61468=( NAMED_UNIT ( * ) SI_UNIT ( $, .STERADIAN. ) SOLID_ANGLE_UNIT ( ) );
#61470=LINE ( 'NONE', #76209, #85583 ) ;
#61472=ORIENTED_EDGE ( 'NONE', *, *, #3104, .F. ) ;
#61474=CARTESIAN_POINT ( 'NONE',  ( -59.75159773472199021, 60.38055040163846598, 59.99999999999999289 ) ) ;
#61478=CARTESIAN_POINT ( 'NONE',  ( -48.47243291925848752, 30.64988553008148031, -10.00000000000000000 ) ) ;
#61489=ORIENTED_EDGE ( 'NONE', *, *, #34851, .T. ) ;
#61490=VECTOR ( 'NONE', #46856, 1000.000000000000114 ) ;
#61491=DIRECTION ( 'NONE',  ( 0.09274582908232943679, 0.9956898167541091693, 0.000000000000000000 ) ) ;
#61492=LINE ( 'NONE', #69094, #39479 ) ;
#61495=VERTEX_POINT ( 'NONE', #46530 ) ;
#61506=ORIENTED_EDGE ( 'NONE', *, *, #43172, .F. ) ;
#61524=EDGE_CURVE ( 'NONE', #68209, #74106, #61238, .T. ) ;
#61527=EDGE_CURVE ( 'NONE', #61138, #43154, #39923, .T. ) ;
#61529=CARTESIAN_POINT ( 'NONE',  ( 15.94180138266918689, 46.41934012499306306, 59.99999999999999289 ) ) ;
#61533=ORIENTED_EDGE ( 'NONE', *, *, #4114, .F. ) ;
#61539=DIRECTION ( 'NONE',  ( -1.000000000000000000, 0.000000000000000000, -0.000000000000000000 ) ) ;
#61546=EDGE_LOOP ( 'NONE', ( #60864, #50809, #67728, #9747 ) ) ;
#61547=DIRECTION ( 'NONE',  ( 0.000000000000000000, 0.000000000000000000, 1.000000000000000000 ) ) ;
#61548=CARTESIAN_POINT ( 'NONE',  ( 26.18314342202568668, 41.82794442100486521, 10.00000000000000000 ) ) ;
#61555=DIRECTION ( 'NONE',  ( -1.000000000000000000, 0.000000000000000000, 0.000000000000000000 ) ) ;
#61563=CARTESIAN_POINT ( 'NONE',  ( -19.65312891409030271, 93.06504152958497400, -10.00000000000000888 ) ) ;
#61576=EDGE_CURVE ( 'NONE', #10473, #10907, #1468, .T. ) ;
#61577=FACE_OUTER_BOUND ( 'NONE', #51842, .T. ) ;
#61582=CARTESIAN_POINT ( 'NONE',  ( -69.61464189717713680, 45.83092310410447112, 10.00000000000000000 ) ) ;
#61586=ORIENTED_EDGE ( 'NONE', *, *, #92315, .F. ) ;
#61591=ADVANCED_FACE ( 'NONE', ( #15129 ), #54628, .F. ) ;
#61599=ORIENTED_EDGE ( 'NONE', *, *, #80736, .F. ) ;
#61602=ORIENTED_EDGE ( 'NONE', *, *, #45891, .F. ) ;
#61617=EDGE_LOOP ( 'NONE', ( #96926, #44415, #21410, #3627 ) ) ;
#61621=EDGE_CURVE ( 'NONE', #87203, #3988, #49058, .T. ) ;
#61623=CARTESIAN_POINT ( 'NONE',  ( 45.80758703142363686, 72.03864405183792030, -10.00000000000000000 ) ) ;
#61630=ADVANCED_FACE ( 'NONE', ( #17659 ), #10560, .T. ) ;
#61632=ADVANCED_FACE ( 'NONE', ( #65733 ), #2469, .F. ) ;
#61643=PLANE ( 'NONE',  #81952 ) ;
#61646=LINE ( 'NONE', #30765, #23825 ) ;
#61650=CIRCLE ( 'NONE', #81167, 0.1418229129680828593 ) ;
#61654=EDGE_LOOP ( 'NONE', ( #91445, #60495, #25844, #12302 ) ) ;
#61665=CARTESIAN_POINT ( 'NONE',  ( -29.63305522156611005, 61.36453520006032392, -10.00000000000000000 ) ) ;
#61671=DIRECTION ( 'NONE',  ( -0.000000000000000000, -0.000000000000000000, -1.000000000000000000 ) ) ;
#61675=CARTESIAN_POINT ( 'NONE',  ( 44.35815684012577265, 67.96982248125696913, 10.00000000000000000 ) ) ;
#61708=EDGE_CURVE ( 'NONE', #14070, #58863, #12058, .T. ) ;
#61717=ORIENTED_EDGE ( 'NONE', *, *, #65951, .T. ) ;
#61724=EDGE_LOOP ( 'NONE', ( #23116, #6855, #76686, #13769 ) ) ;
#61732=PLANE ( 'NONE',  #76016 ) ;
#61736=CARTESIAN_POINT ( 'NONE',  ( -2.330697855141256269, 26.52822386297705393, -10.00000000000000000 ) ) ;
#61737=DIRECTION ( 'NONE',  ( 0.7490285521785712275, -0.6625377181876314081, 0.000000000000000000 ) ) ;
#61738=ORIENTED_EDGE ( 'NONE', *, *, #65687, .T. ) ;
#61739=LINE ( 'NONE', #38939, #84809 ) ;
#61754=CARTESIAN_POINT ( 'NONE',  ( -19.65312891409030271, 93.06504152958497400, 10.00000000000000888 ) ) ;
#61758=VERTEX_POINT ( 'NONE', #53026 ) ;
#61760=EDGE_CURVE ( 'NONE', #69710, #20188, #35341, .T. ) ;
#61762=CARTESIAN_POINT ( 'NONE',  ( -74.22192597045216189, 49.22161114575668250, 10.00000000000000000 ) ) ;
#61764=DIRECTION ( 'NONE',  ( 0.000000000000000000, 0.000000000000000000, 1.000000000000000000 ) ) ;
#61779=DIRECTION ( 'NONE',  ( -0.000000000000000000, 0.000000000000000000, -1.000000000000000000 ) ) ;
#61787=EDGE_LOOP ( 'NONE', ( #77461, #87032, #71176, #20092 ) ) ;
#61794=VERTEX_POINT ( 'NONE', #82981 ) ;
#61803=CARTESIAN_POINT ( 'NONE',  ( -19.65312891409030271, 93.06504152958497400, -10.00000000000000888 ) ) ;
#61815=LINE ( 'NONE', #29439, #56033 ) ;
#61825=CARTESIAN_POINT ( 'NONE',  ( 49.51900556837681222, 105.3795262313705763, -10.00000000000000000 ) ) ;
#61842=FACE_OUTER_BOUND ( 'NONE', #79892, .T. ) ;
#61849=DIRECTION ( 'NONE',  ( -1.000000000000000000, 0.000000000000000000, 0.000000000000000000 ) ) ;
#61859=LINE ( 'NONE', #30970, #32152 ) ;
#61870=CARTESIAN_POINT ( 'NONE',  ( -4.866515740870070772, 77.03598506094434128, 14.21757578985110193 ) ) ;
#61872=CARTESIAN_POINT ( 'NONE',  ( -50.36082798260552806, 30.16005589317048674, -10.00000000000000000 ) ) ;
#61874=ORIENTED_EDGE ( 'NONE', *, *, #16607, .T. ) ;
#61877=CARTESIAN_POINT ( 'NONE',  ( -32.04500338604974985, 25.44370296803430520, -10.00000000000000000 ) ) ;
#61883=EDGE_CURVE ( 'NONE', #93683, #32652, #28743, .T. ) ;
#61894=VERTEX_POINT ( 'NONE', #38816 ) ;
#61897=CARTESIAN_POINT ( 'NONE',  ( -21.43592214265774132, 59.87855815223608147, -10.00000000000000000 ) ) ;
#61898=VECTOR ( 'NONE', #90451, 1000.000000000000000 ) ;
#61910=VECTOR ( 'NONE', #2635, 1000.000000000000000 ) ;
#61916=ORIENTED_EDGE ( 'NONE', *, *, #82743, .F. ) ;
#61946=CARTESIAN_POINT ( 'NONE',  ( -19.65312891409030271, 93.06504152958497400, 10.00000000000000888 ) ) ;
#61956=DIRECTION ( 'NONE',  ( -0.1580495287025880657, -0.9874311856918890351, 0.000000000000000000 ) ) ;
#61958=ORIENTED_EDGE ( 'NONE', *, *, #89686, .F. ) ;
#61961=CARTESIAN_POINT ( 'NONE',  ( -61.08640853961129835, 36.64444830801922848, 177.5919119679930134 ) ) ;
#61975=VECTOR ( 'NONE', #66099, 1000.000000000000000 ) ;
#61983=ORIENTED_EDGE ( 'NONE', *, *, #73005, .F. ) ;
#61985=ORIENTED_EDGE ( 'NONE', *, *, #61524, .T. ) ;
#62009=DIRECTION ( 'NONE',  ( 0.000000000000000000, 0.000000000000000000, 1.000000000000000000 ) ) ;
#62011=EDGE_CURVE ( 'NONE', #79361, #22484, #31703, .T. ) ;
#62017=CARTESIAN_POINT ( 'NONE',  ( -19.65312891409030271, 93.06504152958497400, 40.00000000000000000 ) ) ;
#62027=AXIS2_PLACEMENT_3D ( 'NONE', #53000, #21617, #12028 ) ;
#62029=ORIENTED_EDGE ( 'NONE', *, *, #45472, .T. ) ;
#62038=DIRECTION ( 'NONE',  ( 0.000000000000000000, 0.000000000000000000, 1.000000000000000000 ) ) ;
#62039=ORIENTED_EDGE ( 'NONE', *, *, #82639, .F. ) ;
#62058=CARTESIAN_POINT ( 'NONE',  ( -31.59160691316810343, 24.09060609829247568, 10.00000000000000000 ) ) ;
#62059=ADVANCED_FACE ( 'NONE', ( #3358 ), #80376, .F. ) ;
#62067=DIRECTION ( 'NONE',  ( 0.8434505012732891327, -0.5372068985985168910, 0.000000000000000000 ) ) ;
#62082=EDGE_CURVE ( 'NONE', #13459, #68842, #33226, .T. ) ;
#62089=ORIENTED_EDGE ( 'NONE', *, *, #43563, .F. ) ;
#62093=DIRECTION ( 'NONE',  ( 1.000000000000000000, 0.000000000000000000, 0.000000000000000000 ) ) ;
#62098=FACE_OUTER_BOUND ( 'NONE', #69975, .T. ) ;
#62109=ORIENTED_EDGE ( 'NONE', *, *, #35552, .F. ) ;
#62116=CARTESIAN_POINT ( 'NONE',  ( 48.98810889288134973, 89.24608170897542436, -10.00000000000000000 ) ) ;
#62118=CARTESIAN_POINT ( 'NONE',  ( -65.03992292888629834, 39.77302590755693501, 177.5919119679930134 ) ) ;
#62126=DIRECTION ( 'NONE',  ( 1.000000000000000000, 0.000000000000000000, 0.000000000000000000 ) ) ;
#62135=EDGE_LOOP ( 'NONE', ( #56675, #60931, #90709, #23509 ) ) ;
#62137=LINE ( 'NONE', #12720, #4395 ) ;
#62169=CARTESIAN_POINT ( 'NONE',  ( 47.49582885874515625, 78.29235751436857527, -10.00000000000000000 ) ) ;
#62179=CARTESIAN_POINT ( 'NONE',  ( 35.15122015938992917, 74.24965902719526412, 59.99999999999999289 ) ) ;
#62180=VECTOR ( 'NONE', #75427, 1000.000000000000000 ) ;
#62181=EDGE_CURVE ( 'NONE', #25628, #52271, #97074, .T. ) ;
#62184=FACE_OUTER_BOUND ( 'NONE', #78830, .T. ) ;
#62185=VECTOR ( 'NONE', #96691, 1000.000000000000000 ) ;
#62206=DIRECTION ( 'NONE',  ( 0.9997716407803077798, -0.02136975178731510827, 0.000000000000000000 ) ) ;
#62208=ORIENTED_EDGE ( 'NONE', *, *, #74348, .F. ) ;
#62209=CARTESIAN_POINT ( 'NONE',  ( 48.53010236944518851, 101.9116055364396090, 10.00000000000000000 ) ) ;
#62211=ORIENTED_EDGE ( 'NONE', *, *, #2526, .F. ) ;
#62216=PLANE ( 'NONE',  #28912 ) ;
#62224=LINE ( 'NONE', #93176, #95426 ) ;
#62226=VERTEX_POINT ( 'NONE', #95905 ) ;
#62233=DIRECTION ( 'NONE',  ( -0.000000000000000000, -0.000000000000000000, -1.000000000000000000 ) ) ;
#62235=FACE_OUTER_BOUND ( 'NONE', #85720, .T. ) ;
#62241=ORIENTED_EDGE ( 'NONE', *, *, #19789, .T. ) ;
#62248=VERTEX_POINT ( 'NONE', #48765 ) ;
#62257=ORIENTED_EDGE ( 'NONE', *, *, #3849, .T. ) ;
#62259=VERTEX_POINT ( 'NONE', #42628 ) ;
#62261=AXIS2_PLACEMENT_3D ( 'NONE', #12280, #82714, #97389 ) ;
#62262=ADVANCED_FACE ( 'NONE', ( #96389 ), #73557, .F. ) ;
#62267=CARTESIAN_POINT ( 'NONE',  ( -19.65312891409030271, 93.06504152958497400, 177.5919119679930134 ) ) ;
#62275=EDGE_CURVE ( 'NONE', #14058, #62875, #57339, .T. ) ;
#62284=CARTESIAN_POINT ( 'NONE',  ( -19.65312891409030271, 93.06504152958497400, 59.99999999999999289 ) ) ;
#62290=DIRECTION ( 'NONE',  ( -0.000000000000000000, 0.000000000000000000, 1.000000000000000000 ) ) ;
#62296=DIRECTION ( 'NONE',  ( 1.000000000000000000, 0.000000000000000000, 0.000000000000000000 ) ) ;
#62301=VERTEX_POINT ( 'NONE', #57836 ) ;
#62307=CARTESIAN_POINT ( 'NONE',  ( -61.61048871844075592, 38.59675092633816007, -10.00000000000000000 ) ) ;
#62315=CIRCLE ( 'NONE', #85016, 0.1418229129684263345 ) ;
#62319=DIRECTION ( 'NONE',  ( 1.000000000000000000, -7.137148015447434001E-15, 0.000000000000000000 ) ) ;
#62327=CARTESIAN_POINT ( 'NONE',  ( 50.00170217996128486, 86.12209509027381671, 177.5919119679930134 ) ) ;
#62332=DIRECTION ( 'NONE',  ( -0.9403255362191098587, 0.3402761906661169733, 0.000000000000000000 ) ) ;
#62336=DIRECTION ( 'NONE',  ( -1.000000000000000000, 0.000000000000000000, 0.000000000000000000 ) ) ;
#62341=ORIENTED_EDGE ( 'NONE', *, *, #34632, .T. ) ;
#62350=ORIENTED_EDGE ( 'NONE', *, *, #51786, .F. ) ;
#62352=FACE_OUTER_BOUND ( 'NONE', #77114, .T. ) ;
#62359=CARTESIAN_POINT ( 'NONE',  ( 19.39689925177878749, 34.96947112835014337, 177.5919119679930134 ) ) ;
#62371=EDGE_LOOP ( 'NONE', ( #1170, #76600, #27964, #96459 ) ) ;
#62372=ORIENTED_EDGE ( 'NONE', *, *, #11655, .T. ) ;
#62380=FACE_OUTER_BOUND ( 'NONE', #45651, .T. ) ;
#62394=EDGE_CURVE ( 'NONE', #76267, #40576, #6135, .T. ) ;
#62397=EDGE_CURVE ( 'NONE', #61231, #39956, #52228, .T. ) ;
#62403=CARTESIAN_POINT ( 'NONE',  ( -75.57215499213535281, 50.95729256953105590, 177.5919119679930134 ) ) ;
#62405=CARTESIAN_POINT ( 'NONE',  ( 27.58098951138967436, 43.10352854649765675, 10.00000000000000000 ) ) ;
#62408=DIRECTION ( 'NONE',  ( 0.000000000000000000, 0.000000000000000000, 1.000000000000000000 ) ) ;
#62413=DIRECTION ( 'NONE',  ( -0.000000000000000000, 0.000000000000000000, -1.000000000000000000 ) ) ;
#62414=CARTESIAN_POINT ( 'NONE',  ( -36.26652983198114555, 26.35523046909639788, -10.00000000000000000 ) ) ;
#62425=AXIS2_PLACEMENT_3D ( 'NONE', #100187, #52555, #22169 ) ;
#62437=VECTOR ( 'NONE', #48951, 1000.000000000000114 ) ;
#62448=DIRECTION ( 'NONE',  ( 0.000000000000000000, 0.000000000000000000, 1.000000000000000000 ) ) ;
#62456=VECTOR ( 'NONE', #38583, 1000.000000000000227 ) ;
#62458=CARTESIAN_POINT ( 'NONE',  ( -15.61417992190811077, 23.18166087982998391, 177.5919119679930134 ) ) ;
#62461=CARTESIAN_POINT ( 'NONE',  ( -19.65312891409030271, 93.06504152958497400, 177.5919119679930134 ) ) ;
#62466=LINE ( 'NONE', #26010, #42202 ) ;
#62476=CARTESIAN_POINT ( 'NONE',  ( -19.56945998093726047, 92.95052843746097437, 59.99999999999999289 ) ) ;
#62484=ORIENTED_EDGE ( 'NONE', *, *, #95995, .F. ) ;
#62485=ORIENTED_EDGE ( 'NONE', *, *, #86480, .T. ) ;
#62488=DIRECTION ( 'NONE',  ( -0.9874733399847777093, -0.1577859398657163736, 0.000000000000000000 ) ) ;
#62495=DIRECTION ( 'NONE',  ( 0.000000000000000000, 0.000000000000000000, 1.000000000000000000 ) ) ;
#62503=ORIENTED_EDGE ( 'NONE', *, *, #95305, .T. ) ;
#62518=CARTESIAN_POINT ( 'NONE',  ( -46.31994871380127421, 28.06264584988120347, 10.00000000000000000 ) ) ;
#62533=ORIENTED_EDGE ( 'NONE', *, *, #55089, .F. ) ;
#62547=DIRECTION ( 'NONE',  ( 0.000000000000000000, 0.000000000000000000, 1.000000000000000000 ) ) ;
#62559=DIRECTION ( 'NONE',  ( 0.000000000000000000, 0.000000000000000000, 1.000000000000000000 ) ) ;
#62560=DIRECTION ( 'NONE',  ( 0.2091919045418403900, 0.9778746070300412541, 0.000000000000000000 ) ) ;
#62564=FACE_OUTER_BOUND ( 'NONE', #84517, .T. ) ;
#62569=CARTESIAN_POINT ( 'NONE',  ( -19.65312891409030271, 93.06504152958497400, 10.00000000000000888 ) ) ;
#62571=EDGE_CURVE ( 'NONE', #25248, #1860, #25851, .T. ) ;
#62572=LINE ( 'NONE', #94036, #88032 ) ;
#62580=ORIENTED_EDGE ( 'NONE', *, *, #93453, .T. ) ;
#62588=CIRCLE ( 'NONE', #96643, 70.00000000000001421 ) ;
#62594=ORIENTED_EDGE ( 'NONE', *, *, #41133, .T. ) ;
#62597=DIRECTION ( 'NONE',  ( -0.8660254037844380415, -0.5000000000000009992, 0.000000000000000000 ) ) ;
#62605=VECTOR ( 'NONE', #81495, 1000.000000000000000 ) ;
#62608=VERTEX_POINT ( 'NONE', #27339 ) ;
#62615=ORIENTED_EDGE ( 'NONE', *, *, #17566, .F. ) ;
#62627=VERTEX_POINT ( 'NONE', #58220 ) ;
#62630=EDGE_CURVE ( 'NONE', #77358, #11342, #12646, .T. ) ;
#62632=PLANE ( 'NONE',  #88489 ) ;
#62635=CARTESIAN_POINT ( 'NONE',  ( 41.50249547274756878, 124.4848494355456836, -10.00000000000000000 ) ) ;
#62638=LINE ( 'NONE', #86520, #38368 ) ;
#62651=DIRECTION ( 'NONE',  ( -0.7511915808658203852, -0.6600842437418951159, 0.000000000000000000 ) ) ;
#62656=VECTOR ( 'NONE', #92203, 1000.000000000000000 ) ;
#62661=CARTESIAN_POINT ( 'NONE',  ( 9.242171499132833645, 29.30720582267293750, -10.00000000000000000 ) ) ;
#62670=DIRECTION ( 'NONE',  ( 0.6833540297821638632, -0.7300871660154544251, 0.000000000000000000 ) ) ;
#62672=DIRECTION ( 'NONE',  ( 1.000000000000000000, 0.000000000000000000, 0.000000000000000000 ) ) ;
#62687=AXIS2_PLACEMENT_3D ( 'NONE', #69307, #52596, #21226 ) ;
#62702=LINE ( 'NONE', #40401, #70434 ) ;
#62705=CARTESIAN_POINT ( 'NONE',  ( -33.75225536883274913, 24.49963747467413810, 10.00000000000000000 ) ) ;
#62706=EDGE_CURVE ( 'NONE', #24773, #16945, #85052, .T. ) ;
#62710=VERTEX_POINT ( 'NONE', #45992 ) ;
#62719=VERTEX_POINT ( 'NONE', #18126 ) ;
#62729=CARTESIAN_POINT ( 'NONE',  ( -15.61417992190811788, 23.18166087982996970, 10.00000000000000000 ) ) ;
#62733=ADVANCED_FACE ( 'NONE', ( #25736 ), #1434, .F. ) ;
#62736=DIRECTION ( 'NONE',  ( 0.3851501363289905333, -0.9228539280329037808, 0.000000000000000000 ) ) ;
#62751=CARTESIAN_POINT ( 'NONE',  ( -64.74139798177010618, 41.16849083240310847, -10.00000000000000000 ) ) ;
#62755=ORIENTED_EDGE ( 'NONE', *, *, #62181, .T. ) ;
#62760=LINE ( 'NONE', #16672, #4610 ) ;
#62766=VECTOR ( 'NONE', #33221, 1000.000000000000000 ) ;
#62767=ORIENTED_EDGE ( 'NONE', *, *, #58669, .F. ) ;
#62776=CARTESIAN_POINT ( 'NONE',  ( 22.87549206224920084, 39.05096577487528720, 10.00000000000000000 ) ) ;
#62784=FACE_OUTER_BOUND ( 'NONE', #84309, .T. ) ;
#62788=CARTESIAN_POINT ( 'NONE',  ( -19.15453390681661716, 24.31945705462846163, -10.00000000000000000 ) ) ;
#62789=ORIENTED_EDGE ( 'NONE', *, *, #45572, .F. ) ;
#62799=CIRCLE ( 'NONE', #51459, 0.1418229129684228651 ) ;
#62807=DIRECTION ( 'NONE',  ( 0.09248003802711829424, -0.9957145386939485476, 0.000000000000000000 ) ) ;
#62810=VECTOR ( 'NONE', #14300, 1000.000000000000000 ) ;
#62813=ORIENTED_EDGE ( 'NONE', *, *, #68461, .F. ) ;
#62836=EDGE_CURVE ( 'NONE', #73010, #36208, #2440, .T. ) ;
#62846=VERTEX_POINT ( 'NONE', #71337 ) ;
#62858=ORIENTED_EDGE ( 'NONE', *, *, #88511, .F. ) ;
#62861=ORIENTED_EDGE ( 'NONE', *, *, #8000, .T. ) ;
#62863=CIRCLE ( 'NONE', #70993, 70.00000000000001421 ) ;
#62873=AXIS2_PLACEMENT_3D ( 'NONE', #17131, #32830, #69829 ) ;
#62875=VERTEX_POINT ( 'NONE', #84318 ) ;
#62885=VERTEX_POINT ( 'NONE', #29094 ) ;
#62886=CIRCLE ( 'NONE', #90428, 70.00000000000001421 ) ;
#62892=ORIENTED_EDGE ( 'NONE', *, *, #93761, .T. ) ;
#62904=CARTESIAN_POINT ( 'NONE',  ( 45.66470909604093720, 114.5311720768849995, -10.00000000000000000 ) ) ;
#62925=CARTESIAN_POINT ( 'NONE',  ( 42.76202708541288899, 64.24573752441608576, -10.00000000000000000 ) ) ;
#62934=CARTESIAN_POINT ( 'NONE',  ( -5.362061845104276081, 24.53938646500537146, -10.00000000000000000 ) ) ;
#62937=VECTOR ( 'NONE', #77763, 1000.000000000000000 ) ;
#62939=ORIENTED_EDGE ( 'NONE', *, *, #71320, .T. ) ;
#62940=ADVANCED_FACE ( 'NONE', ( #82341 ), #97995, .F. ) ;
#62943=VECTOR ( 'NONE', #26680, 1000.000000000000000 ) ;
#62948=DIRECTION ( 'NONE',  ( -0.000000000000000000, -0.000000000000000000, -1.000000000000000000 ) ) ;
#62958=AXIS2_PLACEMENT_3D ( 'NONE', #66488, #28480, #11327 ) ;
#62968=EDGE_CURVE ( 'NONE', #35128, #46853, #74712, .T. ) ;
#62973=CARTESIAN_POINT ( 'NONE',  ( -19.42194755839791753, 24.31068691715150010, -10.00000000000000000 ) ) ;
#62981=EDGE_CURVE ( 'NONE', #28238, #29044, #52371, .T. ) ;
#62985=EDGE_CURVE ( 'NONE', #67772, #63278, #5776, .T. ) ;
#62988=ORIENTED_EDGE ( 'NONE', *, *, #74365, .T. ) ;
#62994=CARTESIAN_POINT ( 'NONE',  ( -5.362061845104276081, 24.53938646500537146, 10.00000000000000000 ) ) ;
#62995=DIRECTION ( 'NONE',  ( -1.000000000000000000, 0.000000000000000000, 0.000000000000000000 ) ) ;
#63009=ORIENTED_EDGE ( 'NONE', *, *, #90829, .T. ) ;
#63013=VERTEX_POINT ( 'NONE', #1691 ) ;
#63015=EDGE_CURVE ( 'NONE', #74347, #14902, #93917, .T. ) ;
#63019=VECTOR ( 'NONE', #49890, 1000.000000000000000 ) ;
#63021=DIRECTION ( 'NONE',  ( -0.000000000000000000, -0.000000000000000000, -1.000000000000000000 ) ) ;
#63026=AXIS2_PLACEMENT_3D ( 'NONE', #28170, #83402, #90524 ) ;
#63037=ORIENTED_EDGE ( 'NONE', *, *, #98689, .T. ) ;
#63040=CARTESIAN_POINT ( 'NONE',  ( -58.10760318826260118, 36.06970723555269842, 10.00000000000000000 ) ) ;
#63045=CARTESIAN_POINT ( 'NONE',  ( 45.05588048050944394, 66.36777381976860113, -10.00000000000000000 ) ) ;
#63052=VERTEX_POINT ( 'NONE', #33071 ) ;
#63056=CIRCLE ( 'NONE', #32320, 70.00000000000001421 ) ;
#63078=ORIENTED_EDGE ( 'NONE', *, *, #48859, .F. ) ;
#63084=CARTESIAN_POINT ( 'NONE',  ( -19.65312891409030271, 93.06504152958497400, 177.5919119679930134 ) ) ;
#63092=DIRECTION ( 'NONE',  ( -0.000000000000000000, 0.000000000000000000, -1.000000000000000000 ) ) ;
#63093=ORIENTED_EDGE ( 'NONE', *, *, #80875, .T. ) ;
#63103=VECTOR ( 'NONE', #44851, 1000.000000000000000 ) ;
#63105=ORIENTED_EDGE ( 'NONE', *, *, #80451, .T. ) ;
#63113=EDGE_CURVE ( 'NONE', #44653, #74347, #50752, .T. ) ;
#63119=LINE ( 'NONE', #57383, #94680 ) ;
#63120=LINE ( 'NONE', #24120, #62766 ) ;
#63121=CYLINDRICAL_SURFACE ( 'NONE', #38088, 45.00000000000000000 ) ;
#63138=CARTESIAN_POINT ( 'NONE',  ( -53.24159167507352208, 52.03622613587658208, 59.99999999999999289 ) ) ;
#63146=ORIENTED_EDGE ( 'NONE', *, *, #71672, .F. ) ;
#63149=LINE ( 'NONE', #16052, #7486 ) ;
#63162=AXIS2_PLACEMENT_3D ( 'NONE', #23092, #30712, #7397 ) ;
#63179=CIRCLE ( 'NONE', #58323, 0.1418229129680863287 ) ;
#63184=LINE ( 'NONE', #61675, #29806 ) ;
#63209=LINE ( 'NONE', #76901, #52204 ) ;
#63221=ADVANCED_FACE ( 'NONE', ( #67955 ), #45144, .F. ) ;
#63234=ADVANCED_FACE ( 'NONE', ( #90309 ), #29453, .F. ) ;
#63242=DIRECTION ( 'NONE',  ( -0.8452030915256492083, -0.5344452582589588330, 0.000000000000000000 ) ) ;
#63260=LINE ( 'NONE', #9582, #72824 ) ;
#63270=ORIENTED_EDGE ( 'NONE', *, *, #42849, .T. ) ;
#63278=VERTEX_POINT ( 'NONE', #99369 ) ;
#63279=CARTESIAN_POINT ( 'NONE',  ( -19.75605576492141324, 93.16261100237599635, 59.99999999999999289 ) ) ;
#63291=EDGE_CURVE ( 'NONE', #37083, #9585, #51769, .T. ) ;
#63292=DIRECTION ( 'NONE',  ( -0.9607486656258009683, -0.2774202615135436534, 0.000000000000000000 ) ) ;
#63297=CARTESIAN_POINT ( 'NONE',  ( -71.61465314115659453, 63.06504152958490295, 10.00000000000000888 ) ) ;
#63303=EDGE_CURVE ( 'NONE', #21633, #66853, #82711, .T. ) ;
#63305=ORIENTED_EDGE ( 'NONE', *, *, #92013, .T. ) ;
#63312=EDGE_CURVE ( 'NONE', #31364, #76961, #10999, .T. ) ;
#63327=DIRECTION ( 'NONE',  ( -0.000000000000000000, -0.000000000000000000, 1.000000000000000000 ) ) ;
#63336=DIRECTION ( 'NONE',  ( 0.9874311856918873698, -0.1580495287025983631, 0.000000000000000000 ) ) ;
#63337=EDGE_CURVE ( 'NONE', #15749, #38318, #52733, .T. ) ;
#63346=CARTESIAN_POINT ( 'NONE',  ( 45.56181175559624563, 118.5014625327306135, 10.00000000000000000 ) ) ;
#63348=EDGE_CURVE ( 'NONE', #26065, #5345, #17401, .T. ) ;
#63353=CARTESIAN_POINT ( 'NONE',  ( -17.26243516413818924, 24.35187462261283997, -10.00000000000000000 ) ) ;
#63358=ORIENTED_EDGE ( 'NONE', *, *, #6276, .F. ) ;
#63363=EDGE_CURVE ( 'NONE', #72251, #98005, #24839, .T. ) ;
#63370=VERTEX_POINT ( 'NONE', #63346 ) ;
#63373=CARTESIAN_POINT ( 'NONE',  ( 28.00427808217457937, 41.79349426999505113, 177.5919119679930134 ) ) ;
#63374=ORIENTED_EDGE ( 'NONE', *, *, #47420, .T. ) ;
#63382=ORIENTED_EDGE ( 'NONE', *, *, #47322, .F. ) ;
#63399=CARTESIAN_POINT ( 'NONE',  ( -19.65312891409030271, 93.06504152958497400, -10.00000000000000888 ) ) ;
#63400=VERTEX_POINT ( 'NONE', #70443 ) ;
#63407=ADVANCED_FACE ( 'NONE', ( #17238 ), #79088, .T. ) ;
#63422=ORIENTED_EDGE ( 'NONE', *, *, #84540, .T. ) ;
#63436=LINE ( 'NONE', #54824, #28634 ) ;
#63440=EDGE_CURVE ( 'NONE', #39976, #81025, #64856, .T. ) ;
#63462=ORIENTED_EDGE ( 'NONE', *, *, #11655, .F. ) ;
#63471=DIRECTION ( 'NONE',  ( -0.000000000000000000, -0.000000000000000000, -1.000000000000000000 ) ) ;
#63491=ORIENTED_EDGE ( 'NONE', *, *, #90513, .F. ) ;
#63492=DIRECTION ( 'NONE',  ( -0.4527707594502665689, -0.8916269620120450545, 0.000000000000000000 ) ) ;
#63494=VERTEX_POINT ( 'NONE', #45026 ) ;
#63503=CARTESIAN_POINT ( 'NONE',  ( 40.41628377845468378, 57.12529113016346827, 177.5919119679930134 ) ) ;
#63505=DIRECTION ( 'NONE',  ( 0.000000000000000000, 0.000000000000000000, 1.000000000000000000 ) ) ;
#63506=VERTEX_POINT ( 'NONE', #36930 ) ;
#63507=CARTESIAN_POINT ( 'NONE',  ( -19.15453390681661716, 24.31945705462845453, -10.00000000000000000 ) ) ;
#63509=VECTOR ( 'NONE', #11316, 1000.000000000000000 ) ;
#63511=ORIENTED_EDGE ( 'NONE', *, *, #23905, .F. ) ;
#63513=ORIENTED_EDGE ( 'NONE', *, *, #19029, .T. ) ;
#63515=ORIENTED_EDGE ( 'NONE', *, *, #1153, .F. ) ;
#63518=ADVANCED_FACE ( 'NONE', ( #75969 ), #58719, .F. ) ;
#63531=CYLINDRICAL_SURFACE ( 'NONE', #31176, 49.99999999999999289 ) ;
#63533=FACE_OUTER_BOUND ( 'NONE', #46278, .T. ) ;
#63536=DIRECTION ( 'NONE',  ( -0.9890802632347809320, 0.1473778574936430164, 0.000000000000000000 ) ) ;
#63540=EDGE_CURVE ( 'NONE', #2381, #20300, #95125, .T. ) ;
#63543=CARTESIAN_POINT ( 'NONE',  ( -50.41871976035449165, 31.58591985673634639, -10.00000000000000000 ) ) ;
#63563=ORIENTED_EDGE ( 'NONE', *, *, #75650, .F. ) ;
#63568=CARTESIAN_POINT ( 'NONE',  ( 25.34687108590969729, 93.06504152958497400, 20.00000000000000355 ) ) ;
#63572=VECTOR ( 'NONE', #65821, 1000.000000000000000 ) ;
#63585=AXIS2_PLACEMENT_3D ( 'NONE', #86707, #25345, #92422 ) ;
#63596=LINE ( 'NONE', #48404, #60432 ) ;
#63599=ORIENTED_EDGE ( 'NONE', *, *, #22163, .T. ) ;
#63604=ORIENTED_EDGE ( 'NONE', *, *, #80555, .F. ) ;
#63620=CYLINDRICAL_SURFACE ( 'NONE', #85869, 70.00000000000002842 ) ;
#63625=ORIENTED_EDGE ( 'NONE', *, *, #31534, .T. ) ;
#63633=ORIENTED_EDGE ( 'NONE', *, *, #68378, .T. ) ;
#63640=EDGE_CURVE ( 'NONE', #1592, #54743, #25228, .T. ) ;
#63646=VERTEX_POINT ( 'NONE', #49529 ) ;
#63648=VERTEX_POINT ( 'NONE', #88598 ) ;
#63661=VECTOR ( 'NONE', #47389, 999.9999999999998863 ) ;
#63664=AXIS2_PLACEMENT_3D ( 'NONE', #85343, #61491, #201 ) ;
#63666=CARTESIAN_POINT ( 'NONE',  ( 13.01414456110373052, 45.20707939394876007, 59.99999999999999289 ) ) ;
#63679=CARTESIAN_POINT ( 'NONE',  ( -19.42194755839791753, 24.31068691715150010, 10.00000000000000000 ) ) ;
#63682=CARTESIAN_POINT ( 'NONE',  ( 41.37327796571899796, 124.7191351846657028, -10.00000000000000000 ) ) ;
#63685=EDGE_CURVE ( 'NONE', #72572, #96097, #63736, .T. ) ;
#63693=CARTESIAN_POINT ( 'NONE',  ( 36.38358746446922254, 51.11404133282111673, 10.00000000000000000 ) ) ;
#63706=DIRECTION ( 'NONE',  ( 1.000000000000000000, 0.000000000000000000, 0.000000000000000000 ) ) ;
#63710=DIRECTION ( 'NONE',  ( -0.000000000000000000, -0.000000000000000000, -1.000000000000000000 ) ) ;
#63715=DIRECTION ( 'NONE',  ( -0.9825923819316307872, -0.1857746241280658905, 0.000000000000000000 ) ) ;
#63717=ORIENTED_EDGE ( 'NONE', *, *, #20664, .T. ) ;
#63723=DIRECTION ( 'NONE',  ( -0.06415622980648827411, 0.9979398670145497308, 0.000000000000000000 ) ) ;
#63725=VECTOR ( 'NONE', #81121, 999.9999999999998863 ) ;
#63736=LINE ( 'NONE', #96174, #1280 ) ;
#63740=CIRCLE ( 'NONE', #99330, 70.00000000000001421 ) ;
#63746=ORIENTED_EDGE ( 'NONE', *, *, #11228, .F. ) ;
#63750=CARTESIAN_POINT ( 'NONE',  ( 50.60128122559382291, 92.19983735941717384, 10.00000000000000000 ) ) ;
#63751=FACE_OUTER_BOUND ( 'NONE', #25963, .T. ) ;
#63752=CARTESIAN_POINT ( 'NONE',  ( -19.65312891409030271, 93.06504152958497400, 177.5919119679930134 ) ) ;
#63758=LINE ( 'NONE', #39430, #59417 ) ;
#63764=LINE ( 'NONE', #96203, #74278 ) ;
#63771=VERTEX_POINT ( 'NONE', #79481 ) ;
#63773=PLANE ( 'NONE',  #17116 ) ;
#63783=LINE ( 'NONE', #50571, #85650 ) ;
#63785=FACE_OUTER_BOUND ( 'NONE', #83905, .T. ) ;
#63791=DIRECTION ( 'NONE',  ( -0.000000000000000000, -0.000000000000000000, 1.000000000000000000 ) ) ;
#63793=EDGE_CURVE ( 'NONE', #59464, #57165, #10045, .T. ) ;
#63798=ADVANCED_FACE ( 'NONE', ( #25752 ), #18142, .F. ) ;
#63807=ORIENTED_EDGE ( 'NONE', *, *, #50652, .T. ) ;
#63808=VECTOR ( 'NONE', #59115, 1000.000000000000114 ) ;
#63809=DIRECTION ( 'NONE',  ( 0.000000000000000000, 0.000000000000000000, 1.000000000000000000 ) ) ;
#63821=EDGE_LOOP ( 'NONE', ( #64166, #19143, #84997, #27659 ) ) ;
#63823=CARTESIAN_POINT ( 'NONE',  ( -34.16292631813981728, 25.86630820016799248, -10.00000000000000000 ) ) ;
#63831=CARTESIAN_POINT ( 'NONE',  ( -6.662747857324052170, 100.5650415295849029, 1.836970198720989751E-15 ) ) ;
#63832=DIRECTION ( 'NONE',  ( -0.3103181967972223343, 0.9506327454577401248, 0.000000000000000000 ) ) ;
#63834=FACE_OUTER_BOUND ( 'NONE', #78101, .T. ) ;
#63839=DIRECTION ( 'NONE',  ( -0.000000000000000000, -0.000000000000000000, -1.000000000000000000 ) ) ;
#63842=LINE ( 'NONE', #77562, #15757 ) ;
#63844=CARTESIAN_POINT ( 'NONE',  ( -14.83894680564148238, 24.48641780169619508, -10.00000000000000000 ) ) ;
#63846=FACE_OUTER_BOUND ( 'NONE', #71133, .T. ) ;
#63855=ORIENTED_EDGE ( 'NONE', *, *, #49809, .F. ) ;
#63857=PLANE ( 'NONE',  #77162 ) ;
#63859=CARTESIAN_POINT ( 'NONE',  ( 20.67738335769525904, 35.85097175740956743, 10.00000000000000000 ) ) ;
#63860=ORIENTED_EDGE ( 'NONE', *, *, #79300, .T. ) ;
#63865=AXIS2_PLACEMENT_3D ( 'NONE', #29151, #6831, #38718 ) ;
#63871=EDGE_LOOP ( 'NONE', ( #87500, #6461, #71637, #87166 ) ) ;
#63875=LINE ( 'NONE', #24871, #35409 ) ;
#63876=ADVANCED_FACE ( 'NONE', ( #27242 ), #5925, .T. ) ;
#63878=AXIS2_PLACEMENT_3D ( 'NONE', #10769, #16355, #94393 ) ;
#63885=CARTESIAN_POINT ( 'NONE',  ( 43.53831125515428369, 65.97156238185917232, 10.00000000000000000 ) ) ;
#63891=PLANE ( 'NONE',  #56025 ) ;
#63892=EDGE_LOOP ( 'NONE', ( #27111, #30759, #29662, #76099 ) ) ;
#63909=ORIENTED_EDGE ( 'NONE', *, *, #59052, .F. ) ;
#63925=CARTESIAN_POINT ( 'NONE',  ( -40.08433460452723551, 25.84155934987275671, -10.00000000000000000 ) ) ;
#63926=EDGE_CURVE ( 'NONE', #70875, #17814, #46523, .T. ) ;
#63935=VECTOR ( 'NONE', #34388, 1000.000000000000000 ) ;
#63943=LINE ( 'NONE', #86306, #80698 ) ;
#63950=DIRECTION ( 'NONE',  ( -0.9599109957006575211, -0.2803049773603249473, 0.000000000000000000 ) ) ;
#63953=LINE ( 'NONE', #48260, #37529 ) ;
#63954=DIRECTION ( 'NONE',  ( 0.000000000000000000, 0.000000000000000000, 1.000000000000000000 ) ) ;
#63969=PLANE ( 'NONE',  #52584 ) ;
#63970=DIRECTION ( 'NONE',  ( 0.000000000000000000, 0.000000000000000000, 1.000000000000000000 ) ) ;
#63974=LINE ( 'NONE', #9286, #26337 ) ;
#63980=ORIENTED_EDGE ( 'NONE', *, *, #51690, .F. ) ;
#63983=AXIS2_PLACEMENT_3D ( 'NONE', #89050, #96616, #65658 ) ;
#63985=CARTESIAN_POINT ( 'NONE',  ( -33.92913075610074003, 36.15268528101246659, 59.99999999999999289 ) ) ;
#64003=VECTOR ( 'NONE', #39, 1000.000000000000000 ) ;
#64004=LINE ( 'NONE', #41187, #81271 ) ;
#64008=FACE_OUTER_BOUND ( 'NONE', #7161, .T. ) ;
#64010=ORIENTED_EDGE ( 'NONE', *, *, #48738, .T. ) ;
#64012=ORIENTED_EDGE ( 'NONE', *, *, #61176, .F. ) ;
#64015=ORIENTED_EDGE ( 'NONE', *, *, #7091, .T. ) ;
#64020=DIRECTION ( 'NONE',  ( -0.8263106059122556912, -0.5632146860273805622, 0.000000000000000000 ) ) ;
#64026=CARTESIAN_POINT ( 'NONE',  ( 45.11483101423404918, 69.99284853207299761, 10.00000000000000000 ) ) ;
#64032=ORIENTED_EDGE ( 'NONE', *, *, #39960, .F. ) ;
#64040=ORIENTED_EDGE ( 'NONE', *, *, #23855, .F. ) ;
#64041=DIRECTION ( 'NONE',  ( -0.8492021815265757834, 0.5280678506503729830, 0.000000000000000000 ) ) ;
#64042=EDGE_CURVE ( 'NONE', #14427, #50922, #58976, .T. ) ;
#64043=PLANE ( 'NONE',  #52823 ) ;
#64053=EDGE_CURVE ( 'NONE', #4321, #37845, #43293, .T. ) ;
#64061=VECTOR ( 'NONE', #97084, 1000.000000000000000 ) ;
#64079=CARTESIAN_POINT ( 'NONE',  ( 43.63646518856938172, 66.22046553916848666, 10.00000000000000000 ) ) ;
#64091=CARTESIAN_POINT ( 'NONE',  ( -32.30932376655839988, 25.48519649537502119, -10.00000000000000000 ) ) ;
#64093=ORIENTED_EDGE ( 'NONE', *, *, #99265, .T. ) ;
#64100=LINE ( 'NONE', #40775, #44098 ) ;
#64111=ORIENTED_EDGE ( 'NONE', *, *, #90976, .F. ) ;
#64121=AXIS2_PLACEMENT_3D ( 'NONE', #46460, #68771, #100202 ) ;
#64125=ORIENTED_EDGE ( 'NONE', *, *, #49809, .T. ) ;
#64129=VECTOR ( 'NONE', #8460, 1000.000000000000114 ) ;
#64142=CARTESIAN_POINT ( 'NONE',  ( 23.64814127513160358, 118.0650415295850166, -40.00000000000000711 ) ) ;
#64149=ORIENTED_EDGE ( 'NONE', *, *, #45398, .F. ) ;
#64154=LINE ( 'NONE', #25669, #22385 ) ;
#64158=VECTOR ( 'NONE', #70376, 1000.000000000000114 ) ;
#64166=ORIENTED_EDGE ( 'NONE', *, *, #40273, .F. ) ;
#64183=CARTESIAN_POINT ( 'NONE',  ( 41.49446470602975978, 58.46153712902343358, -10.00000000000000000 ) ) ;
#64190=VECTOR ( 'NONE', #51294, 999.9999999999998863 ) ;
#64204=EDGE_CURVE ( 'NONE', #9798, #26753, #59466, .T. ) ;
#64209=PLANE ( 'NONE',  #48980 ) ;
#64221=DIRECTION ( 'NONE',  ( -0.000000000000000000, 0.000000000000000000, -1.000000000000000000 ) ) ;
#64223=CARTESIAN_POINT ( 'NONE',  ( 31.47957939141361905, 85.21460096010893892, 59.99999999999999289 ) ) ;
#64228=ORIENTED_EDGE ( 'NONE', *, *, #93462, .F. ) ;
#64230=ORIENTED_EDGE ( 'NONE', *, *, #899, .F. ) ;
#64242=ORIENTED_EDGE ( 'NONE', *, *, #22731, .T. ) ;
#64253=DIRECTION ( 'NONE',  ( -0.5435407515102095299, 0.8393827800519358950, 0.000000000000000000 ) ) ;
#64256=DIRECTION ( 'NONE',  ( -0.8143688203140631021, 0.5803476755362091399, 0.000000000000000000 ) ) ;
#64265=CARTESIAN_POINT ( 'NONE',  ( 48.16808589598787904, 104.3116767361652535, -10.00000000000000000 ) ) ;
#64267=VECTOR ( 'NONE', #99450, 1000.000000000000000 ) ;
#64270=ORIENTED_EDGE ( 'NONE', *, *, #39398, .F. ) ;
#64271=ORIENTED_EDGE ( 'NONE', *, *, #68585, .F. ) ;
#64281=VERTEX_POINT ( 'NONE', #41312 ) ;
#64284=ADVANCED_FACE ( 'NONE', ( #89011 ), #57519, .T. ) ;
#64286=ORIENTED_EDGE ( 'NONE', *, *, #81189, .T. ) ;
#64292=ORIENTED_EDGE ( 'NONE', *, *, #92872, .T. ) ;
#64293=AXIS2_PLACEMENT_3D ( 'NONE', #44971, #37367, #59665 ) ;
#64313=CARTESIAN_POINT ( 'NONE',  ( 32.61785165683026122, 46.50599740114041225, 10.00000000000000000 ) ) ;
#64320=LINE ( 'NONE', #10126, #49726 ) ;
#64322=DIRECTION ( 'NONE',  ( -0.000000000000000000, 0.000000000000000000, -1.000000000000000000 ) ) ;
#64323=ORIENTED_EDGE ( 'NONE', *, *, #67351, .T. ) ;
#64338=VECTOR ( 'NONE', #93375, 1000.000000000000000 ) ;
#64345=CARTESIAN_POINT ( 'NONE',  ( -9.255205446392002600, 85.17849077645132638, 14.12110100382514410 ) ) ;
#64348=ORIENTED_EDGE ( 'NONE', *, *, #303, .T. ) ;
#64366=CARTESIAN_POINT ( 'NONE',  ( 7.819191540449072164, 28.68125778831126382, -10.00000000000000000 ) ) ;
#64377=EDGE_CURVE ( 'NONE', #85106, #72480, #42316, .T. ) ;
#64397=ORIENTED_EDGE ( 'NONE', *, *, #63348, .T. ) ;
#64400=CARTESIAN_POINT ( 'NONE',  ( 44.08135397534552169, 118.8355609772188188, -10.00000000000000000 ) ) ;
#64401=DIRECTION ( 'NONE',  ( -0.000000000000000000, -0.000000000000000000, -1.000000000000000000 ) ) ;
#64409=CIRCLE ( 'NONE', #61201, 0.1418229129681591871 ) ;
#64414=VECTOR ( 'NONE', #88270, 1000.000000000000000 ) ;
#64419=CARTESIAN_POINT ( 'NONE',  ( 46.89542285554266954, 70.53237680267110932, 10.00000000000000000 ) ) ;
#64425=VECTOR ( 'NONE', #49265, 1000.000000000000000 ) ;
#64432=CIRCLE ( 'NONE', #10856, 70.00000000000001421 ) ;
#64462=CARTESIAN_POINT ( 'NONE',  ( 46.30674614090290220, 112.4688969640381231, 10.00000000000000000 ) ) ;
#64467=CARTESIAN_POINT ( 'NONE',  ( -25.89332989531674301, 24.59406508915897760, -10.00000000000000000 ) ) ;
#64477=AXIS2_PLACEMENT_3D ( 'NONE', #38634, #53342, #84293 ) ;
#64495=EDGE_LOOP ( 'NONE', ( #73244, #3767, #65365, #84284 ) ) ;
#64496=AXIS2_PLACEMENT_3D ( 'NONE', #66095, #27611, #43276 ) ;
#64505=EDGE_CURVE ( 'NONE', #24764, #23591, #13445, .T. ) ;
#64508=VECTOR ( 'NONE', #2791, 1000.000000000000000 ) ;
#64515=ORIENTED_EDGE ( 'NONE', *, *, #47988, .F. ) ;
#64518=ORIENTED_EDGE ( 'NONE', *, *, #84564, .F. ) ;
#64519=ORIENTED_EDGE ( 'NONE', *, *, #76556, .T. ) ;
#64538=EDGE_LOOP ( 'NONE', ( #38299, #48823, #56245, #83809, #21738 ) ) ;
#64541=CARTESIAN_POINT ( 'NONE',  ( 43.35468487962022266, 120.5828561944265687, -10.00000000000000000 ) ) ;
#64542=CARTESIAN_POINT ( 'NONE',  ( 40.82928596147627331, 60.38352576601455723, -10.00000000000000000 ) ) ;
#64549=AXIS2_PLACEMENT_3D ( 'NONE', #22045, #91998, #22548 ) ;
#64550=CARTESIAN_POINT ( 'NONE',  ( -28.64605662510459183, 40.80936565889331291, 59.99999999999999289 ) ) ;
#64554=AXIS2_PLACEMENT_3D ( 'NONE', #6874, #83421, #69667 ) ;
#64557=VECTOR ( 'NONE', #66297, 1000.000000000000000 ) ;
#64562=AXIS2_PLACEMENT_3D ( 'NONE', #80674, #19834, #3640 ) ;
#64564=ORIENTED_EDGE ( 'NONE', *, *, #59213, .F. ) ;
#64570=CARTESIAN_POINT ( 'NONE',  ( -77.58047734835668052, 56.02942318228900120, 10.00000000000000000 ) ) ;
#64571=VECTOR ( 'NONE', #25998, 1000.000000000000114 ) ;
#64576=EDGE_LOOP ( 'NONE', ( #55022, #43068, #72995, #49130 ) ) ;
#64587=CARTESIAN_POINT ( 'NONE',  ( 43.24043327773039636, 120.8247932685368227, -10.00000000000000000 ) ) ;
#64591=EDGE_CURVE ( 'NONE', #49306, #49232, #67116, .T. ) ;
#64597=CARTESIAN_POINT ( 'NONE',  ( 39.64431452495995245, 58.26521502737223557, 10.00000000000000000 ) ) ;
#64606=CARTESIAN_POINT ( 'NONE',  ( -5.171971415982786979, 24.31384663199769491, 10.00000000000000000 ) ) ;
#64611=EDGE_CURVE ( 'NONE', #10907, #1989, #35336, .T. ) ;
#64630=EDGE_CURVE ( 'NONE', #5467, #27174, #67663, .T. ) ;
#64645=LINE ( 'NONE', #55507, #45981 ) ;
#64646=CIRCLE ( 'NONE', #14453, 70.00000000000001421 ) ;
#64659=ORIENTED_EDGE ( 'NONE', *, *, #25303, .F. ) ;
#64662=VERTEX_POINT ( 'NONE', #18934 ) ;
#64665=CARTESIAN_POINT ( 'NONE',  ( 44.98086946945897324, 119.9434018396067643, 177.5919119679930134 ) ) ;
#64673=ORIENTED_EDGE ( 'NONE', *, *, #21384, .F. ) ;
#64677=LINE ( 'NONE', #41859, #40288 ) ;
#64707=DIRECTION ( 'NONE',  ( 1.000000000000000000, 0.000000000000000000, 0.000000000000000000 ) ) ;
#64711=LINE ( 'NONE', #72834, #31914 ) ;
#64712=DIRECTION ( 'NONE',  ( 0.000000000000000000, 0.000000000000000000, 1.000000000000000000 ) ) ;
#64720=LINE ( 'NONE', #95669, #87330 ) ;
#64725=LINE ( 'NONE', #26221, #87200 ) ;
#64730=CARTESIAN_POINT ( 'NONE',  ( 38.52196584993465223, 56.41980893122115504, -10.00000000000000000 ) ) ;
#64733=DIRECTION ( 'NONE',  ( -0.000000000000000000, 0.000000000000000000, 1.000000000000000000 ) ) ;
#64735=FACE_OUTER_BOUND ( 'NONE', #48155, .T. ) ;
#64740=ADVANCED_FACE ( 'NONE', ( #28000 ), #74633, .F. ) ;
#64742=ORIENTED_EDGE ( 'NONE', *, *, #65508, .F. ) ;
#64744=ORIENTED_EDGE ( 'NONE', *, *, #100085, .T. ) ;
#64749=DIRECTION ( 'NONE',  ( -0.9481851146622203297, -0.3177184104407421716, 0.000000000000000000 ) ) ;
#64751=ORIENTED_EDGE ( 'NONE', *, *, #53947, .T. ) ;
#64761=CARTESIAN_POINT ( 'NONE',  ( -0.8836234265189104597, 25.35879081310345029, -10.00000000000000000 ) ) ;
#64772=VECTOR ( 'NONE', #84895, 1000.000000000000000 ) ;
#64776=ORIENTED_EDGE ( 'NONE', *, *, #8245, .F. ) ;
#64778=DIRECTION ( 'NONE',  ( 0.000000000000000000, 0.000000000000000000, 1.000000000000000000 ) ) ;
#64787=LINE ( 'NONE', #96215, #26918 ) ;
#64791=CARTESIAN_POINT ( 'NONE',  ( 45.11483101423404918, 69.99284853207299761, 10.00000000000000000 ) ) ;
#64794=ADVANCED_FACE ( 'NONE', ( #82754 ), #12831, .F. ) ;
#64798=DIRECTION ( 'NONE',  ( 0.000000000000000000, -0.000000000000000000, 1.000000000000000000 ) ) ;
#64804=CARTESIAN_POINT ( 'NONE',  ( -12.95261720355844126, 24.63757726406876714, -10.00000000000000000 ) ) ;
#64807=DIRECTION ( 'NONE',  ( 1.000000000000000000, -4.068174368805037318E-13, 0.000000000000000000 ) ) ;
#64821=EDGE_CURVE ( 'NONE', #43030, #12312, #5697, .T. ) ;
#64824=CARTESIAN_POINT ( 'NONE',  ( -42.47074677134370546, 28.21475011077167849, -10.00000000000000000 ) ) ;
#64828=EDGE_CURVE ( 'NONE', #49424, #51013, #29496, .T. ) ;
#64847=LINE ( 'NONE', #16736, #28412 ) ;
#64851=CARTESIAN_POINT ( 'NONE',  ( -54.35768244943842120, 45.75294371086302903, 59.99999999999999289 ) ) ;
#64855=CARTESIAN_POINT ( 'NONE',  ( -17.48682250002296712, 81.73217073256289211, 14.51763226715314126 ) ) ;
#64856=LINE ( 'NONE', #33450, #12580 ) ;
#64867=VERTEX_POINT ( 'NONE', #22393 ) ;
#64870=CARTESIAN_POINT ( 'NONE',  ( -56.29836151245349640, 34.88994676555962116, 10.00000000000000000 ) ) ;
#64876=FACE_OUTER_BOUND ( 'NONE', #84585, .T. ) ;
#64890=EDGE_CURVE ( 'NONE', #63648, #22887, #25581, .T. ) ;
#64892=VERTEX_POINT ( 'NONE', #68982 ) ;
#64902=CARTESIAN_POINT ( 'NONE',  ( 44.44706364856357084, 64.93738052781135650, -10.00000000000000000 ) ) ;
#64904=DIRECTION ( 'NONE',  ( 0.9994538543569184696, -0.03304531753667278721, 0.000000000000000000 ) ) ;
#64914=DIRECTION ( 'NONE',  ( 0.9979227057047517224, -0.06442261589618512863, 0.000000000000000000 ) ) ;
#64923=CARTESIAN_POINT ( 'NONE',  ( -19.53260179278070652, 92.99029561550555911, 59.99999999999999289 ) ) ;
#64927=VECTOR ( 'NONE', #54867, 1000.000000000000114 ) ;
#64938=CARTESIAN_POINT ( 'NONE',  ( -29.41917662106829212, 23.74964416229700248, 10.00000000000000000 ) ) ;
#64941=EDGE_CURVE ( 'NONE', #4560, #22737, #591, .T. ) ;
#64960=DIRECTION ( 'NONE',  ( -0.6623377501714527993, 0.7492053821868994712, 0.000000000000000000 ) ) ;
#64998=VECTOR ( 'NONE', #46643, 1000.000000000000114 ) ;
#65007=LINE ( 'NONE', #73607, #21585 ) ;
#65015=ORIENTED_EDGE ( 'NONE', *, *, #2043, .F. ) ;
#65020=ORIENTED_EDGE ( 'NONE', *, *, #76556, .F. ) ;
#65022=ORIENTED_EDGE ( 'NONE', *, *, #26832, .T. ) ;
#65028=CARTESIAN_POINT ( 'NONE',  ( 25.88271472100439041, 39.90032630942972247, -10.00000000000000000 ) ) ;
#65030=VERTEX_POINT ( 'NONE', #94825 ) ;
#65033=DIRECTION ( 'NONE',  ( -0.6116140086401625764, 0.7911563084720434347, 0.000000000000000000 ) ) ;
#65040=DIRECTION ( 'NONE',  ( -0.000000000000000000, 0.000000000000000000, -1.000000000000000000 ) ) ;
#65043=ORIENTED_EDGE ( 'NONE', *, *, #19363, .T. ) ;
#65045=LINE ( 'NONE', #55911, #33843 ) ;
#65061=DIRECTION ( 'NONE',  ( 0.1783728972749306640, 0.9839629614562466209, 0.000000000000000000 ) ) ;
#65068=ADVANCED_FACE ( 'NONE', ( #18306 ), #80138, .F. ) ;
#65080=EDGE_LOOP ( 'NONE', ( #20825, #68571, #97658, #60265 ) ) ;
#65093=LINE ( 'NONE', #2315, #28073 ) ;
#65096=ORIENTED_EDGE ( 'NONE', *, *, #19842, .T. ) ;
#65107=LINE ( 'NONE', #34212, #90593 ) ;
#65109=ORIENTED_EDGE ( 'NONE', *, *, #93047, .F. ) ;
#65119=LINE ( 'NONE', #32213, #24898 ) ;
#65127=CARTESIAN_POINT ( 'NONE',  ( -28.63239376340754561, 61.06670042544809007, -10.00000000000000000 ) ) ;
#65131=EDGE_CURVE ( 'NONE', #69843, #4429, #7785, .T. ) ;
#65134=ORIENTED_EDGE ( 'NONE', *, *, #79460, .T. ) ;
#65136=CARTESIAN_POINT ( 'NONE',  ( 32.14254330279432992, 120.6340272870843364, 59.99999999999999289 ) ) ;
#65149=ORIENTED_EDGE ( 'NONE', *, *, #92424, .F. ) ;
#65156=DIRECTION ( 'NONE',  ( -1.000000000000000000, 0.000000000000000000, 0.000000000000000000 ) ) ;
#65158=ORIENTED_EDGE ( 'NONE', *, *, #48377, .T. ) ;
#65164=CARTESIAN_POINT ( 'NONE',  ( 50.15574305400770072, 101.0118721476823964, 10.00000000000000000 ) ) ;
#65167=VECTOR ( 'NONE', #1300, 999.9999999999998863 ) ;
#65168=CARTESIAN_POINT ( 'NONE',  ( -19.65312891409030271, 93.06504152958497400, 10.00000000000000888 ) ) ;
#65172=ORIENTED_EDGE ( 'NONE', *, *, #45944, .F. ) ;
#65173=ADVANCED_FACE ( 'NONE', ( #36472 ), #75496, .F. ) ;
#65175=DIRECTION ( 'NONE',  ( 0.7696402260561062691, 0.6384778167143364547, 0.000000000000000000 ) ) ;
#65188=CARTESIAN_POINT ( 'NONE',  ( -19.63199130574582796, 93.20528039779287610, 59.99999999999999289 ) ) ;
#65189=ADVANCED_FACE ( 'NONE', ( #46054 ), #53179, .F. ) ;
#65190=VECTOR ( 'NONE', #54615, 1000.000000000000227 ) ;
#65194=EDGE_CURVE ( 'NONE', #30353, #41966, #41762, .T. ) ;
#65196=EDGE_CURVE ( 'NONE', #98414, #28497, #77493, .T. ) ;
#65197=CARTESIAN_POINT ( 'NONE',  ( -19.65312891409030271, 93.06504152958497400, 10.00000000000000888 ) ) ;
#65223=LINE ( 'NONE', #27233, #79308 ) ;
#65240=EDGE_CURVE ( 'NONE', #35732, #90334, #30877, .T. ) ;
#65253=AXIS2_PLACEMENT_3D ( 'NONE', #69689, #23081, #24586 ) ;
#65254=CARTESIAN_POINT ( 'NONE',  ( -19.57831724403558837, 92.94455521224399774, 59.99999999999999289 ) ) ;
#65257=EDGE_CURVE ( 'NONE', #28901, #85997, #62760, .T. ) ;
#65258=CARTESIAN_POINT ( 'NONE',  ( 47.05668214639808156, 76.45164061169337799, -10.00000000000000000 ) ) ;
#65261=ORIENTED_EDGE ( 'NONE', *, *, #33829, .F. ) ;
#65263=DIRECTION ( 'NONE',  ( -0.9862134920484688649, -0.1654779384134468789, 0.000000000000000000 ) ) ;
#65271=DIRECTION ( 'NONE',  ( 0.4552093898365224267, -0.8903844177683372108, 0.000000000000000000 ) ) ;
#65272=LINE ( 'NONE', #19204, #94918 ) ;
#65273=EDGE_CURVE ( 'NONE', #69721, #63278, #80660, .T. ) ;
#65275=ORIENTED_EDGE ( 'NONE', *, *, #5997, .F. ) ;
#65282=PLANE ( 'NONE',  #23538 ) ;
#65287=FACE_OUTER_BOUND ( 'NONE', #74217, .T. ) ;
#65296=DIRECTION ( 'NONE',  ( -0.000000000000000000, -0.000000000000000000, -1.000000000000000000 ) ) ;
#65297=DIRECTION ( 'NONE',  ( -0.8099771808667527440, -0.5864613938488599798, 0.000000000000000000 ) ) ;
#65298=DIRECTION ( 'NONE',  ( -0.000000000000000000, 0.000000000000000000, -1.000000000000000000 ) ) ;
#65310=ADVANCED_FACE ( 'NONE', ( #50071 ), #80519, .F. ) ;
#65319=AXIS2_PLACEMENT_3D ( 'NONE', #9516, #26699, #73799 ) ;
#65322=VECTOR ( 'NONE', #6919, 1000.000000000000227 ) ;
#65332=DIRECTION ( 'NONE',  ( 0.9954067278227226589, -0.09573633691164461224, 0.000000000000000000 ) ) ;
#65334=PRODUCT ( 'Middle Movable Base', 'Middle Movable Base', '', ( #60334 ) ) ;
#65336=CARTESIAN_POINT ( 'NONE',  ( 46.22371820283660782, 112.7232458147606451, 10.00000000000000000 ) ) ;
#65342=ORIENTED_EDGE ( 'NONE', *, *, #97782, .T. ) ;
#65353=CARTESIAN_POINT ( 'NONE',  ( -64.94778771796556782, 41.33875607593969193, -10.00000000000000000 ) ) ;
#65354=ORIENTED_EDGE ( 'NONE', *, *, #69079, .F. ) ;
#65357=DIRECTION ( 'NONE',  ( -1.000000000000000000, 4.892646582057456999E-14, 0.000000000000000000 ) ) ;
#65358=DIRECTION ( 'NONE',  ( -0.09274582908234026146, -0.9956898167541081701, 0.000000000000000000 ) ) ;
#65363=DIRECTION ( 'NONE',  ( -0.9981117208278907915, 0.06142469166374903145, 0.000000000000000000 ) ) ;
#65365=ORIENTED_EDGE ( 'NONE', *, *, #54147, .F. ) ;
#65370=DIRECTION ( 'NONE',  ( -0.000000000000000000, -0.000000000000000000, -1.000000000000000000 ) ) ;
#65376=ADVANCED_FACE ( 'NONE', ( #11094 ), #72401, .T. ) ;
#65377=CARTESIAN_POINT ( 'NONE',  ( -73.83803415018344651, 50.74234351129840093, -10.00000000000000000 ) ) ;
#65378=EDGE_LOOP ( 'NONE', ( #93723, #72515, #96016, #53988 ) ) ;
#65393=CARTESIAN_POINT ( 'NONE',  ( 33.63407072503001416, 49.62913085183823370, -10.00000000000000000 ) ) ;
#65401=VECTOR ( 'NONE', #42318, 1000.000000000000114 ) ;
#65411=CARTESIAN_POINT ( 'NONE',  ( -53.68831936616819434, 31.89637462494507147, 10.00000000000000000 ) ) ;
#65413=DIRECTION ( 'NONE',  ( -1.000000000000000000, 0.000000000000000000, 0.000000000000000000 ) ) ;
#65416=DIRECTION ( 'NONE',  ( 0.000000000000000000, 0.000000000000000000, 1.000000000000000000 ) ) ;
#65417=ORIENTED_EDGE ( 'NONE', *, *, #53760, .F. ) ;
#65418=CARTESIAN_POINT ( 'NONE',  ( 48.53010236944520273, 101.9116055364396090, -10.00000000000000000 ) ) ;
#65426=DIRECTION ( 'NONE',  ( 0.04218457335174655848, 0.9991098346884246251, 0.000000000000000000 ) ) ;
#65433=CARTESIAN_POINT ( 'NONE',  ( 7.225231395932167899, 28.43104314603600358, 10.00000000000000000 ) ) ;
#65437=VERTEX_POINT ( 'NONE', #23633 ) ;
#65454=VECTOR ( 'NONE', #83881, 1000.000000000000000 ) ;
#65464=CARTESIAN_POINT ( 'NONE',  ( 4.102725850843912170, 28.55253618238880620, 10.00000000000000000 ) ) ;
#65479=EDGE_LOOP ( 'NONE', ( #73638, #11964, #60850, #66129 ) ) ;
#65484=ORIENTED_EDGE ( 'NONE', *, *, #56105, .F. ) ;
#65485=ORIENTED_EDGE ( 'NONE', *, *, #13400, .F. ) ;
#65489=ORIENTED_EDGE ( 'NONE', *, *, #60060, .F. ) ;
#65492=VERTEX_POINT ( 'NONE', #84012 ) ;
#65497=VERTEX_POINT ( 'NONE', #357 ) ;
#65501=ORIENTED_EDGE ( 'NONE', *, *, #53579, .T. ) ;
#65503=DIRECTION ( 'NONE',  ( -1.000000000000000000, 0.000000000000000000, 0.000000000000000000 ) ) ;
#65507=ORIENTED_EDGE ( 'NONE', *, *, #82257, .F. ) ;
#65508=EDGE_CURVE ( 'NONE', #79283, #93301, #64154, .T. ) ;
#65525=VERTEX_POINT ( 'NONE', #56550 ) ;
#65527=CYLINDRICAL_SURFACE ( 'NONE', #56170, 60.00000000000002132 ) ;
#65529=DIRECTION ( 'NONE',  ( 0.000000000000000000, 0.000000000000000000, 1.000000000000000000 ) ) ;
#65543=CARTESIAN_POINT ( 'NONE',  ( 50.33662733789741139, 94.26254718190894266, 10.00000000000000000 ) ) ;
#65564=EDGE_CURVE ( 'NONE', #73010, #3544, #20439, .T. ) ;
#65571=DIRECTION ( 'NONE',  ( -0.9182972510888884887, 0.3958915996110436430, 0.000000000000000000 ) ) ;
#65582=DIRECTION ( 'NONE',  ( 0.000000000000000000, 0.000000000000000000, 1.000000000000000000 ) ) ;
#65597=VECTOR ( 'NONE', #56098, 1000.000000000000000 ) ;
#65607=DIRECTION ( 'NONE',  ( -0.5888918169447132644, 0.8082118706970061739, 0.000000000000000000 ) ) ;
#65608=AXIS2_PLACEMENT_3D ( 'NONE', #33712, #28086, #50387 ) ;
#65609=ORIENTED_EDGE ( 'NONE', *, *, #68513, .F. ) ;
#65613=VERTEX_POINT ( 'NONE', #33781 ) ;
#65618=ORIENTED_EDGE ( 'NONE', *, *, #62571, .T. ) ;
#65621=ORIENTED_EDGE ( 'NONE', *, *, #58813, .T. ) ;
#65625=LINE ( 'NONE', #89013, #55680 ) ;
#65627=VERTEX_POINT ( 'NONE', #10974 ) ;
#65633=ADVANCED_FACE ( 'NONE', ( #37108 ), #21423, .F. ) ;
#65635=LINE ( 'NONE', #73747, #7857 ) ;
#65637=EDGE_LOOP ( 'NONE', ( #53173, #9160 ) ) ;
#65641=VECTOR ( 'NONE', #39607, 1000.000000000000114 ) ;
#65644=CARTESIAN_POINT ( 'NONE',  ( -46.35039662390601478, 28.35603213498495023, -10.00000000000000000 ) ) ;
#65648=VECTOR ( 'NONE', #73282, 1000.000000000000000 ) ;
#65655=CARTESIAN_POINT ( 'NONE',  ( -8.406493707509316238, 25.24382671950690948, -10.00000000000000000 ) ) ;
#65658=DIRECTION ( 'NONE',  ( 1.000000000000000000, 0.000000000000000000, 0.000000000000000000 ) ) ;
#65660=DIRECTION ( 'NONE',  ( -0.000000000000000000, -0.000000000000000000, -1.000000000000000000 ) ) ;
#65664=CIRCLE ( 'NONE', #4195, 70.00000000000001421 ) ;
#65665=AXIS2_PLACEMENT_3D ( 'NONE', #51093, #29804, #83547 ) ;
#65683=DIRECTION ( 'NONE',  ( -0.2500151307524235422, 0.9682419296822714072, 0.000000000000000000 ) ) ;
#65685=CARTESIAN_POINT ( 'NONE',  ( -19.74615283476394367, 92.95798879106189361, 59.99999999999999289 ) ) ;
#65687=EDGE_CURVE ( 'NONE', #88229, #39565, #97938, .T. ) ;
#65689=LINE ( 'NONE', #35294, #98332 ) ;
#65694=CARTESIAN_POINT ( 'NONE',  ( -19.65312891409030271, 93.06504152958497400, 10.00000000000000888 ) ) ;
#65706=CARTESIAN_POINT ( 'NONE',  ( 48.43557798863805886, 76.81918075477977936, 177.5919119679930134 ) ) ;
#65707=VECTOR ( 'NONE', #85244, 1000.000000000000000 ) ;
#65710=CARTESIAN_POINT ( 'NONE',  ( 50.33662733789742560, 94.26254718190892845, 177.5919119679930134 ) ) ;
#65714=VERTEX_POINT ( 'NONE', #62904 ) ;
#65716=ORIENTED_EDGE ( 'NONE', *, *, #84540, .F. ) ;
#65719=ORIENTED_EDGE ( 'NONE', *, *, #57949, .F. ) ;
#65720=CARTESIAN_POINT ( 'NONE',  ( 49.60098510475376088, 81.22027839155747131, 10.00000000000000000 ) ) ;
#65733=FACE_OUTER_BOUND ( 'NONE', #1261, .T. ) ;
#65734=AXIS2_PLACEMENT_3D ( 'NONE', #50565, #12084, #35368 ) ;
#65735=VERTEX_POINT ( 'NONE', #118 ) ;
#65736=ORIENTED_EDGE ( 'NONE', *, *, #44686, .F. ) ;
#65743=LINE ( 'NONE', #95210, #45166 ) ;
#65746=EDGE_CURVE ( 'NONE', #14010, #32823, #49222, .T. ) ;
#65764=CARTESIAN_POINT ( 'NONE',  ( -0.2492734796364602656, 27.10516647459198225, -10.00000000000000000 ) ) ;
#65768=AXIS2_PLACEMENT_3D ( 'NONE', #16695, #63791, #86655 ) ;
#65774=ORIENTED_EDGE ( 'NONE', *, *, #15929, .F. ) ;
#65775=VECTOR ( 'NONE', #16445, 1000.000000000000114 ) ;
#65779=LINE ( 'NONE', #50580, #15727 ) ;
#65781=AXIS2_PLACEMENT_3D ( 'NONE', #28759, #74393, #30251 ) ;
#65795=ADVANCED_FACE ( 'NONE', ( #33338 ), #40912, .T. ) ;
#65797=DIRECTION ( 'NONE',  ( -0.7061384650677096086, -0.7080737730998225565, 0.000000000000000000 ) ) ;
#65803=EDGE_LOOP ( 'NONE', ( #75887, #75098, #18078, #87268 ) ) ;
#65804=EDGE_CURVE ( 'NONE', #83079, #25248, #100003, .T. ) ;
#65814=CARTESIAN_POINT ( 'NONE',  ( 44.95821123098110661, 116.5722627105190270, -10.00000000000000000 ) ) ;
#65817=DIRECTION ( 'NONE',  ( -0.2805612043866616556, -0.9598361373656993933, 0.000000000000000000 ) ) ;
#65818=ADVANCED_FACE ( 'NONE', ( #78971 ), #62216, .F. ) ;
#65821=DIRECTION ( 'NONE',  ( 0.000000000000000000, 0.000000000000000000, 1.000000000000000000 ) ) ;
#65823=ORIENTED_EDGE ( 'NONE', *, *, #77420, .T. ) ;
#65825=VERTEX_POINT ( 'NONE', #48027 ) ;
#65829=ORIENTED_EDGE ( 'NONE', *, *, #27330, .T. ) ;
#65832=CARTESIAN_POINT ( 'NONE',  ( -19.65312891409030271, 93.06504152958497400, 10.00000000000000888 ) ) ;
#65843=LINE ( 'NONE', #21749, #21341 ) ;
#65850=VERTEX_POINT ( 'NONE', #11057 ) ;
#65855=DIRECTION ( 'NONE',  ( -0.000000000000000000, 0.000000000000000000, 1.000000000000000000 ) ) ;
#65864=ADVANCED_FACE ( 'NONE', ( #3459 ), #56634, .T. ) ;
#65868=ORIENTED_EDGE ( 'NONE', *, *, #97604, .T. ) ;
#65869=AXIS2_PLACEMENT_3D ( 'NONE', #34035, #10726, #41094 ) ;
#65876=EDGE_CURVE ( 'NONE', #83731, #1098, #35327, .T. ) ;
#65881=LINE ( 'NONE', #90234, #69324 ) ;
#65887=ORIENTED_EDGE ( 'NONE', *, *, #85646, .F. ) ;
#65889=DIRECTION ( 'NONE',  ( 0.7884491381006394350, -0.6150999566154746745, 0.000000000000000000 ) ) ;
#65891=DIRECTION ( 'NONE',  ( -0.000000000000000000, -0.000000000000000000, -1.000000000000000000 ) ) ;
#65892=CARTESIAN_POINT ( 'NONE',  ( 11.23059542939759581, 30.24628978557580083, 177.5919119679930134 ) ) ;
#65897=ORIENTED_EDGE ( 'NONE', *, *, #53495, .T. ) ;
#65906=DIRECTION ( 'NONE',  ( -1.000000000000000000, 0.000000000000000000, 0.000000000000000000 ) ) ;
#65916=CIRCLE ( 'NONE', #57815, 49.99999999999999289 ) ;
#65917=VECTOR ( 'NONE', #18158, 1000.000000000000114 ) ;
#65927=VECTOR ( 'NONE', #8498, 1000.000000000000114 ) ;
#65941=AXIS2_PLACEMENT_3D ( 'NONE', #4084, #97315, #5091 ) ;
#65944=FACE_OUTER_BOUND ( 'NONE', #46027, .T. ) ;
#65948=EDGE_CURVE ( 'NONE', #38684, #80425, #45092, .T. ) ;
#65951=EDGE_CURVE ( 'NONE', #74392, #95597, #3936, .T. ) ;
#65956=DIRECTION ( 'NONE',  ( -0.9778746070300391446, 0.2091919045418505763, 0.000000000000000000 ) ) ;
#65985=EDGE_CURVE ( 'NONE', #9430, #53961, #10548, .T. ) ;
#66004=ORIENTED_EDGE ( 'NONE', *, *, #37950, .F. ) ;
#66008=EDGE_CURVE ( 'NONE', #93223, #75236, #33773, .T. ) ;
#66012=DIRECTION ( 'NONE',  ( -1.000000000000000000, 0.000000000000000000, 0.000000000000000000 ) ) ;
#66014=VECTOR ( 'NONE', #15370, 1000.000000000000114 ) ;
#66020=CARTESIAN_POINT ( 'NONE',  ( -19.65312891409030271, 93.06504152958497400, 177.5919119679930134 ) ) ;
#66022=AXIS2_PLACEMENT_3D ( 'NONE', #16278, #31968, #16776 ) ;
#66025=CARTESIAN_POINT ( 'NONE',  ( -56.29836151245349640, 34.88994676555962116, 10.00000000000000000 ) ) ;
#66028=CARTESIAN_POINT ( 'NONE',  ( 46.54103524584390783, 115.8319611975524595, -10.00000000000000000 ) ) ;
#66035=DIRECTION ( 'NONE',  ( 0.000000000000000000, 0.000000000000000000, 1.000000000000000000 ) ) ;
#66038=VERTEX_POINT ( 'NONE', #55986 ) ;
#66041=AXIS2_PLACEMENT_3D ( 'NONE', #12372, #95007, #88426 ) ;
#66043=FACE_OUTER_BOUND ( 'NONE', #51669, .T. ) ;
#66044=EDGE_CURVE ( 'NONE', #74402, #50322, #92556, .T. ) ;
#66049=DIRECTION ( 'NONE',  ( 0.000000000000000000, 0.000000000000000000, 1.000000000000000000 ) ) ;
#66055=FACE_OUTER_BOUND ( 'NONE', #3967, .T. ) ;
#66069=VECTOR ( 'NONE', #12705, 1000.000000000000114 ) ;
#66071=VECTOR ( 'NONE', #69374, 1000.000000000000000 ) ;
#66076=CARTESIAN_POINT ( 'NONE',  ( -3.153128914090298274, 64.48620320469859735, 0.000000000000000000 ) ) ;
#66082=EDGE_CURVE ( 'NONE', #91721, #71865, #78836, .T. ) ;
#66084=DIRECTION ( 'NONE',  ( 0.7005979833698788850, 0.7135562106085679979, 0.000000000000000000 ) ) ;
#66088=LINE ( 'NONE', #87958, #54871 ) ;
#66095=CARTESIAN_POINT ( 'NONE',  ( 41.82599275875796252, 62.29945068332010294, -10.00000000000000000 ) ) ;
#66099=DIRECTION ( 'NONE',  ( 0.000000000000000000, -0.000000000000000000, 1.000000000000000000 ) ) ;
#66104=LINE ( 'NONE', #97528, #82557 ) ;
#66109=EDGE_LOOP ( 'NONE', ( #13181, #66381, #19041, #2517 ) ) ;
#66113=ORIENTED_EDGE ( 'NONE', *, *, #19029, .F. ) ;
#66115=DIRECTION ( 'NONE',  ( -1.000000000000000000, 0.000000000000000000, 0.000000000000000000 ) ) ;
#66116=VECTOR ( 'NONE', #35783, 1000.000000000000227 ) ;
#66118=VERTEX_POINT ( 'NONE', #46913 ) ;
#66124=EDGE_CURVE ( 'NONE', #19199, #88235, #84953, .T. ) ;
#66129=ORIENTED_EDGE ( 'NONE', *, *, #29455, .F. ) ;
#66136=VECTOR ( 'NONE', #80288, 1000.000000000000000 ) ;
#66147=EDGE_CURVE ( 'NONE', #96097, #90241, #94057, .T. ) ;
#66160=VECTOR ( 'NONE', #79745, 1000.000000000000227 ) ;
#66165=VERTEX_POINT ( 'NONE', #30723 ) ;
#66168=DIRECTION ( 'NONE',  ( -0.8218955677251095215, -0.5696381972391070247, 0.000000000000000000 ) ) ;
#66170=PLANE ( 'NONE',  #77511 ) ;
#66173=VECTOR ( 'NONE', #74599, 1000.000000000000000 ) ;
#66174=DIRECTION ( 'NONE',  ( -0.000000000000000000, -0.000000000000000000, -1.000000000000000000 ) ) ;
#66175=ORIENTED_EDGE ( 'NONE', *, *, #7828, .T. ) ;
#66185=CARTESIAN_POINT ( 'NONE',  ( -15.10528209597770299, 24.46087392797018722, 10.00000000000000000 ) ) ;
#66191=CARTESIAN_POINT ( 'NONE',  ( 21.20245638554208867, 36.22472881207376361, 177.5919119679930134 ) ) ;
#66201=EDGE_CURVE ( 'NONE', #34850, #59964, #39781, .T. ) ;
#66202=DIRECTION ( 'NONE',  ( 0.9053220668578600971, 0.4247257412262792631, 0.000000000000000000 ) ) ;
#66204=VECTOR ( 'NONE', #34949, 1000.000000000000000 ) ;
#66216=DIRECTION ( 'NONE',  ( -0.9172102815912978047, -0.3984034379159046568, 0.000000000000000000 ) ) ;
#66228=AXIS2_PLACEMENT_3D ( 'NONE', #86113, #30846, #92681 ) ;
#66235=CARTESIAN_POINT ( 'NONE',  ( 38.65784837781280459, 56.65029301956751340, 10.00000000000000000 ) ) ;
#66237=ORIENTED_EDGE ( 'NONE', *, *, #51252, .F. ) ;
#66245=CIRCLE ( 'NONE', #22557, 70.00000000000001421 ) ;
#66251=ORIENTED_EDGE ( 'NONE', *, *, #30407, .T. ) ;
#66262=DIRECTION ( 'NONE',  ( 0.000000000000000000, 0.000000000000000000, 1.000000000000000000 ) ) ;
#66263=EDGE_CURVE ( 'NONE', #95838, #68986, #100076, .T. ) ;
#66264=CARTESIAN_POINT ( 'NONE',  ( 43.83595887736690599, 122.5461495720015677, 177.5919119679930134 ) ) ;
#66267=CYLINDRICAL_SURFACE ( 'NONE', #90059, 70.00000000000002842 ) ;
#66270=ORIENTED_EDGE ( 'NONE', *, *, #16537, .T. ) ;
#66277=ORIENTED_EDGE ( 'NONE', *, *, #54298, .T. ) ;
#66280=FACE_OUTER_BOUND ( 'NONE', #81789, .T. ) ;
#66283=VECTOR ( 'NONE', #26765, 1000.000000000000000 ) ;
#66290=VECTOR ( 'NONE', #37769, 1000.000000000000000 ) ;
#66297=DIRECTION ( 'NONE',  ( -0.000000000000000000, -0.000000000000000000, -1.000000000000000000 ) ) ;
#66298=DIRECTION ( 'NONE',  ( -1.000000000000000000, 0.000000000000000000, 0.000000000000000000 ) ) ;
#66299=CARTESIAN_POINT ( 'NONE',  ( 29.13110022456613635, 42.86445400964587549, 10.00000000000000000 ) ) ;
#66306=VECTOR ( 'NONE', #60095, 1000.000000000000114 ) ;
#66308=DIRECTION ( 'NONE',  ( -0.1860369090531061032, -0.9825427565607341984, 0.000000000000000000 ) ) ;
#66311=VECTOR ( 'NONE', #89185, 1000.000000000000114 ) ;
#66313=LINE ( 'NONE', #21705, #4530 ) ;
#66322=CARTESIAN_POINT ( 'NONE',  ( 32.07315653955450330, 47.77038272570916888, -10.00000000000000000 ) ) ;
#66340=ORIENTED_EDGE ( 'NONE', *, *, #55327, .F. ) ;
#66345=CARTESIAN_POINT ( 'NONE',  ( -36.52772323645827868, 26.41323893245353105, -10.00000000000000000 ) ) ;
#66347=CARTESIAN_POINT ( 'NONE',  ( -19.65312891409030271, 93.06504152958497400, 177.5919119679930134 ) ) ;
#66352=ORIENTED_EDGE ( 'NONE', *, *, #19842, .F. ) ;
#66357=DIRECTION ( 'NONE',  ( 1.000000000000000000, 0.000000000000000000, 0.000000000000000000 ) ) ;
#66358=ORIENTED_EDGE ( 'NONE', *, *, #85698, .T. ) ;
#66361=FACE_OUTER_BOUND ( 'NONE', #53267, .T. ) ;
#66371=DIRECTION ( 'NONE',  ( -1.000000000000000000, 0.000000000000000000, 0.000000000000000000 ) ) ;
#66377=EDGE_CURVE ( 'NONE', #81256, #24137, #73231, .T. ) ;
#66378=VERTEX_POINT ( 'NONE', #21512 ) ;
#66381=ORIENTED_EDGE ( 'NONE', *, *, #89652, .T. ) ;
#66383=CARTESIAN_POINT ( 'NONE',  ( -30.18034446749236821, 25.12100238203590763, -10.00000000000000000 ) ) ;
#66385=VERTEX_POINT ( 'NONE', #5805 ) ;
#66395=FACE_OUTER_BOUND ( 'NONE', #19197, .T. ) ;
#66397=CARTESIAN_POINT ( 'NONE',  ( -0.4668637173180778532, 25.74574839753308808, 177.5919119679930134 ) ) ;
#66403=VERTEX_POINT ( 'NONE', #35709 ) ;
#66404=FACE_OUTER_BOUND ( 'NONE', #94930, .T. ) ;
#66411=ADVANCED_FACE ( 'NONE', ( #91437 ), #6305, .F. ) ;
#66418=LINE ( 'NONE', #35515, #93228 ) ;
#66419=DIRECTION ( 'NONE',  ( -0.000000000000000000, 0.000000000000000000, -1.000000000000000000 ) ) ;
#66420=LINE ( 'NONE', #37006, #7834 ) ;
#66425=EDGE_CURVE ( 'NONE', #34863, #83781, #90463, .T. ) ;
#66429=DIRECTION ( 'NONE',  ( 0.000000000000000000, 0.000000000000000000, 1.000000000000000000 ) ) ;
#66432=AXIS2_PLACEMENT_3D ( 'NONE', #54418, #8843, #94483 ) ;
#66436=CARTESIAN_POINT ( 'NONE',  ( 47.57035326562169075, 72.63383583914733777, 10.00000000000000000 ) ) ;
#66437=ORIENTED_EDGE ( 'NONE', *, *, #61527, .T. ) ;
#66438=ADVANCED_FACE ( 'NONE', ( #52893 ), #83845, .F. ) ;
#66470=DIRECTION ( 'NONE',  ( -0.4829524219151362097, 0.8756465943326133816, 0.000000000000000000 ) ) ;
#66474=PLANE ( 'NONE',  #48911 ) ;
#66485=EDGE_LOOP ( 'NONE', ( #18859, #42037, #88223, #1595 ) ) ;
#66488=CARTESIAN_POINT ( 'NONE',  ( -19.65312891409030271, 93.06504152958497400, 59.99999999999999289 ) ) ;
#66489=ORIENTED_EDGE ( 'NONE', *, *, #82884, .T. ) ;
#66494=EDGE_CURVE ( 'NONE', #12428, #20062, #198, .T. ) ;
#66495=ORIENTED_EDGE ( 'NONE', *, *, #36089, .F. ) ;
#66499=VERTEX_POINT ( 'NONE', #62994 ) ;
#66502=ADVANCED_FACE ( 'NONE', ( #93435 ), #31577, .F. ) ;
#66505=VERTEX_POINT ( 'NONE', #54367 ) ;
#66510=DIRECTION ( 'NONE',  ( -0.000000000000000000, 0.000000000000000000, -1.000000000000000000 ) ) ;
#66517=VERTEX_POINT ( 'NONE', #30601 ) ;
#66521=CARTESIAN_POINT ( 'NONE',  ( -19.65312891409030271, 93.06504152958497400, 10.00000000000000888 ) ) ;
#66524=LINE ( 'NONE', #49453, #44666 ) ;
#66529=ADVANCED_FACE ( 'NONE', ( #39664 ), #78209, .F. ) ;
#66534=VERTEX_POINT ( 'NONE', #70588 ) ;
#66547=EDGE_LOOP ( 'NONE', ( #29500, #95966, #75124, #42050 ) ) ;
#66557=EDGE_CURVE ( 'NONE', #91721, #44730, #48303, .T. ) ;
#66562=EDGE_CURVE ( 'NONE', #55017, #48579, #3227, .T. ) ;
#66568=CARTESIAN_POINT ( 'NONE',  ( -19.73169950930824967, 92.94697205762078340, 59.99999999999999289 ) ) ;
#66579=LINE ( 'NONE', #34676, #48197 ) ;
#66610=ORIENTED_EDGE ( 'NONE', *, *, #99511, .F. ) ;
#66620=EDGE_LOOP ( 'NONE', ( #4567, #2487, #27160, #9472 ) ) ;
#66624=ORIENTED_EDGE ( 'NONE', *, *, #75974, .F. ) ;
#66626=VERTEX_POINT ( 'NONE', #42671 ) ;
#66632=DIRECTION ( 'NONE',  ( 0.000000000000000000, 0.000000000000000000, 1.000000000000000000 ) ) ;
#66643=ORIENTED_EDGE ( 'NONE', *, *, #67651, .T. ) ;
#66654=ORIENTED_EDGE ( 'NONE', *, *, #84765, .T. ) ;
#66656=EDGE_LOOP ( 'NONE', ( #40806, #1220, #97073, #21750 ) ) ;
#66657=DIRECTION ( 'NONE',  ( 1.000000000000000000, 0.000000000000000000, 0.000000000000000000 ) ) ;
#66659=DIRECTION ( 'NONE',  ( 0.5346708562973920831, 0.8450603975019853609, 0.000000000000000000 ) ) ;
#66664=CARTESIAN_POINT ( 'NONE',  ( -4.429217378738782962, 26.01694505731172313, -10.00000000000000000 ) ) ;
#66665=ORIENTED_EDGE ( 'NONE', *, *, #60060, .T. ) ;
#66667=CARTESIAN_POINT ( 'NONE',  ( 41.10245927640360009, 127.8322459559854138, -10.00000000000000000 ) ) ;
#66668=CARTESIAN_POINT ( 'NONE',  ( -49.78034631855286563, 29.87998972566340683, 10.00000000000000000 ) ) ;
#66673=CARTESIAN_POINT ( 'NONE',  ( 29.59124024723001867, 43.31574901297116043, -10.00000000000000000 ) ) ;
#66683=LINE ( 'NONE', #51483, #1174 ) ;
#66705=DIRECTION ( 'NONE',  ( 0.3595896960900372696, 0.9331105242498740626, 0.000000000000000000 ) ) ;
#66713=LINE ( 'NONE', #59089, #11309 ) ;
#66726=ORIENTED_EDGE ( 'NONE', *, *, #91616, .T. ) ;
#66729=DIRECTION ( 'NONE',  ( 0.000000000000000000, 0.000000000000000000, 1.000000000000000000 ) ) ;
#66736=ORIENTED_EDGE ( 'NONE', *, *, #95076, .F. ) ;
#66737=ORIENTED_EDGE ( 'NONE', *, *, #99511, .T. ) ;
#66738=CARTESIAN_POINT ( 'NONE',  ( -19.65312891409030271, 93.06504152958497400, -10.00000000000000888 ) ) ;
#66740=DIRECTION ( 'NONE',  ( -0.5270369400482041167, -0.8498423758701525443, 0.000000000000000000 ) ) ;
#66748=DIRECTION ( 'NONE',  ( 0.000000000000000000, 0.000000000000000000, 1.000000000000000000 ) ) ;
#66755=AXIS2_PLACEMENT_3D ( 'NONE', #15592, #78430, #1921 ) ;
#66757=EDGE_LOOP ( 'NONE', ( #78448, #12830, #54269, #19557 ) ) ;
#66762=DIRECTION ( 'NONE',  ( 0.000000000000000000, 0.000000000000000000, 1.000000000000000000 ) ) ;
#66770=LINE ( 'NONE', #11600, #33311 ) ;
#66774=AXIS2_PLACEMENT_3D ( 'NONE', #72031, #79665, #79162 ) ;
#66784=CARTESIAN_POINT ( 'NONE',  ( 48.74043828842093262, 100.0309547576005258, -10.00000000000000000 ) ) ;
#66791=EDGE_CURVE ( 'NONE', #12449, #56928, #90417, .T. ) ;
#66806=ORIENTED_EDGE ( 'NONE', *, *, #50984, .T. ) ;
#66807=DIRECTION ( 'NONE',  ( 0.000000000000000000, -0.000000000000000000, 1.000000000000000000 ) ) ;
#66809=CARTESIAN_POINT ( 'NONE',  ( -71.61465314115659453, 63.06504152958490295, -40.00000000000000000 ) ) ;
#66829=VERTEX_POINT ( 'NONE', #50659 ) ;
#66838=LINE ( 'NONE', #51651, #83080 ) ;
#66842=DIRECTION ( 'NONE',  ( 0.4525327339300069251, -0.8917477921037054722, 0.000000000000000000 ) ) ;
#66853=VERTEX_POINT ( 'NONE', #74984 ) ;
#66868=EDGE_LOOP ( 'NONE', ( #70484, #24985, #42357, #33474 ) ) ;
#66869=ORIENTED_EDGE ( 'NONE', *, *, #80451, .F. ) ;
#66874=CARTESIAN_POINT ( 'NONE',  ( 39.20103187901341357, 54.69033006916458106, -10.00000000000000000 ) ) ;
#66897=ORIENTED_EDGE ( 'NONE', *, *, #53823, .T. ) ;
#66898=CARTESIAN_POINT ( 'NONE',  ( -61.39381520214497101, 38.43978098112751951, -10.00000000000000000 ) ) ;
#66901=CARTESIAN_POINT ( 'NONE',  ( 40.08283240419611815, 56.57374221892477806, 10.00000000000000000 ) ) ;
#66903=DIRECTION ( 'NONE',  ( -0.7005979833698863235, -0.7135562106085605594, 0.000000000000000000 ) ) ;
#66904=ORIENTED_EDGE ( 'NONE', *, *, #51004, .F. ) ;
#66927=EDGE_CURVE ( 'NONE', #29146, #81396, #90213, .T. ) ;
#66938=EDGE_CURVE ( 'NONE', #10169, #28472, #51677, .T. ) ;
#66959=ORIENTED_EDGE ( 'NONE', *, *, #32610, .T. ) ;
#66963=ORIENTED_EDGE ( 'NONE', *, *, #62397, .T. ) ;
#66968=AXIS2_PLACEMENT_3D ( 'NONE', #84480, #76832, #22143 ) ;
#66970=ORIENTED_EDGE ( 'NONE', *, *, #33960, .F. ) ;
#66975=ORIENTED_EDGE ( 'NONE', *, *, #35203, .F. ) ;
#66980=PLANE ( 'NONE',  #3800 ) ;
#66981=CIRCLE ( 'NONE', #44344, 70.00000000000001421 ) ;
#66983=EDGE_LOOP ( 'NONE', ( #72647, #82661, #87994, #34728 ) ) ;
#66987=ORIENTED_EDGE ( 'NONE', *, *, #54191, .F. ) ;
#66990=EDGE_LOOP ( 'NONE', ( #5487, #42894, #55368, #78982 ) ) ;
#67010=LINE ( 'NONE', #98440, #59600 ) ;
#67014=CARTESIAN_POINT ( 'NONE',  ( 11.47080329375824981, 30.07510926853015221, 10.00000000000000000 ) ) ;
#67023=CARTESIAN_POINT ( 'NONE',  ( 45.57373283677818421, 114.7827874512443032, 10.00000000000000000 ) ) ;
#67034=DIRECTION ( 'NONE',  ( -0.6386832404231509441, -0.7694697644498993405, 0.000000000000000000 ) ) ;
#67042=VECTOR ( 'NONE', #70791, 1000.000000000000000 ) ;
#67048=VERTEX_POINT ( 'NONE', #14168 ) ;
#67050=VECTOR ( 'NONE', #80077, 1000.000000000000000 ) ;
#67053=ADVANCED_FACE ( 'NONE', ( #12181 ), #98790, .T. ) ;
#67056=PLANE ( 'NONE',  #92077 ) ;
#67061=DIRECTION ( 'NONE',  ( -0.5891075386695772131, -0.8080546441192405505, 0.000000000000000000 ) ) ;
#67069=CARTESIAN_POINT ( 'NONE',  ( -19.78514814072851280, 93.11685525788735163, 59.99999999999999289 ) ) ;
#67094=DIRECTION ( 'NONE',  ( -0.9689225787001356505, 0.2473641778533816060, 0.000000000000000000 ) ) ;
#67111=VERTEX_POINT ( 'NONE', #88901 ) ;
#67113=ORIENTED_EDGE ( 'NONE', *, *, #69198, .T. ) ;
#67116=LINE ( 'NONE', #90480, #20743 ) ;
#67127=CIRCLE ( 'NONE', #63878, 70.00000000000001421 ) ;
#67134=ORIENTED_EDGE ( 'NONE', *, *, #71824, .T. ) ;
#67138=ORIENTED_EDGE ( 'NONE', *, *, #10119, .T. ) ;
#67150=CARTESIAN_POINT ( 'NONE',  ( 28.00427808217458647, 41.79349426999503692, 10.00000000000000000 ) ) ;
#67154=CARTESIAN_POINT ( 'NONE',  ( 45.56181175559623142, 118.5014625327306135, 177.5919119679930134 ) ) ;
#67166=DIRECTION ( 'NONE',  ( -0.000000000000000000, -0.000000000000000000, -1.000000000000000000 ) ) ;
#67168=CARTESIAN_POINT ( 'NONE',  ( -19.65312891409030271, 93.06504152958497400, 10.00000000000000888 ) ) ;
#67180=DIRECTION ( 'NONE',  ( -0.5369817302126890235, 0.8435938723211464652, 0.000000000000000000 ) ) ;
#67186=LINE ( 'NONE', #5893, #86959 ) ;
#67191=EDGE_CURVE ( 'NONE', #33084, #74024, #9091, .T. ) ;
#67199=CARTESIAN_POINT ( 'NONE',  ( -58.62427208439002158, 70.56504152958493137, -45.00000000000001421 ) ) ;
#67205=DIRECTION ( 'NONE',  ( -0.9974094913373522386, -0.07193265315671491800, 0.000000000000000000 ) ) ;
#67206=CARTESIAN_POINT ( 'NONE',  ( -40.60196443811259570, 67.26451206140657746, -10.00000000000000000 ) ) ;
#67209=EDGE_CURVE ( 'NONE', #48279, #88645, #95237, .T. ) ;
#67213=LINE ( 'NONE', #5919, #98660 ) ;
#67216=EDGE_LOOP ( 'NONE', ( #72644, #57014, #51426, #25512 ) ) ;
#67218=ORIENTED_EDGE ( 'NONE', *, *, #47331, .F. ) ;
#67221=ORIENTED_EDGE ( 'NONE', *, *, #39507, .F. ) ;
#67224=CARTESIAN_POINT ( 'NONE',  ( -2.590881078880516331, 25.17631125121047475, -10.00000000000000000 ) ) ;
#67229=AXIS2_PLACEMENT_3D ( 'NONE', #96241, #26801, #57685 ) ;
#67231=CARTESIAN_POINT ( 'NONE',  ( -19.65312891409030271, 93.06504152958497400, 10.00000000000000888 ) ) ;
#67235=ORIENTED_EDGE ( 'NONE', *, *, #43248, .T. ) ;
#67248=EDGE_CURVE ( 'NONE', #6051, #18914, #63783, .T. ) ;
#67250=ORIENTED_EDGE ( 'NONE', *, *, #47420, .F. ) ;
#67254=VERTEX_POINT ( 'NONE', #57670 ) ;
#67255=AXIS2_PLACEMENT_3D ( 'NONE', #94229, #25283, #79022 ) ;
#67262=CARTESIAN_POINT ( 'NONE',  ( -46.49770490450612215, 29.77544742692501600, 10.00000000000000000 ) ) ;
#67264=VECTOR ( 'NONE', #88289, 1000.000000000000114 ) ;
#67265=VERTEX_POINT ( 'NONE', #13100 ) ;
#67267=ORIENTED_EDGE ( 'NONE', *, *, #51786, .T. ) ;
#67268=CARTESIAN_POINT ( 'NONE',  ( -19.65312891409030271, 93.06504152958497400, 10.00000000000000888 ) ) ;
#67270=DIRECTION ( 'NONE',  ( 0.5864613938488598688, -0.8099771808667527440, 0.000000000000000000 ) ) ;
#67273=DIRECTION ( 'NONE',  ( -0.9538480676139692305, 0.3002896333693469422, 0.000000000000000000 ) ) ;
#67274=ORIENTED_EDGE ( 'NONE', *, *, #61318, .F. ) ;
#67305=CARTESIAN_POINT ( 'NONE',  ( -71.61465314115659453, 63.06504152958490295, 20.00000000000001776 ) ) ;
#67312=CARTESIAN_POINT ( 'NONE',  ( -8.669243101527598583, 25.19333184544593252, 10.00000000000000000 ) ) ;
#67320=EDGE_CURVE ( 'NONE', #44730, #16478, #35873, .T. ) ;
#67323=DIRECTION ( 'NONE',  ( -0.9839629614562445115, 0.1783728972749415165, 0.000000000000000000 ) ) ;
#67329=ORIENTED_EDGE ( 'NONE', *, *, #68019, .T. ) ;
#67331=ORIENTED_EDGE ( 'NONE', *, *, #3345, .F. ) ;
#67351=EDGE_CURVE ( 'NONE', #42396, #20252, #53560, .T. ) ;
#67364=CARTESIAN_POINT ( 'NONE',  ( 46.88368875251780565, 110.3874725885333135, 10.00000000000000000 ) ) ;
#67368=CARTESIAN_POINT ( 'NONE',  ( 15.36455789491911794, 32.15369338429142942, -10.00000000000000000 ) ) ;
#67369=VECTOR ( 'NONE', #70244, 1000.000000000000000 ) ;
#67372=FACE_BOUND ( 'NONE', #7117, .T. ) ;
#67378=AXIS2_PLACEMENT_3D ( 'NONE', #59641, #99665, #75376 ) ;
#67401=VECTOR ( 'NONE', #9072, 1000.000000000000000 ) ;
#67403=CARTESIAN_POINT ( 'NONE',  ( 24.35067441160642687, 40.23626134430271861, 10.00000000000000000 ) ) ;
#67406=CARTESIAN_POINT ( 'NONE',  ( -56.16025090550425602, 33.03454289568183100, 10.00000000000000000 ) ) ;
#67411=FACE_OUTER_BOUND ( 'NONE', #33992, .T. ) ;
#67417=LINE ( 'NONE', #61309, #58204 ) ;
#67429=DIRECTION ( 'NONE',  ( 0.000000000000000000, 0.000000000000000000, 1.000000000000000000 ) ) ;
#67431=DIRECTION ( 'NONE',  ( -0.6623377501714446947, 0.7492053821869066876, 0.000000000000000000 ) ) ;
#67432=VECTOR ( 'NONE', #8939, 1000.000000000000000 ) ;
#67438=EDGE_CURVE ( 'NONE', #94399, #37194, #38354, .T. ) ;
#67439=AXIS2_PLACEMENT_3D ( 'NONE', #88024, #18573, #9971 ) ;
#67442=CARTESIAN_POINT ( 'NONE',  ( 38.52196584993465223, 56.41980893122115504, -10.00000000000000000 ) ) ;
#67463=DIRECTION ( 'NONE',  ( -1.000000000000000000, 0.000000000000000000, 0.000000000000000000 ) ) ;
#67464=CARTESIAN_POINT ( 'NONE',  ( -50.26415955272096880, 51.36194717159466450, 59.99999999999999289 ) ) ;
#67469=CARTESIAN_POINT ( 'NONE',  ( 29.13110022456613635, 42.86445400964586838, 177.5919119679930134 ) ) ;
#67472=EDGE_LOOP ( 'NONE', ( #5252, #80817, #27041, #74755 ) ) ;
#67473=ORIENTED_EDGE ( 'NONE', *, *, #4231, .F. ) ;
#67477=ORIENTED_EDGE ( 'NONE', *, *, #44629, .F. ) ;
#67480=DIRECTION ( 'NONE',  ( -0.5634352399127592337, -0.8261602328994366307, 0.000000000000000000 ) ) ;
#67481=ORIENTED_EDGE ( 'NONE', *, *, #82257, .T. ) ;
#67493=CARTESIAN_POINT ( 'NONE',  ( -52.88606886026012432, 92.76052029034119073, -10.00000000000000000 ) ) ;
#67506=VECTOR ( 'NONE', #19484, 1000.000000000000000 ) ;
#67507=ADVANCED_FACE ( 'NONE', ( #8473 ), #372, .F. ) ;
#67509=DIRECTION ( 'NONE',  ( -0.4245406647209920559, -0.9054088711727195093, 0.000000000000000000 ) ) ;
#67510=DIRECTION ( 'NONE',  ( -0.5696381972391160176, 0.8218955677251033043, 0.000000000000000000 ) ) ;
#67521=ORIENTED_EDGE ( 'NONE', *, *, #23962, .F. ) ;
#67523=AXIS2_PLACEMENT_3D ( 'NONE', #45955, #53568, #9490 ) ;
#67535=CIRCLE ( 'NONE', #19051, 70.00000000000001421 ) ;
#67556=CARTESIAN_POINT ( 'NONE',  ( 30.62489312496363425, 46.16797101519271962, -10.00000000000000000 ) ) ;
#67557=ADVANCED_FACE ( 'NONE', ( #82906 ), #66170, .F. ) ;
#67561=LINE ( 'NONE', #83306, #68283 ) ;
#67566=VECTOR ( 'NONE', #97145, 1000.000000000000000 ) ;
#67572=CARTESIAN_POINT ( 'NONE',  ( 25.34687108590969729, 93.06504152958497400, 60.00000000000000000 ) ) ;
#67589=LINE ( 'NONE', #29596, #39069 ) ;
#67603=DIRECTION ( 'NONE',  ( 0.7893155279419866721, 0.6139877827364833562, 0.000000000000000000 ) ) ;
#67604=VECTOR ( 'NONE', #43668, 1000.000000000000000 ) ;
#67606=FACE_OUTER_BOUND ( 'NONE', #96306, .T. ) ;
#67607=VERTEX_POINT ( 'NONE', #4367 ) ;
#67611=DIRECTION ( 'NONE',  ( -0.000000000000000000, -0.000000000000000000, -1.000000000000000000 ) ) ;
#67623=CARTESIAN_POINT ( 'NONE',  ( 19.18375657693640335, 36.32959363016014720, -10.00000000000000000 ) ) ;
#67632=ADVANCED_FACE ( 'NONE', ( #51966 ), #6366, .F. ) ;
#67635=EDGE_LOOP ( 'NONE', ( #97888, #40155, #18702, #34118, #81517 ) ) ;
#67637=EDGE_CURVE ( 'NONE', #16766, #41280, #6343, .T. ) ;
#67642=CARTESIAN_POINT ( 'NONE',  ( 41.19957572438558913, 58.46810036157969392, -10.00000000000000000 ) ) ;
#67648=ORIENTED_EDGE ( 'NONE', *, *, #43563, .T. ) ;
#67649=CIRCLE ( 'NONE', #96762, 0.1418229129680897982 ) ;
#67650=CARTESIAN_POINT ( 'NONE',  ( -19.65312891409030271, 93.06504152958497400, 60.00000000000000000 ) ) ;
#67651=EDGE_CURVE ( 'NONE', #70217, #26616, #14463, .T. ) ;
#67663=CIRCLE ( 'NONE', #49870, 70.00000000000001421 ) ;
#67665=PLANE ( 'NONE',  #56449 ) ;
#67666=CARTESIAN_POINT ( 'NONE',  ( 9.476883925432959543, 29.12856466152289414, -10.00000000000000000 ) ) ;
#67669=CARTESIAN_POINT ( 'NONE',  ( -51.16543076746616947, 82.50588140424335393, -10.00000000000000000 ) ) ;
#67671=VECTOR ( 'NONE', #59695, 999.9999999999998863 ) ;
#67680=DIRECTION ( 'NONE',  ( -0.9979227057047524996, 0.06442261589617470641, 0.000000000000000000 ) ) ;
#67684=LINE ( 'NONE', #98614, #84045 ) ;
#67692=EDGE_CURVE ( 'NONE', #30899, #5086, #53439, .T. ) ;
#67694=CARTESIAN_POINT ( 'NONE',  ( -32.23964971562050863, 42.88792865763274875, 59.99999999999999289 ) ) ;
#67715=ADVANCED_FACE ( 'NONE', ( #18838 ), #58794, .F. ) ;
#67720=DIRECTION ( 'NONE',  ( -0.000000000000000000, 0.000000000000000000, -1.000000000000000000 ) ) ;
#67722=EDGE_LOOP ( 'NONE', ( #42315, #82774, #85478, #48728 ) ) ;
#67725=ORIENTED_EDGE ( 'NONE', *, *, #82936, .T. ) ;
#67728=ORIENTED_EDGE ( 'NONE', *, *, #54218, .F. ) ;
#67731=VECTOR ( 'NONE', #96275, 1000.000000000000000 ) ;
#67738=VECTOR ( 'NONE', #70199, 1000.000000000000114 ) ;
#67743=ORIENTED_EDGE ( 'NONE', *, *, #88222, .F. ) ;
#67747=VECTOR ( 'NONE', #295, 1000.000000000000000 ) ;
#67759=CARTESIAN_POINT ( 'NONE',  ( -19.65312891409030271, 93.06504152958497400, 177.5919119679930134 ) ) ;
#67763=AXIS2_PLACEMENT_3D ( 'NONE', #55318, #96878, #57822 ) ;
#67767=CARTESIAN_POINT ( 'NONE',  ( -19.65312891409030271, 93.06504152958497400, 20.00000000000000355 ) ) ;
#67770=LINE ( 'NONE', #29275, #36647 ) ;
#67771=ORIENTED_EDGE ( 'NONE', *, *, #82938, .F. ) ;
#67772=VERTEX_POINT ( 'NONE', #57314 ) ;
#67773=CARTESIAN_POINT ( 'NONE',  ( 33.23512877817899636, 89.27284934918669990, 59.99999999999999289 ) ) ;
#67777=DIRECTION ( 'NONE',  ( -0.9805290675673918876, -0.1963739994383708332, 0.000000000000000000 ) ) ;
#67781=FACE_OUTER_BOUND ( 'NONE', #996, .T. ) ;
#67788=ADVANCED_FACE ( 'NONE', ( #58309 ), #89286, .F. ) ;
#67798=DIRECTION ( 'NONE',  ( 0.000000000000000000, 0.000000000000000000, 1.000000000000000000 ) ) ;
#67799=AXIS2_PLACEMENT_3D ( 'NONE', #54326, #85822, #10261 ) ;
#67801=AXIS2_PLACEMENT_3D ( 'NONE', #73293, #49473, #19610 ) ;
#67802=VECTOR ( 'NONE', #37369, 1000.000000000000000 ) ;
#67814=ADVANCED_FACE ( 'NONE', ( #3270 ), #71163, .T. ) ;
#67817=EDGE_CURVE ( 'NONE', #27077, #16029, #65045, .T. ) ;
#67818=CARTESIAN_POINT ( 'NONE',  ( -61.08640853961129835, 36.64444830801921427, -10.00000000000000000 ) ) ;
#67824=DIRECTION ( 'NONE',  ( -1.000000000000000000, 0.000000000000000000, 0.000000000000000000 ) ) ;
#67847=CARTESIAN_POINT ( 'NONE',  ( -19.65312891409030271, 93.06504152958497400, -10.00000000000000888 ) ) ;
#67849=CARTESIAN_POINT ( 'NONE',  ( 33.21408624426133827, 88.98998513028048762, 59.99999999999999289 ) ) ;
#67851=DIRECTION ( 'NONE',  ( -0.4897629171537585258, 0.8718556560469402639, 0.000000000000000000 ) ) ;
#67860=PLANE ( 'NONE',  #54473 ) ;
#67861=ORIENTED_EDGE ( 'NONE', *, *, #186, .T. ) ;
#67862=ORIENTED_EDGE ( 'NONE', *, *, #54218, .T. ) ;
#67864=DIRECTION ( 'NONE',  ( -1.000000000000000000, 0.000000000000000000, 0.000000000000000000 ) ) ;
#67874=ORIENTED_EDGE ( 'NONE', *, *, #40393, .F. ) ;
#67876=CARTESIAN_POINT ( 'NONE',  ( -6.281727404287059890, 25.63055774385195917, 10.00000000000000000 ) ) ;
#67877=VERTEX_POINT ( 'NONE', #67023 ) ;
#67878=AXIS2_PLACEMENT_3D ( 'NONE', #25857, #71954, #63336 ) ;
#67881=EDGE_LOOP ( 'NONE', ( #84605, #90352, #82591, #25750 ) ) ;
#67890=EDGE_LOOP ( 'NONE', ( #40041, #83010, #62350, #18449 ) ) ;
#67891=AXIS2_PLACEMENT_3D ( 'NONE', #10995, #34273, #26673 ) ;
#67898=CIRCLE ( 'NONE', #74433, 70.00000000000001421 ) ;
#67923=DIRECTION ( 'NONE',  ( 0.000000000000000000, -0.000000000000000000, 1.000000000000000000 ) ) ;
#67925=LINE ( 'NONE', #97848, #77404 ) ;
#67944=ADVANCED_FACE ( 'NONE', ( #74159 ), #21434, .F. ) ;
#67947=AXIS2_PLACEMENT_3D ( 'NONE', #91749, #7107, #92743 ) ;
#67955=FACE_OUTER_BOUND ( 'NONE', #25663, .T. ) ;
#67961=EDGE_CURVE ( 'NONE', #67254, #71229, #75151, .T. ) ;
#67969=ORIENTED_EDGE ( 'NONE', *, *, #98080, .T. ) ;
#67974=ADVANCED_FACE ( 'NONE', ( #12351 ), #5728, .F. ) ;
#67976=ORIENTED_EDGE ( 'NONE', *, *, #5384, .F. ) ;
#67983=DIRECTION ( 'NONE',  ( 0.000000000000000000, 0.000000000000000000, 1.000000000000000000 ) ) ;
#67985=ORIENTED_EDGE ( 'NONE', *, *, #33447, .F. ) ;
#67987=ORIENTED_EDGE ( 'NONE', *, *, #73005, .T. ) ;
#67990=ORIENTED_EDGE ( 'NONE', *, *, #15192, .F. ) ;
#67994=CARTESIAN_POINT ( 'NONE',  ( -8.010917706491644807, 72.92290384248846635, 15.00660040458968503 ) ) ;
#68003=LINE ( 'NONE', #57912, #64190 ) ;
#68009=DIRECTION ( 'NONE',  ( -0.8452030915256490973, -0.5344452582589588330, 0.000000000000000000 ) ) ;
#68013=LINE ( 'NONE', #29520, #72349 ) ;
#68018=DIRECTION ( 'NONE',  ( 0.000000000000000000, -0.000000000000000000, -1.000000000000000000 ) ) ;
#68019=EDGE_CURVE ( 'NONE', #20265, #32467, #35634, .T. ) ;
#68021=EDGE_CURVE ( 'NONE', #31449, #94911, #27559, .T. ) ;
#68023=AXIS2_PLACEMENT_3D ( 'NONE', #50701, #21315, #42596 ) ;
#68026=CARTESIAN_POINT ( 'NONE',  ( -46.31994871380127421, 28.06264584988120347, -10.00000000000000000 ) ) ;
#68063=VERTEX_POINT ( 'NONE', #9097 ) ;
#68068=DIRECTION ( 'NONE',  ( -0.5951734788405994570, 0.8035972437015811431, 0.000000000000000000 ) ) ;
#68082=VERTEX_POINT ( 'NONE', #26795 ) ;
#68083=LINE ( 'NONE', #43279, #73217 ) ;
#68091=VECTOR ( 'NONE', #83335, 1000.000000000000000 ) ;
#68099=DIRECTION ( 'NONE',  ( -0.000000000000000000, -0.000000000000000000, -1.000000000000000000 ) ) ;
#68111=ORIENTED_EDGE ( 'NONE', *, *, #34398, .T. ) ;
#68113=ORIENTED_EDGE ( 'NONE', *, *, #24339, .F. ) ;
#68117=DIRECTION ( 'NONE',  ( -0.000000000000000000, -0.000000000000000000, 1.000000000000000000 ) ) ;
#68118=ORIENTED_EDGE ( 'NONE', *, *, #26811, .T. ) ;
#68120=CARTESIAN_POINT ( 'NONE',  ( -77.42978507651396569, 55.80833764325424085, 10.00000000000000000 ) ) ;
#68124=EDGE_LOOP ( 'NONE', ( #84121, #49935, #12444, #30374 ) ) ;
#68143=EDGE_CURVE ( 'NONE', #1972, #50533, #50093, .T. ) ;
#68148=DIRECTION ( 'NONE',  ( -0.8769651246872975925, 0.4805540241036304061, 0.000000000000000000 ) ) ;
#68156=PLANE ( 'NONE',  #86917 ) ;
#68165=DIRECTION ( 'NONE',  ( -0.000000000000000000, -0.000000000000000000, -1.000000000000000000 ) ) ;
#68187=DIRECTION ( 'NONE',  ( 0.000000000000000000, 0.000000000000000000, 1.000000000000000000 ) ) ;
#68193=ORIENTED_EDGE ( 'NONE', *, *, #74668, .F. ) ;
#68209=VERTEX_POINT ( 'NONE', #66784 ) ;
#68211=EDGE_CURVE ( 'NONE', #93198, #28495, #6977, .T. ) ;
#68225=ORIENTED_EDGE ( 'NONE', *, *, #14955, .F. ) ;
#68226=VECTOR ( 'NONE', #21988, 1000.000000000000227 ) ;
#68237=CARTESIAN_POINT ( 'NONE',  ( -19.65312891409030271, 93.06504152958497400, -10.00000000000000888 ) ) ;
#68242=ORIENTED_EDGE ( 'NONE', *, *, #13551, .T. ) ;
#68243=LINE ( 'NONE', #22155, #96578 ) ;
#68253=DIRECTION ( 'NONE',  ( 0.2500151307524129951, -0.9682419296822740717, 0.000000000000000000 ) ) ;
#68254=ORIENTED_EDGE ( 'NONE', *, *, #21058, .T. ) ;
#68257=DIRECTION ( 'NONE',  ( -0.3986482622784180974, -0.9171038997749370036, 0.000000000000000000 ) ) ;
#68270=ORIENTED_EDGE ( 'NONE', *, *, #86864, .F. ) ;
#68278=LINE ( 'NONE', #37373, #71160 ) ;
#68283=VECTOR ( 'NONE', #82331, 1000.000000000000000 ) ;
#68287=CARTESIAN_POINT ( 'NONE',  ( 47.96820964746023463, 80.67316705762479501, 10.00000000000000000 ) ) ;
#68290=CARTESIAN_POINT ( 'NONE',  ( -60.12289532704065920, 50.57929518357629206, 59.99999999999999289 ) ) ;
#68292=DIRECTION ( 'NONE',  ( -1.000000000000000000, 0.000000000000000000, 0.000000000000000000 ) ) ;
#68295=DIRECTION ( 'NONE',  ( 0.000000000000000000, 0.000000000000000000, 1.000000000000000000 ) ) ;
#68310=CARTESIAN_POINT ( 'NONE',  ( 40.08283240419611815, 56.57374221892477806, -10.00000000000000000 ) ) ;
#68315=CARTESIAN_POINT ( 'NONE',  ( -64.94778771796556782, 41.33875607593970614, 10.00000000000000000 ) ) ;
#68323=ORIENTED_EDGE ( 'NONE', *, *, #53266, .T. ) ;
#68326=EDGE_CURVE ( 'NONE', #70323, #55128, #4373, .T. ) ;
#68330=CARTESIAN_POINT ( 'NONE',  ( -19.65312891409030271, 93.06504152958497400, -10.00000000000000888 ) ) ;
#68341=EDGE_CURVE ( 'NONE', #48849, #20062, #36262, .T. ) ;
#68349=DIRECTION ( 'NONE',  ( -0.9991767892008870389, -0.04056776950001317328, 0.000000000000000000 ) ) ;
#68350=CARTESIAN_POINT ( 'NONE',  ( 42.55442611339157821, 60.96799964870728417, -10.00000000000000000 ) ) ;
#68357=AXIS2_PLACEMENT_3D ( 'NONE', #57423, #66035, #82283 ) ;
#68360=ORIENTED_EDGE ( 'NONE', *, *, #20933, .T. ) ;
#68365=CARTESIAN_POINT ( 'NONE',  ( -38.42080210277662644, 44.85759688798118816, 59.99999999999999289 ) ) ;
#68366=ORIENTED_EDGE ( 'NONE', *, *, #51003, .F. ) ;
#68377=ORIENTED_EDGE ( 'NONE', *, *, #41367, .T. ) ;
#68378=EDGE_CURVE ( 'NONE', #47742, #17718, #74798, .T. ) ;
#68382=EDGE_CURVE ( 'NONE', #58260, #79765, #51467, .T. ) ;
#68385=EDGE_CURVE ( 'NONE', #29620, #37787, #35771, .T. ) ;
#68389=ORIENTED_EDGE ( 'NONE', *, *, #91671, .T. ) ;
#68391=ADVANCED_FACE ( 'NONE', ( #30155 ), #13972, .F. ) ;
#68393=FACE_OUTER_BOUND ( 'NONE', #26771, .T. ) ;
#68396=VERTEX_POINT ( 'NONE', #6856 ) ;
#68400=DIRECTION ( 'NONE',  ( -0.9576970189910627429, -0.2877784213863714968, 0.000000000000000000 ) ) ;
#68403=DIRECTION ( 'NONE',  ( -0.000000000000000000, -0.000000000000000000, -1.000000000000000000 ) ) ;
#68405=AXIS2_PLACEMENT_3D ( 'NONE', #38866, #97344, #82166 ) ;
#68413=CARTESIAN_POINT ( 'NONE',  ( -19.51183051894608766, 93.07722767632783700, 59.99999999999999289 ) ) ;
#68418=DIRECTION ( 'NONE',  ( 0.000000000000000000, -0.000000000000000000, -1.000000000000000000 ) ) ;
#68433=LINE ( 'NONE', #67442, #91162 ) ;
#68440=DIRECTION ( 'NONE',  ( -0.8452030915256490973, -0.5344452582589588330, 0.000000000000000000 ) ) ;
#68456=ADVANCED_FACE ( 'NONE', ( #44849 ), #67665, .F. ) ;
#68461=EDGE_CURVE ( 'NONE', #95115, #78977, #43359, .T. ) ;
#68464=VERTEX_POINT ( 'NONE', #21573 ) ;
#68466=DIRECTION ( 'NONE',  ( -0.000000000000000000, -0.000000000000000000, -1.000000000000000000 ) ) ;
#68472=ORIENTED_EDGE ( 'NONE', *, *, #89040, .F. ) ;
#68477=VERTEX_POINT ( 'NONE', #66667 ) ;
#68480=AXIS2_PLACEMENT_3D ( 'NONE', #80085, #26847, #96277 ) ;
#68481=EDGE_LOOP ( 'NONE', ( #94230, #87265, #52138, #41912 ) ) ;
#68483=CARTESIAN_POINT ( 'NONE',  ( -10.53546450992863370, 72.07795844810249264, 14.77482737668580270 ) ) ;
#68487=ORIENTED_EDGE ( 'NONE', *, *, #99295, .F. ) ;
#68488=ORIENTED_EDGE ( 'NONE', *, *, #31190, .F. ) ;
#68490=ADVANCED_FACE ( 'NONE', ( #98085 ), #60045, .F. ) ;
#68500=AXIS2_PLACEMENT_3D ( 'NONE', #83848, #4831, #6309 ) ;
#68501=EDGE_CURVE ( 'NONE', #45411, #91719, #22604, .T. ) ;
#68505=LINE ( 'NONE', #99427, #12716 ) ;
#68506=DIRECTION ( 'NONE',  ( -0.2776767122488494333, -0.9606745773021526658, 0.000000000000000000 ) ) ;
#68513=EDGE_CURVE ( 'NONE', #68082, #34660, #59041, .T. ) ;
#68514=DIRECTION ( 'NONE',  ( -0.7226656227773308183, -0.6911977992267138715, 0.000000000000000000 ) ) ;
#68531=CARTESIAN_POINT ( 'NONE',  ( 15.77038241084232517, 34.14663330942826747, -10.00000000000000000 ) ) ;
#68542=ADVANCED_FACE ( 'NONE', ( #6373 ), #37256, .T. ) ;
#68559=MECHANICAL_DESIGN_GEOMETRIC_PRESENTATION_REPRESENTATION('',(#39400),#96104);
#68565=CARTESIAN_POINT ( 'NONE',  ( -52.86010516724736163, 91.71679868308304151, -10.00000000000000000 ) ) ;
#68567=VECTOR ( 'NONE', #97540, 1000.000000000000000 ) ;
#68569=DIRECTION ( 'NONE',  ( -1.000000000000000000, 0.000000000000000000, 0.000000000000000000 ) ) ;
#68571=ORIENTED_EDGE ( 'NONE', *, *, #38722, .T. ) ;
#68577=EDGE_LOOP ( 'NONE', ( #74255, #97787, #69883, #51269 ) ) ;
#68580=CARTESIAN_POINT ( 'NONE',  ( -1.846057691949487101, 43.12070627514476229, 59.99999999999999289 ) ) ;
#68582=LINE ( 'NONE', #21987, #6875 ) ;
#68585=EDGE_CURVE ( 'NONE', #24573, #38349, #38717, .T. ) ;
#68588=EDGE_LOOP ( 'NONE', ( #65716, #6075, #59889, #91964 ) ) ;
#68592=VERTEX_POINT ( 'NONE', #54427 ) ;
#68598=DIRECTION ( 'NONE',  ( -0.6139877827364833562, 0.7893155279419866721, 0.000000000000000000 ) ) ;
#68607=ORIENTED_EDGE ( 'NONE', *, *, #13041, .F. ) ;
#68609=ORIENTED_EDGE ( 'NONE', *, *, #79150, .F. ) ;
#68611=VERTEX_POINT ( 'NONE', #15434 ) ;
#68615=LINE ( 'NONE', #38706, #18660 ) ;
#68631=CARTESIAN_POINT ( 'NONE',  ( -38.35373792487678202, 26.90998726756845727, 10.00000000000000000 ) ) ;
#68635=EDGE_LOOP ( 'NONE', ( #11727, #8439, #77734, #28473 ) ) ;
#68638=FACE_OUTER_BOUND ( 'NONE', #90369, .T. ) ;
#68651=ORIENTED_EDGE ( 'NONE', *, *, #51690, .T. ) ;
#68663=CARTESIAN_POINT ( 'NONE',  ( -19.65312891409030271, 93.06504152958497400, 177.5919119679930134 ) ) ;
#68665=CARTESIAN_POINT ( 'NONE',  ( -7.332799823397643024, 36.44574457902104569, 59.99999999999999289 ) ) ;
#68667=DIRECTION ( 'NONE',  ( -0.000000000000000000, -0.000000000000000000, -1.000000000000000000 ) ) ;
#68675=DIRECTION ( 'NONE',  ( -0.9008877160804935613, -0.4340522123146846045, 0.000000000000000000 ) ) ;
#68680=CARTESIAN_POINT ( 'NONE',  ( 21.13464251418870532, 61.24490853227566589, 59.99999999999999289 ) ) ;
#68685=DIRECTION ( 'NONE',  ( 1.000000000000000000, 0.000000000000000000, 0.000000000000000000 ) ) ;
#68693=EDGE_LOOP ( 'NONE', ( #38059, #30982, #29098, #37835 ) ) ;
#68702=DIRECTION ( 'NONE',  ( 0.000000000000000000, 0.000000000000000000, 1.000000000000000000 ) ) ;
#68711=EDGE_CURVE ( 'NONE', #18010, #566, #85924, .T. ) ;
#68715=DIRECTION ( 'NONE',  ( -0.9862134920484689760, -0.1654779384134469067, 0.000000000000000000 ) ) ;
#68716=LINE ( 'NONE', #30222, #71860 ) ;
#68724=CARTESIAN_POINT ( 'NONE',  ( -27.77457187288641904, 24.79904599702367562, -10.00000000000000000 ) ) ;
#68727=ORIENTED_EDGE ( 'NONE', *, *, #57745, .T. ) ;
#68728=ORIENTED_EDGE ( 'NONE', *, *, #46448, .F. ) ;
#68732=LINE ( 'NONE', #8936, #94495 ) ;
#68745=ORIENTED_EDGE ( 'NONE', *, *, #62082, .F. ) ;
#68752=ORIENTED_EDGE ( 'NONE', *, *, #47659, .F. ) ;
#68754=ORIENTED_EDGE ( 'NONE', *, *, #69079, .T. ) ;
#68755=DIRECTION ( 'NONE',  ( -0.000000000000000000, -0.000000000000000000, 1.000000000000000000 ) ) ;
#68758=EDGE_CURVE ( 'NONE', #50548, #81396, #86417, .T. ) ;
#68761=ADVANCED_FACE ( 'NONE', ( #38508 ), #7116, .F. ) ;
#68762=CARTESIAN_POINT ( 'NONE',  ( 10.06845959268932411, 31.07446838803123157, -10.00000000000000000 ) ) ;
#68766=VERTEX_POINT ( 'NONE', #23812 ) ;
#68771=DIRECTION ( 'NONE',  ( -0.000000000000000000, 0.000000000000000000, -1.000000000000000000 ) ) ;
#68773=CIRCLE ( 'NONE', #52572, 6.749999999999992006 ) ;
#68782=PLANE ( 'NONE',  #80251 ) ;
#68784=AXIS2_PLACEMENT_3D ( 'NONE', #15354, #91924, #23457 ) ;
#68786=CARTESIAN_POINT ( 'NONE',  ( -20.51833308425736391, 22.81063138990083061, 10.00000000000000000 ) ) ;
#68803=CARTESIAN_POINT ( 'NONE',  ( -19.65312891409030271, 93.06504152958497400, 59.99999999999999289 ) ) ;
#68805=FACE_OUTER_BOUND ( 'NONE', #9056, .T. ) ;
#68813=VECTOR ( 'NONE', #92127, 1000.000000000000000 ) ;
#68818=VERTEX_POINT ( 'NONE', #76538 ) ;
#68819=CARTESIAN_POINT ( 'NONE',  ( -72.48190909937208914, 49.06123820388767598, -10.00000000000000000 ) ) ;
#68841=AXIS2_PLACEMENT_3D ( 'NONE', #83979, #99645, #75863 ) ;
#68842=VERTEX_POINT ( 'NONE', #23309 ) ;
#68854=ORIENTED_EDGE ( 'NONE', *, *, #33767, .T. ) ;
#68855=LINE ( 'NONE', #99776, #25206 ) ;
#68860=PLANE ( 'NONE',  #35778 ) ;
#68868=ORIENTED_EDGE ( 'NONE', *, *, #83861, .F. ) ;
#68870=CARTESIAN_POINT ( 'NONE',  ( -19.54717911816667453, 93.15931973166004809, 59.99999999999999289 ) ) ;
#68879=ORIENTED_EDGE ( 'NONE', *, *, #72640, .T. ) ;
#68881=CARTESIAN_POINT ( 'NONE',  ( -5.860417570053906289, 43.20579575138734896, 59.99999999999999289 ) ) ;
#68897=VERTEX_POINT ( 'NONE', #76055 ) ;
#68900=EDGE_CURVE ( 'NONE', #67265, #7039, #6636, .T. ) ;
#68901=VECTOR ( 'NONE', #59925, 1000.000000000000000 ) ;
#68905=DIRECTION ( 'NONE',  ( 0.000000000000000000, 0.000000000000000000, 1.000000000000000000 ) ) ;
#68907=EDGE_CURVE ( 'NONE', #27844, #26008, #37511, .T. ) ;
#68914=CARTESIAN_POINT ( 'NONE',  ( 46.88368875251780565, 110.3874725885333135, 10.00000000000000000 ) ) ;
#68923=LINE ( 'NONE', #92284, #31330 ) ;
#68924=ADVANCED_FACE ( 'NONE', ( #53705 ), #29924, .F. ) ;
#68929=CARTESIAN_POINT ( 'NONE',  ( -7.338644212303985448, 23.89290704711799052, -10.00000000000000000 ) ) ;
#68932=CARTESIAN_POINT ( 'NONE',  ( 47.22349865033176286, 113.7415181542322955, 177.5919119679930134 ) ) ;
#68933=LINE ( 'NONE', #46636, #69478 ) ;
#68946=VERTEX_POINT ( 'NONE', #39998 ) ;
#68950=EDGE_CURVE ( 'NONE', #32335, #51511, #92225, .T. ) ;
#68953=EDGE_CURVE ( 'NONE', #16754, #95045, #55691, .T. ) ;
#68964=ORIENTED_EDGE ( 'NONE', *, *, #84191, .T. ) ;
#68968=CARTESIAN_POINT ( 'NONE',  ( 46.08672700828314817, 69.01776843458344501, 10.00000000000000000 ) ) ;
#68969=ORIENTED_EDGE ( 'NONE', *, *, #90976, .T. ) ;
#68978=CARTESIAN_POINT ( 'NONE',  ( -19.76768764414644153, 93.14864796480769371, 59.99999999999999289 ) ) ;
#68980=ORIENTED_EDGE ( 'NONE', *, *, #46993, .T. ) ;
#68981=CARTESIAN_POINT ( 'NONE',  ( -17.93832473636817326, 77.02999682207506282, 13.50375772155920195 ) ) ;
#68982=CARTESIAN_POINT ( 'NONE',  ( -62.95439910331221256, 68.06504152958493137, 40.00000000000000000 ) ) ;
#68983=CARTESIAN_POINT ( 'NONE',  ( -19.65312891409030271, 93.06504152958497400, 177.5919119679930134 ) ) ;
#68985=CIRCLE ( 'NONE', #38236, 70.00000000000001421 ) ;
#68986=VERTEX_POINT ( 'NONE', #3543 ) ;
#68987=ORIENTED_EDGE ( 'NONE', *, *, #223, .T. ) ;
#69001=LINE ( 'NONE', #83760, #70768 ) ;
#69008=ORIENTED_EDGE ( 'NONE', *, *, #66494, .T. ) ;
#69015=ADVANCED_FACE ( 'NONE', ( #48636 ), #32913, .F. ) ;
#69021=AXIS2_PLACEMENT_3D ( 'NONE', #45440, #60136, #61136 ) ;
#69029=CARTESIAN_POINT ( 'NONE',  ( 15.77038241084232517, 34.14663330942826036, -10.00000000000000000 ) ) ;
#69034=LINE ( 'NONE', #52838, #28494 ) ;
#69055=VECTOR ( 'NONE', #12438, 999.9999999999998863 ) ;
#69056=EDGE_CURVE ( 'NONE', #36969, #28484, #1579, .T. ) ;
#69058=DIRECTION ( 'NONE',  ( -1.000000000000000000, 0.000000000000000000, 0.000000000000000000 ) ) ;
#69069=ORIENTED_EDGE ( 'NONE', *, *, #24192, .T. ) ;
#69077=EDGE_CURVE ( 'NONE', #68477, #35732, #73926, .T. ) ;
#69079=EDGE_CURVE ( 'NONE', #5333, #89008, #19738, .T. ) ;
#69088=ORIENTED_EDGE ( 'NONE', *, *, #30062, .F. ) ;
#69094=CARTESIAN_POINT ( 'NONE',  ( -42.47074677134370546, 28.21475011077167849, -10.00000000000000000 ) ) ;
#69097=ORIENTED_EDGE ( 'NONE', *, *, #20040, .F. ) ;
#69107=DIRECTION ( 'NONE',  ( -0.6444573283589029034, 0.7646402761589956576, 0.000000000000000000 ) ) ;
#69110=VERTEX_POINT ( 'NONE', #14969 ) ;
#69112=VECTOR ( 'NONE', #70250, 1000.000000000000000 ) ;
#69122=FACE_OUTER_BOUND ( 'NONE', #44088, .T. ) ;
#69123=DIRECTION ( 'NONE',  ( -0.1963739994383812415, 0.9805290675673896672, 0.000000000000000000 ) ) ;
#69134=LINE ( 'NONE', #91481, #88918 ) ;
#69139=DIRECTION ( 'NONE',  ( -0.4140345431502778228, -0.9102611697080902342, 0.000000000000000000 ) ) ;
#69142=CARTESIAN_POINT ( 'NONE',  ( -19.56010499341666886, 93.17209426810804018, 59.99999999999999289 ) ) ;
#69146=ORIENTED_EDGE ( 'NONE', *, *, #44251, .F. ) ;
#69148=CARTESIAN_POINT ( 'NONE',  ( -54.12856498932600147, 45.58573084041748302, 59.99999999999999289 ) ) ;
#69161=CARTESIAN_POINT ( 'NONE',  ( 5.871984111234073822, 29.22396284167520619, -10.00000000000000000 ) ) ;
#69162=AXIS2_PLACEMENT_3D ( 'NONE', #67268, #98194, #21192 ) ;
#69174=ORIENTED_EDGE ( 'NONE', *, *, #81415, .F. ) ;
#69177=EDGE_CURVE ( 'NONE', #1290, #59347, #14288, .T. ) ;
#69188=CARTESIAN_POINT ( 'NONE',  ( 23.64814127513154673, 118.0650415295851019, 45.00000000000000711 ) ) ;
#69194=AXIS2_PLACEMENT_3D ( 'NONE', #60869, #7181, #16287 ) ;
#69198=EDGE_CURVE ( 'NONE', #66499, #49306, #11409, .T. ) ;
#69204=CARTESIAN_POINT ( 'NONE',  ( 30.34687108590969373, 93.06504152958497400, 60.00000000000000000 ) ) ;
#69214=CARTESIAN_POINT ( 'NONE',  ( -76.38857681351474582, 54.22815603855766398, 10.00000000000000000 ) ) ;
#69224=ORIENTED_EDGE ( 'NONE', *, *, #26318, .F. ) ;
#69227=ORIENTED_EDGE ( 'NONE', *, *, #90513, .T. ) ;
#69235=VECTOR ( 'NONE', #82336, 1000.000000000000114 ) ;
#69236=LINE ( 'NONE', #93575, #44650 ) ;
#69253=ORIENTED_EDGE ( 'NONE', *, *, #8988, .F. ) ;
#69254=CARTESIAN_POINT ( 'NONE',  ( 48.73804053012793247, 107.9864336245683631, 177.5919119679930134 ) ) ;
#69255=CIRCLE ( 'NONE', #51472, 70.00000000000001421 ) ;
#69261=AXIS2_PLACEMENT_3D ( 'NONE', #47006, #32303, #16107 ) ;
#69279=FACE_OUTER_BOUND ( 'NONE', #48941, .T. ) ;
#69281=AXIS2_PLACEMENT_3D ( 'NONE', #33342, #94182, #87621 ) ;
#69299=DIRECTION ( 'NONE',  ( -0.8660254037844369313, -0.5000000000000029976, -0.000000000000000000 ) ) ;
#69306=VECTOR ( 'NONE', #55716, 1000.000000000000227 ) ;
#69307=CARTESIAN_POINT ( 'NONE',  ( 44.47956695515382108, 64.36960560548604349, -10.00000000000000000 ) ) ;
#69310=CIRCLE ( 'NONE', #96919, 0.1418229129680863287 ) ;
#69314=CARTESIAN_POINT ( 'NONE',  ( -79.28667360730979397, 56.40661347651924729, -10.00000000000000000 ) ) ;
#69319=VECTOR ( 'NONE', #11814, 1000.000000000000000 ) ;
#69324=VECTOR ( 'NONE', #72522, 1000.000000000000000 ) ;
#69331=ORIENTED_EDGE ( 'NONE', *, *, #13294, .F. ) ;
#69334=DIRECTION ( 'NONE',  ( -1.000000000000000000, 0.000000000000000000, 0.000000000000000000 ) ) ;
#69335=ORIENTED_EDGE ( 'NONE', *, *, #25612, .F. ) ;
#69339=FACE_OUTER_BOUND ( 'NONE', #45350, .T. ) ;
#69345=DIRECTION ( 'NONE',  ( -0.8035972437015875824, -0.5951734788405910193, 0.000000000000000000 ) ) ;
#69346=CARTESIAN_POINT ( 'NONE',  ( -59.87889494062799400, 37.30571521936384016, -10.00000000000000000 ) ) ;
#69347=EDGE_LOOP ( 'NONE', ( #69824, #13692, #82486, #86279, #984, #74239 ) ) ;
#69358=EDGE_CURVE ( 'NONE', #27245, #31851, #20972, .T. ) ;
#69369=ORIENTED_EDGE ( 'NONE', *, *, #4322, .F. ) ;
#69374=DIRECTION ( 'NONE',  ( 0.000000000000000000, -0.000000000000000000, 1.000000000000000000 ) ) ;
#69380=ORIENTED_EDGE ( 'NONE', *, *, #5342, .T. ) ;
#69399=ORIENTED_EDGE ( 'NONE', *, *, #44174, .F. ) ;
#69401=CIRCLE ( 'NONE', #90507, 0.1418229129681522482 ) ;
#69410=EDGE_LOOP ( 'NONE', ( #59936, #20181, #26538, #21016 ) ) ;
#69419=LINE ( 'NONE', #30916, #71179 ) ;
#69423=ORIENTED_EDGE ( 'NONE', *, *, #49069, .F. ) ;
#69437=LINE ( 'NONE', #59324, #59532 ) ;
#69440=CARTESIAN_POINT ( 'NONE',  ( 36.10619739613039769, 52.83927550304669296, -10.00000000000000000 ) ) ;
#69453=FACE_OUTER_BOUND ( 'NONE', #85104, .T. ) ;
#69456=CARTESIAN_POINT ( 'NONE',  ( 30.96785900501025424, 44.34188169337050311, 10.00000000000000000 ) ) ;
#69460=ORIENTED_EDGE ( 'NONE', *, *, #4322, .T. ) ;
#69465=EDGE_LOOP ( 'NONE', ( #97759, #28123, #97077, #84969 ) ) ;
#69469=VERTEX_POINT ( 'NONE', #87345 ) ;
#69478=VECTOR ( 'NONE', #30443, 1000.000000000000114 ) ;
#69480=CARTESIAN_POINT ( 'NONE',  ( -19.65312891409030271, 93.06504152958497400, -10.00000000000000888 ) ) ;
#69481=LINE ( 'NONE', #82749, #54212 ) ;
#69482=VERTEX_POINT ( 'NONE', #80205 ) ;
#69486=FACE_OUTER_BOUND ( 'NONE', #50281, .T. ) ;
#69488=CARTESIAN_POINT ( 'NONE',  ( -61.08640853961129835, 36.64444830801921427, 10.00000000000000000 ) ) ;
#69490=ORIENTED_EDGE ( 'NONE', *, *, #82448, .T. ) ;
#69491=ORIENTED_EDGE ( 'NONE', *, *, #6783, .T. ) ;
#69493=CARTESIAN_POINT ( 'NONE',  ( 47.22349865033175575, 113.7415181542323097, 10.00000000000000000 ) ) ;
#69494=LINE ( 'NONE', #85241, #80126 ) ;
#69501=DIRECTION ( 'NONE',  ( 0.4737039832092511671, 0.8806841296921895657, 0.000000000000000000 ) ) ;
#69502=CARTESIAN_POINT ( 'NONE',  ( 29.59124024723001867, 43.31574901297116043, 10.00000000000000000 ) ) ;
#69506=EDGE_LOOP ( 'NONE', ( #71754, #54500, #724, #92275 ) ) ;
#69517=EDGE_CURVE ( 'NONE', #94399, #18285, #72588, .T. ) ;
#69522=VECTOR ( 'NONE', #7829, 999.9999999999998863 ) ;
#69523=EDGE_CURVE ( 'NONE', #36145, #6477, #17877, .T. ) ;
#69533=ADVANCED_FACE ( 'NONE', ( #3677 ), #56345, .T. ) ;
#69539=DIRECTION ( 'NONE',  ( -0.000000000000000000, 0.000000000000000000, -1.000000000000000000 ) ) ;
#69540=CIRCLE ( 'NONE', #76073, 70.00000000000001421 ) ;
#69553=CARTESIAN_POINT ( 'NONE',  ( 30.34687108590970794, 93.06504152958497400, -40.00000000000000000 ) ) ;
#69569=DIRECTION ( 'NONE',  ( 0.8082118706970062849, 0.5888918169447132644, 0.000000000000000000 ) ) ;
#69574=CARTESIAN_POINT ( 'NONE',  ( 48.74043828842092552, 100.0309547576005258, -10.00000000000000000 ) ) ;
#69576=ORIENTED_EDGE ( 'NONE', *, *, #35071, .T. ) ;
#69581=CARTESIAN_POINT ( 'NONE',  ( 50.06890205215325551, 99.29708757740750968, -10.00000000000000000 ) ) ;
#69584=EDGE_LOOP ( 'NONE', ( #65897, #7655, #46574, #5281 ) ) ;
#69587=DIRECTION ( 'NONE',  ( -0.000000000000000000, -0.000000000000000000, -1.000000000000000000 ) ) ;
#69592=ORIENTED_EDGE ( 'NONE', *, *, #71380, .T. ) ;
#69593=EDGE_CURVE ( 'NONE', #68818, #33333, #79208, .T. ) ;
#69594=CIRCLE ( 'NONE', #72893, 0.1418229129681522482 ) ;
#69607=ORIENTED_EDGE ( 'NONE', *, *, #64890, .F. ) ;
#69610=DIRECTION ( 'NONE',  ( 1.000000000000000000, 0.000000000000000000, 0.000000000000000000 ) ) ;
#69613=ORIENTED_EDGE ( 'NONE', *, *, #82136, .F. ) ;
#69622=CARTESIAN_POINT ( 'NONE',  ( 41.19957572438558913, 58.46810036157969392, 177.5919119679930134 ) ) ;
#69635=CARTESIAN_POINT ( 'NONE',  ( -64.94778771796556782, 41.33875607593970614, -10.00000000000000000 ) ) ;
#69637=EDGE_CURVE ( 'NONE', #15491, #83740, #15218, .T. ) ;
#69649=ORIENTED_EDGE ( 'NONE', *, *, #1428, .F. ) ;
#69650=CARTESIAN_POINT ( 'NONE',  ( -12.95261720355844126, 24.63757726406876714, 10.00000000000000000 ) ) ;
#69654=CARTESIAN_POINT ( 'NONE',  ( -46.74660806181546491, 29.87360136034011049, -10.00000000000000000 ) ) ;
#69667=DIRECTION ( 'NONE',  ( -1.000000000000000000, 0.000000000000000000, 0.000000000000000000 ) ) ;
#69671=DIRECTION ( 'NONE',  ( 0.000000000000000000, 0.000000000000000000, 1.000000000000000000 ) ) ;
#69674=DIRECTION ( 'NONE',  ( -0.5891075386695857619, -0.8080546441192343332, 0.000000000000000000 ) ) ;
#69675=ORIENTED_EDGE ( 'NONE', *, *, #58439, .F. ) ;
#69676=DIRECTION ( 'NONE',  ( -0.000000000000000000, -0.000000000000000000, -1.000000000000000000 ) ) ;
#69684=LINE ( 'NONE', #289, #29053 ) ;
#69689=CARTESIAN_POINT ( 'NONE',  ( -65.13399084342830747, 55.99333101439553673, 59.99999999999999289 ) ) ;
#69691=CARTESIAN_POINT ( 'NONE',  ( 20.94669640352213236, 37.57748520232516398, -10.00000000000000000 ) ) ;
#69701=CARTESIAN_POINT ( 'NONE',  ( -21.74822063352838697, 40.08241122545509683, 59.99999999999999289 ) ) ;
#69702=CARTESIAN_POINT ( 'NONE',  ( 15.67199189347853761, 32.63213790969699346, 177.5919119679930134 ) ) ;
#69710=VERTEX_POINT ( 'NONE', #65336 ) ;
#69719=CARTESIAN_POINT ( 'NONE',  ( -65.10162659358719850, 39.48459004765182812, 10.00000000000000000 ) ) ;
#69720=ADVANCED_FACE ( 'NONE', ( #63834 ), #48651, .F. ) ;
#69721=VERTEX_POINT ( 'NONE', #87217 ) ;
#69726=ORIENTED_EDGE ( 'NONE', *, *, #89366, .T. ) ;
#69728=EDGE_LOOP ( 'NONE', ( #56396, #62208, #13764, #4511 ) ) ;
#69732=CARTESIAN_POINT ( 'NONE',  ( 17.38248943320504836, 35.13769309531819829, 10.00000000000000000 ) ) ;
#69735=LINE ( 'NONE', #31232, #45295 ) ;
#69742=ORIENTED_EDGE ( 'NONE', *, *, #5521, .F. ) ;
#69756=ADVANCED_FACE ( 'NONE', ( #56733 ), #48134, .F. ) ;
#69757=DIRECTION ( 'NONE',  ( 0.000000000000000000, 0.000000000000000000, 1.000000000000000000 ) ) ;
#69758=ORIENTED_EDGE ( 'NONE', *, *, #54391, .T. ) ;
#69772=EDGE_CURVE ( 'NONE', #20413, #16667, #88199, .T. ) ;
#69776=CYLINDRICAL_SURFACE ( 'NONE', #30716, 70.00000000000002842 ) ;
#69787=DIRECTION ( 'NONE',  ( 0.000000000000000000, 0.000000000000000000, 1.000000000000000000 ) ) ;
#69790=CARTESIAN_POINT ( 'NONE',  ( 36.10619739613039769, 52.83927550304669296, 10.00000000000000000 ) ) ;
#69794=CARTESIAN_POINT ( 'NONE',  ( -58.00277386063315532, 34.50477571329874138, -10.00000000000000000 ) ) ;
#69795=EDGE_CURVE ( 'NONE', #26008, #68209, #26843, .T. ) ;
#69797=ADVANCED_FACE ( 'NONE', ( #12144 ), #34922, .F. ) ;
#69803=CARTESIAN_POINT ( 'NONE',  ( 43.53192288983093761, 62.93782412512172186, 177.5919119679930134 ) ) ;
#69819=CARTESIAN_POINT ( 'NONE',  ( -19.65615963453818082, 92.92325100318677755, 59.99999999999999289 ) ) ;
#69822=DIRECTION ( 'NONE',  ( -0.9689885751534038638, -0.2471055264905585858, 0.000000000000000000 ) ) ;
#69824=ORIENTED_EDGE ( 'NONE', *, *, #86864, .T. ) ;
#69828=ORIENTED_EDGE ( 'NONE', *, *, #69358, .T. ) ;
#69829=DIRECTION ( 'NONE',  ( 1.000000000000000000, 0.000000000000000000, 0.000000000000000000 ) ) ;
#69834=VERTEX_POINT ( 'NONE', #81572 ) ;
#69837=LINE ( 'NONE', #23233, #9624 ) ;
#69839=ORIENTED_EDGE ( 'NONE', *, *, #75240, .T. ) ;
#69842=EDGE_CURVE ( 'NONE', #95622, #9585, #96846, .T. ) ;
#69843=VERTEX_POINT ( 'NONE', #54318 ) ;
#69860=EDGE_LOOP ( 'NONE', ( #13952, #25676, #88274, #7308 ) ) ;
#69864=CARTESIAN_POINT ( 'NONE',  ( 32.24342178309110096, 47.97677246190463052, -10.00000000000000000 ) ) ;
#69867=CARTESIAN_POINT ( 'NONE',  ( 11.80767242186427879, 30.53330575246455325, 177.5919119679930134 ) ) ;
#69872=EDGE_LOOP ( 'NONE', ( #54737, #65022, #19061, #54904 ) ) ;
#69873=EDGE_CURVE ( 'NONE', #1725, #70239, #7747, .T. ) ;
#69883=ORIENTED_EDGE ( 'NONE', *, *, #15702, .F. ) ;
#69889=DIRECTION ( 'NONE',  ( 0.7278481391575630788, -0.6857383512134002101, 0.000000000000000000 ) ) ;
#69901=CARTESIAN_POINT ( 'NONE',  ( -19.65312891409030271, 93.06504152958497400, -40.00000000000000000 ) ) ;
#69913=DIRECTION ( 'NONE',  ( 1.000000000000000000, -1.066607120086310925E-13, 0.000000000000000000 ) ) ;
#69943=CARTESIAN_POINT ( 'NONE',  ( -19.65312891409030271, 93.06504152958497400, 177.5919119679930134 ) ) ;
#69957=ORIENTED_EDGE ( 'NONE', *, *, #77543, .F. ) ;
#69962=CARTESIAN_POINT ( 'NONE',  ( 29.13110022456613635, 42.86445400964587549, -10.00000000000000000 ) ) ;
#69970=CARTESIAN_POINT ( 'NONE',  ( -21.58168810074490551, 24.33735145887882112, 10.00000000000000000 ) ) ;
#69975=EDGE_LOOP ( 'NONE', ( #20813, #95982, #60969, #33322 ) ) ;
#69976=CARTESIAN_POINT ( 'NONE',  ( -18.15312891409030982, 78.55673867226647644, 13.76774301257399458 ) ) ;
#69980=VERTEX_POINT ( 'NONE', #47239 ) ;
#69983=CARTESIAN_POINT ( 'NONE',  ( 25.34687108590969729, 93.06504152958497400, 60.00000000000000000 ) ) ;
#69993=CIRCLE ( 'NONE', #40917, 0.1418229129683777623 ) ;
#69995=DIRECTION ( 'NONE',  ( 0.7253665389804488939, 0.6883628288392138472, 0.000000000000000000 ) ) ;
#70000=ORIENTED_EDGE ( 'NONE', *, *, #14542, .F. ) ;
#70009=ORIENTED_EDGE ( 'NONE', *, *, #71141, .F. ) ;
#70014=LINE ( 'NONE', #72042, #51056 ) ;
#70015=AXIS2_PLACEMENT_3D ( 'NONE', #99063, #6350, #84376 ) ;
#70018=LINE ( 'NONE', #32538, #32062 ) ;
#70020=EDGE_CURVE ( 'NONE', #26987, #5926, #85289, .T. ) ;
#70025=DIRECTION ( 'NONE',  ( -1.000000000000000000, 0.000000000000000000, 0.000000000000000000 ) ) ;
#70027=LINE ( 'NONE', #22931, #41797 ) ;
#70029=DIRECTION ( 'NONE',  ( -0.4831861483251571054, -0.8755176446347036068, 0.000000000000000000 ) ) ;
#70033=EDGE_LOOP ( 'NONE', ( #33891, #27005, #97653, #99133 ) ) ;
#70034=EDGE_CURVE ( 'NONE', #66385, #13582, #87185, .T. ) ;
#70039=CARTESIAN_POINT ( 'NONE',  ( -25.71980777823813114, 41.69035350511823879, 59.99999999999999289 ) ) ;
#70040=CYLINDRICAL_SURFACE ( 'NONE', #61025, 60.00000000000002132 ) ;
#70048=EDGE_LOOP ( 'NONE', ( #93537, #10454, #53293, #12075 ) ) ;
#70053=DIRECTION ( 'NONE',  ( 1.000000000000000000, 0.000000000000000000, 0.000000000000000000 ) ) ;
#70054=CARTESIAN_POINT ( 'NONE',  ( -4.170157060006060235, 26.08383846222962887, -10.00000000000000000 ) ) ;
#70067=EDGE_CURVE ( 'NONE', #41966, #95838, #14841, .T. ) ;
#70072=LINE ( 'NONE', #31074, #91421 ) ;
#70083=ORIENTED_EDGE ( 'NONE', *, *, #53495, .F. ) ;
#70087=CIRCLE ( 'NONE', #6966, 0.1418229129680828593 ) ;
#70091=ORIENTED_EDGE ( 'NONE', *, *, #31583, .T. ) ;
#70095=EDGE_LOOP ( 'NONE', ( #79498, #90479, #31398, #44534 ) ) ;
#70100=CARTESIAN_POINT ( 'NONE',  ( -18.45562326176556311, 23.07528527759725634, 177.5919119679930134 ) ) ;
#70101=ORIENTED_EDGE ( 'NONE', *, *, #87641, .T. ) ;
#70108=CARTESIAN_POINT ( 'NONE',  ( -69.61464189717713680, 45.83092310410447112, -10.00000000000000000 ) ) ;
#70115=LINE ( 'NONE', #32632, #44738 ) ;
#70117=DIRECTION ( 'NONE',  ( 0.000000000000000000, 0.000000000000000000, 1.000000000000000000 ) ) ;
#70127=PLANE ( 'NONE',  #23562 ) ;
#70145=VECTOR ( 'NONE', #75206, 1000.000000000000227 ) ;
#70151=VECTOR ( 'NONE', #52353, 1000.000000000000114 ) ;
#70154=DIRECTION ( 'NONE',  ( 0.03277852384265245167, -0.9994626398093610087, 0.000000000000000000 ) ) ;
#70159=EDGE_CURVE ( 'NONE', #38705, #72251, #91262, .T. ) ;
#70168=LINE ( 'NONE', #7895, #36771 ) ;
#70183=ORIENTED_EDGE ( 'NONE', *, *, #72666, .T. ) ;
#70184=CARTESIAN_POINT ( 'NONE',  ( -68.10632939235270555, 44.28490124273476880, -10.00000000000000000 ) ) ;
#70199=DIRECTION ( 'NONE',  ( 0.4535245244745221282, -0.8912437970051507730, 0.000000000000000000 ) ) ;
#70203=EDGE_CURVE ( 'NONE', #55881, #67265, #75075, .T. ) ;
#70208=CARTESIAN_POINT ( 'NONE',  ( -19.65312891409030271, 93.06504152958497400, 59.99999999999999289 ) ) ;
#70213=CARTESIAN_POINT ( 'NONE',  ( -19.65312891409030271, 93.06504152958497400, -10.00000000000000888 ) ) ;
#70214=EDGE_CURVE ( 'NONE', #92543, #54381, #44633, .T. ) ;
#70217=VERTEX_POINT ( 'NONE', #87228 ) ;
#70219=ORIENTED_EDGE ( 'NONE', *, *, #10692, .F. ) ;
#70231=LINE ( 'NONE', #99660, #62437 ) ;
#70239=VERTEX_POINT ( 'NONE', #47137 ) ;
#70240=CARTESIAN_POINT ( 'NONE',  ( 29.12701137275935181, 44.61184105132205957, -10.00000000000000000 ) ) ;
#70244=DIRECTION ( 'NONE',  ( -0.000000000000000000, 0.000000000000000000, -1.000000000000000000 ) ) ;
#70250=DIRECTION ( 'NONE',  ( 0.000000000000000000, 0.000000000000000000, 1.000000000000000000 ) ) ;
#70255=DIRECTION ( 'NONE',  ( -0.000000000000000000, -0.000000000000000000, -1.000000000000000000 ) ) ;
#70263=ORIENTED_EDGE ( 'NONE', *, *, #4583, .T. ) ;
#70278=DIRECTION ( 'NONE',  ( -0.9756173257765569096, -0.2194785493951510180, 0.000000000000000000 ) ) ;
#70284=DIRECTION ( 'NONE',  ( -0.000000000000000000, -0.000000000000000000, -1.000000000000000000 ) ) ;
#70287=EDGE_CURVE ( 'NONE', #4641, #72984, #94783, .T. ) ;
#70292=DIRECTION ( 'NONE',  ( 0.000000000000000000, 0.000000000000000000, 1.000000000000000000 ) ) ;
#70293=EDGE_CURVE ( 'NONE', #44322, #21282, #23836, .T. ) ;
#70302=CARTESIAN_POINT ( 'NONE',  ( 4.781100836665275189, 70.53751509772452266, -10.00000000000000000 ) ) ;
#70318=ADVANCED_FACE ( 'NONE', ( #1568 ), #31933, .F. ) ;
#70323=VERTEX_POINT ( 'NONE', #63844 ) ;
#70327=ORIENTED_EDGE ( 'NONE', *, *, #90949, .F. ) ;
#70331=CARTESIAN_POINT ( 'NONE',  ( -19.65009819364242105, 93.20683205598336940, 59.99999999999999289 ) ) ;
#70332=EDGE_CURVE ( 'NONE', #25048, #17411, #71963, .T. ) ;
#70336=EDGE_LOOP ( 'NONE', ( #71110, #61916, #90252, #51131 ) ) ;
#70338=DIRECTION ( 'NONE',  ( -0.5951734788405910193, 0.8035972437015875824, 0.000000000000000000 ) ) ;
#70342=ORIENTED_EDGE ( 'NONE', *, *, #40586, .F. ) ;
#70343=LINE ( 'NONE', #61736, #88710 ) ;
#70367=DIRECTION ( 'NONE',  ( -0.000000000000000000, -0.000000000000000000, -1.000000000000000000 ) ) ;
#70373=ORIENTED_EDGE ( 'NONE', *, *, #13487, .T. ) ;
#70374=VECTOR ( 'NONE', #43425, 1000.000000000000114 ) ;
#70376=DIRECTION ( 'NONE',  ( 0.7059494278973771353, -0.7082622432767159415, 0.000000000000000000 ) ) ;
#70379=ORIENTED_EDGE ( 'NONE', *, *, #26204, .T. ) ;
#70382=VECTOR ( 'NONE', #78615, 1000.000000000000000 ) ;
#70390=CARTESIAN_POINT ( 'NONE',  ( 40.48539884740146277, 126.3902902409112556, -10.00000000000000000 ) ) ;
#70394=VERTEX_POINT ( 'NONE', #79596 ) ;
#70401=ORIENTED_EDGE ( 'NONE', *, *, #85332, .T. ) ;
#70407=DIRECTION ( 'NONE',  ( 1.000000000000000000, 0.000000000000000000, 0.000000000000000000 ) ) ;
#70411=ADVANCED_FACE ( 'NONE', ( #48145 ), #77565, .F. ) ;
#70418=DIRECTION ( 'NONE',  ( -0.9404163354663408469, -0.3400251696390412803, 0.000000000000000000 ) ) ;
#70425=DIRECTION ( 'NONE',  ( 1.000000000000000000, 0.000000000000000000, 0.000000000000000000 ) ) ;
#70427=LINE ( 'NONE', #62307, #97678 ) ;
#70434=VECTOR ( 'NONE', #9540, 1000.000000000000114 ) ;
#70440=CARTESIAN_POINT ( 'NONE',  ( 48.77433535142598231, 99.76555324011610537, 10.00000000000000000 ) ) ;
#70443=CARTESIAN_POINT ( 'NONE',  ( 44.85937643310611378, 116.8208962945185050, -10.00000000000000000 ) ) ;
#70446=DIRECTION ( 'NONE',  ( 0.8261602328994307465, -0.5634352399127678934, 0.000000000000000000 ) ) ;
#70453=ORIENTED_EDGE ( 'NONE', *, *, #57987, .T. ) ;
#70462=EDGE_LOOP ( 'NONE', ( #56664, #51560, #34114, #85610 ) ) ;
#70473=ADVANCED_FACE ( 'NONE', ( #56743 ), #12154, .F. ) ;
#70474=LINE ( 'NONE', #9707, #93287 ) ;
#70475=VECTOR ( 'NONE', #58543, 1000.000000000000114 ) ;
#70479=ORIENTED_EDGE ( 'NONE', *, *, #99162, .F. ) ;
#70484=ORIENTED_EDGE ( 'NONE', *, *, #51003, .T. ) ;
#70487=VECTOR ( 'NONE', #60390, 1000.000000000000000 ) ;
#70489=ORIENTED_EDGE ( 'NONE', *, *, #62571, .F. ) ;
#70496=DIRECTION ( 'NONE',  ( 0.6600842437418872333, -0.7511915808658273797, 0.000000000000000000 ) ) ;
#70498=CARTESIAN_POINT ( 'NONE',  ( 31.12960416526798824, 44.88710030135629836, -10.00000000000000000 ) ) ;
#70499=CARTESIAN_POINT ( 'NONE',  ( -48.92208041226317050, 108.8082784536894110, -10.00000000000000000 ) ) ;
#70503=CARTESIAN_POINT ( 'NONE',  ( 38.67262647093125594, 99.46401760883253473, 59.99999999999999289 ) ) ;
#70511=CIRCLE ( 'NONE', #26845, 70.00000000000001421 ) ;
#70523=FACE_OUTER_BOUND ( 'NONE', #35206, .T. ) ;
#70526=ORIENTED_EDGE ( 'NONE', *, *, #34499, .T. ) ;
#70527=LINE ( 'NONE', #1144, #39788 ) ;
#70528=CARTESIAN_POINT ( 'NONE',  ( 50.00170217996129907, 86.12209509027381671, 10.00000000000000000 ) ) ;
#70532=LINE ( 'NONE', #7742, #100039 ) ;
#70534=EDGE_CURVE ( 'NONE', #65714, #76666, #42041, .T. ) ;
#70539=EDGE_CURVE ( 'NONE', #62627, #74024, #99252, .T. ) ;
#70546=CARTESIAN_POINT ( 'NONE',  ( 47.66616421796179992, 112.2513067263565034, 177.5919119679930134 ) ) ;
#70548=FACE_OUTER_BOUND ( 'NONE', #69728, .T. ) ;
#70573=CIRCLE ( 'NONE', #73850, 70.00000000000001421 ) ;
#70582=ORIENTED_EDGE ( 'NONE', *, *, #98914, .F. ) ;
#70584=VERTEX_POINT ( 'NONE', #92189 ) ;
#70587=ORIENTED_EDGE ( 'NONE', *, *, #23073, .T. ) ;
#70588=CARTESIAN_POINT ( 'NONE',  ( 32.51871346713573274, 102.5332718713895588, 59.99999999999999289 ) ) ;
#70603=ORIENTED_EDGE ( 'NONE', *, *, #23962, .T. ) ;
#70604=ORIENTED_EDGE ( 'NONE', *, *, #7079, .T. ) ;
#70607=ORIENTED_EDGE ( 'NONE', *, *, #32862, .T. ) ;
#70616=CARTESIAN_POINT ( 'NONE',  ( 47.78135487164287554, 106.4364430393875267, -10.00000000000000000 ) ) ;
#70617=EDGE_LOOP ( 'NONE', ( #79013, #4778, #45045, #76248 ) ) ;
#70627=DIRECTION ( 'NONE',  ( -0.9184028970038772277, -0.3956464567955659817, 0.000000000000000000 ) ) ;
#70630=AXIS2_PLACEMENT_3D ( 'NONE', #92951, #54916, #7832 ) ;
#70634=ORIENTED_EDGE ( 'NONE', *, *, #65564, .T. ) ;
#70636=DIRECTION ( 'NONE',  ( -1.000000000000000000, 0.000000000000000000, 0.000000000000000000 ) ) ;
#70646=VERTEX_POINT ( 'NONE', #82597 ) ;
#70649=CARTESIAN_POINT ( 'NONE',  ( -58.62427208439002158, 70.56504152958493137, 60.00000000000000000 ) ) ;
#70651=EDGE_CURVE ( 'NONE', #8402, #61894, #29348, .T. ) ;
#70660=ORIENTED_EDGE ( 'NONE', *, *, #51004, .T. ) ;
#70662=ADVANCED_FACE ( 'NONE', ( #90184 ), #74958, .T. ) ;
#70676=VERTEX_POINT ( 'NONE', #46010 ) ;
#70688=DIRECTION ( 'NONE',  ( 1.000000000000000000, 0.000000000000000000, 0.000000000000000000 ) ) ;
#70689=VECTOR ( 'NONE', #79001, 1000.000000000000227 ) ;
#70693=ORIENTED_EDGE ( 'NONE', *, *, #80791, .T. ) ;
#70696=AXIS2_PLACEMENT_3D ( 'NONE', #23742, #50541, #12066 ) ;
#70698=ORIENTED_EDGE ( 'NONE', *, *, #42609, .T. ) ;
#70702=DIRECTION ( 'NONE',  ( -0.8560416229147732592, -0.5169068966820244970, 0.000000000000000000 ) ) ;
#70705=AXIS2_PLACEMENT_3D ( 'NONE', #55667, #24301, #63292 ) ;
#70710=ORIENTED_EDGE ( 'NONE', *, *, #27580, .F. ) ;
#70719=CARTESIAN_POINT ( 'NONE',  ( -52.57320609282758994, 32.70376883311633520, -10.00000000000000000 ) ) ;
#70722=AXIS2_PLACEMENT_3D ( 'NONE', #36841, #60123, #75875 ) ;
#70726=VERTEX_POINT ( 'NONE', #45521 ) ;
#70728=ORIENTED_EDGE ( 'NONE', *, *, #47722, .F. ) ;
#70737=CARTESIAN_POINT ( 'NONE',  ( -10.80656490723494123, 24.88181024604956804, 10.00000000000000000 ) ) ;
#70760=ORIENTED_EDGE ( 'NONE', *, *, #46855, .T. ) ;
#70763=ORIENTED_EDGE ( 'NONE', *, *, #59425, .F. ) ;
#70764=CARTESIAN_POINT ( 'NONE',  ( -19.65312891409030271, 93.06504152958497400, -10.00000000000000888 ) ) ;
#70768=VECTOR ( 'NONE', #99433, 1000.000000000000114 ) ;
#70791=DIRECTION ( 'NONE',  ( 0.1162373735601320568, 0.9932214622066130039, 0.000000000000000000 ) ) ;
#70805=EDGE_CURVE ( 'NONE', #20627, #11925, #99750, .T. ) ;
#70809=CARTESIAN_POINT ( 'NONE',  ( 32.30839531297598910, 123.0650415295850593, -25.00000000000000000 ) ) ;
#70812=VECTOR ( 'NONE', #83422, 1000.000000000000114 ) ;
#70814=PLANE ( 'NONE',  #74141 ) ;
#70832=DIRECTION ( 'NONE',  ( -0.9974094913373522386, -0.07193265315671491800, 0.000000000000000000 ) ) ;
#70834=ORIENTED_EDGE ( 'NONE', *, *, #99971, .T. ) ;
#70836=VECTOR ( 'NONE', #40761, 1000.000000000000114 ) ;
#70843=DIRECTION ( 'NONE',  ( -0.1654779384134575648, 0.9862134920484671996, 0.000000000000000000 ) ) ;
#70844=ORIENTED_EDGE ( 'NONE', *, *, #29406, .F. ) ;
#70845=LINE ( 'NONE', #85599, #74960 ) ;
#70847=DIRECTION ( 'NONE',  ( -0.5344452582589588330, 0.8452030915256492083, 0.000000000000000000 ) ) ;
#70848=VECTOR ( 'NONE', #15078, 1000.000000000000000 ) ;
#70849=VERTEX_POINT ( 'NONE', #1943 ) ;
#70857=ORIENTED_EDGE ( 'NONE', *, *, #96425, .T. ) ;
#70859=DIRECTION ( 'NONE',  ( 0.3002896333693371722, 0.9538480676139722281, 0.000000000000000000 ) ) ;
#70872=VECTOR ( 'NONE', #9290, 1000.000000000000000 ) ;
#70875=VERTEX_POINT ( 'NONE', #438 ) ;
#70890=EDGE_CURVE ( 'NONE', #99040, #47742, #15940, .T. ) ;
#70892=ORIENTED_EDGE ( 'NONE', *, *, #67438, .F. ) ;
#70893=VERTEX_POINT ( 'NONE', #88101 ) ;
#70894=LINE ( 'NONE', #63279, #39897 ) ;
#70898=DIRECTION ( 'NONE',  ( -0.8660254037844369313, -0.5000000000000029976, -0.000000000000000000 ) ) ;
#70901=VERTEX_POINT ( 'NONE', #72867 ) ;
#70921=EDGE_CURVE ( 'NONE', #45184, #58863, #88599, .T. ) ;
#70935=VECTOR ( 'NONE', #97516, 1000.000000000000114 ) ;
#70938=VERTEX_POINT ( 'NONE', #59979 ) ;
#70950=DIRECTION ( 'NONE',  ( 0.000000000000000000, 0.000000000000000000, 1.000000000000000000 ) ) ;
#70965=CARTESIAN_POINT ( 'NONE',  ( 45.88188149789386472, 72.29567966924399514, 10.00000000000000000 ) ) ;
#70966=DIRECTION ( 'NONE',  ( -0.9957145386939475484, -0.09248003802712848054, 0.000000000000000000 ) ) ;
#70967=VERTEX_POINT ( 'NONE', #33863 ) ;
#70969=CYLINDRICAL_SURFACE ( 'NONE', #63585, 70.00000000000002842 ) ;
#70975=VECTOR ( 'NONE', #34289, 1000.000000000000000 ) ;
#70977=ORIENTED_EDGE ( 'NONE', *, *, #11405, .T. ) ;
#70987=ORIENTED_EDGE ( 'NONE', *, *, #5083, .F. ) ;
#70993=AXIS2_PLACEMENT_3D ( 'NONE', #52795, #31000, #29517 ) ;
#70994=DIRECTION ( 'NONE',  ( 0.8755176446346986108, -0.4831861483251663203, 0.000000000000000000 ) ) ;
#70996=DIRECTION ( 'NONE',  ( 0.000000000000000000, 0.000000000000000000, 1.000000000000000000 ) ) ;
#70999=EDGE_CURVE ( 'NONE', #65627, #33084, #9527, .T. ) ;
#71017=AXIS2_PLACEMENT_3D ( 'NONE', #94812, #54246, #40055 ) ;
#71021=FACE_OUTER_BOUND ( 'NONE', #66868, .T. ) ;
#71022=EDGE_LOOP ( 'NONE', ( #82995, #47784, #4859, #58721, #65020, #4319 ) ) ;
#71034=ORIENTED_EDGE ( 'NONE', *, *, #98607, .F. ) ;
#71041=EDGE_LOOP ( 'NONE', ( #29608, #84322, #75851, #79756 ) ) ;
#71060=DIRECTION ( 'NONE',  ( 1.000000000000000000, -1.070572202317114942E-14, 0.000000000000000000 ) ) ;
#71072=CARTESIAN_POINT ( 'NONE',  ( -19.52403302344049507, 93.00632194460597191, 59.99999999999999289 ) ) ;
#71073=CARTESIAN_POINT ( 'NONE',  ( 42.25626477193290498, 60.39660150822810891, 177.5919119679930134 ) ) ;
#71091=EDGE_CURVE ( 'NONE', #50887, #11410, #7793, .T. ) ;
#71109=DIRECTION ( 'NONE',  ( -0.5000000000000012212, 0.8660254037844378194, -0.000000000000000000 ) ) ;
#71110=ORIENTED_EDGE ( 'NONE', *, *, #12345, .F. ) ;
#71113=ORIENTED_EDGE ( 'NONE', *, *, #96152, .T. ) ;
#71114=DIRECTION ( 'NONE',  ( 0.4803199113995043623, -0.8770933717188679202, 0.000000000000000000 ) ) ;
#71115=LINE ( 'NONE', #87385, #66160 ) ;
#71116=ORIENTED_EDGE ( 'NONE', *, *, #67438, .T. ) ;
#71119=LINE ( 'NONE', #10813, #90149 ) ;
#71123=DIRECTION ( 'NONE',  ( 1.000000000000000000, 0.000000000000000000, 0.000000000000000000 ) ) ;
#71129=ORIENTED_EDGE ( 'NONE', *, *, #75925, .T. ) ;
#71130=ADVANCED_FACE ( 'NONE', ( #53385, #31076 ), #23470, .F. ) ;
#71131=ORIENTED_EDGE ( 'NONE', *, *, #85646, .T. ) ;
#71133=EDGE_LOOP ( 'NONE', ( #67725, #66495, #76001, #24362 ) ) ;
#71135=CARTESIAN_POINT ( 'NONE',  ( 19.39999966495784989, 36.48715600906563594, -10.00000000000000000 ) ) ;
#71138=EDGE_CURVE ( 'NONE', #75897, #42311, #9814, .T. ) ;
#71141=EDGE_CURVE ( 'NONE', #99910, #6796, #26007, .T. ) ;
#71147=DIRECTION ( 'NONE',  ( -0.7280311630581435267, -0.6855440362341479466, 0.000000000000000000 ) ) ;
#71151=AXIS2_PLACEMENT_3D ( 'NONE', #99082, #29664, #60541 ) ;
#71152=CARTESIAN_POINT ( 'NONE',  ( -19.65312891409030271, 93.06504152958497400, 10.00000000000000888 ) ) ;
#71153=VERTEX_POINT ( 'NONE', #8789 ) ;
#71160=VECTOR ( 'NONE', #98715, 1000.000000000000114 ) ;
#71161=ORIENTED_EDGE ( 'NONE', *, *, #10728, .F. ) ;
#71163=CYLINDRICAL_SURFACE ( 'NONE', #3122, 70.00000000000002842 ) ;
#71166=DIRECTION ( 'NONE',  ( -0.9606745773021557744, 0.2776767122488390527, 0.000000000000000000 ) ) ;
#71170=FACE_OUTER_BOUND ( 'NONE', #72014, .T. ) ;
#71171=FACE_OUTER_BOUND ( 'NONE', #13085, .T. ) ;
#71173=CARTESIAN_POINT ( 'NONE',  ( -44.49648453423614569, 28.96346851210257967, 10.00000000000000000 ) ) ;
#71174=VECTOR ( 'NONE', #18283, 1000.000000000000000 ) ;
#71176=ORIENTED_EDGE ( 'NONE', *, *, #42942, .T. ) ;
#71179=VECTOR ( 'NONE', #32420, 1000.000000000000000 ) ;
#71182=CARTESIAN_POINT ( 'NONE',  ( -19.51454890667437425, 93.09519646595313702, 59.99999999999999289 ) ) ;
#71208=VECTOR ( 'NONE', #25527, 1000.000000000000000 ) ;
#71210=CARTESIAN_POINT ( 'NONE',  ( 9.242171499132833645, 29.30720582267293750, 10.00000000000000000 ) ) ;
#71222=ORIENTED_EDGE ( 'NONE', *, *, #28134, .F. ) ;
#71225=CARTESIAN_POINT ( 'NONE',  ( -19.65312891409030271, 93.06504152958497400, -10.00000000000000888 ) ) ;
#71229=VERTEX_POINT ( 'NONE', #99828 ) ;
#71230=DIRECTION ( 'NONE',  ( -0.6363689690731114679, -0.7713848165480219343, 0.000000000000000000 ) ) ;
#71236=DIRECTION ( 'NONE',  ( 0.5864613938488598688, -0.8099771808667527440, 0.000000000000000000 ) ) ;
#71250=ORIENTED_EDGE ( 'NONE', *, *, #6598, .T. ) ;
#71253=DIRECTION ( 'NONE',  ( 0.5102188382608533468, -0.8600446134263879383, 0.000000000000000000 ) ) ;
#71257=DIRECTION ( 'NONE',  ( -1.000000000000000000, 0.000000000000000000, 0.000000000000000000 ) ) ;
#71261=DIRECTION ( 'NONE',  ( -0.000000000000000000, 0.000000000000000000, 1.000000000000000000 ) ) ;
#71264=VERTEX_POINT ( 'NONE', #46092 ) ;
#71269=ORIENTED_EDGE ( 'NONE', *, *, #92088, .T. ) ;
#71279=LINE ( 'NONE', #9470, #90206 ) ;
#71283=VERTEX_POINT ( 'NONE', #30911 ) ;
#71296=CYLINDRICAL_SURFACE ( 'NONE', #18321, 70.00000000000002842 ) ;
#71300=CARTESIAN_POINT ( 'NONE',  ( 50.37091257173480585, 98.81520120758277415, -10.00000000000000000 ) ) ;
#71301=VECTOR ( 'NONE', #20082, 1000.000000000000114 ) ;
#71307=LINE ( 'NONE', #55565, #70975 ) ;
#71308=CARTESIAN_POINT ( 'NONE',  ( 49.07419501245632176, 91.40403951869188859, -10.00000000000000000 ) ) ;
#71310=ADVANCED_FACE ( 'NONE', ( #8123 ), #93758, .F. ) ;
#71314=CYLINDRICAL_SURFACE ( 'NONE', #93314, 49.99999999999999289 ) ;
#71318=DIRECTION ( 'NONE',  ( -0.000000000000000000, -0.000000000000000000, -1.000000000000000000 ) ) ;
#71320=EDGE_CURVE ( 'NONE', #93866, #179, #37991, .T. ) ;
#71337=CARTESIAN_POINT ( 'NONE',  ( 28.50765780192512366, 60.84557485627980356, 59.99999999999999289 ) ) ;
#71340=CARTESIAN_POINT ( 'NONE',  ( -16.99542894172669349, 24.36904009834038476, -10.00000000000000000 ) ) ;
#71346=EDGE_LOOP ( 'NONE', ( #99181, #93258, #99650, #51337 ) ) ;
#71359=EDGE_LOOP ( 'NONE', ( #14636, #7682, #9740, #48663 ) ) ;
#71364=EDGE_CURVE ( 'NONE', #46853, #29881, #43981, .T. ) ;
#71366=ORIENTED_EDGE ( 'NONE', *, *, #96297, .T. ) ;
#71367=FACE_OUTER_BOUND ( 'NONE', #49918, .T. ) ;
#71370=VECTOR ( 'NONE', #14771, 1000.000000000000000 ) ;
#71380=EDGE_CURVE ( 'NONE', #47254, #28615, #51601, .T. ) ;
#71382=DIRECTION ( 'NONE',  ( -0.1889875038809470109, -0.9819794923402672682, 0.000000000000000000 ) ) ;
#71386=DIRECTION ( 'NONE',  ( -0.9042435392811277728, -0.4270171210482544000, 0.000000000000000000 ) ) ;
#71388=ORIENTED_EDGE ( 'NONE', *, *, #58430, .T. ) ;
#71392=CARTESIAN_POINT ( 'NONE',  ( -19.65312891409030271, 93.06504152958497400, 177.5919119679930134 ) ) ;
#71399=ORIENTED_EDGE ( 'NONE', *, *, #70287, .T. ) ;
#71402=ORIENTED_EDGE ( 'NONE', *, *, #14495, .T. ) ;
#71413=DIRECTION ( 'NONE',  ( -0.8806841296921844586, 0.4737039832092607705, 0.000000000000000000 ) ) ;
#71415=EDGE_LOOP ( 'NONE', ( #82253, #78175, #7693, #58611 ) ) ;
#71434=CARTESIAN_POINT ( 'NONE',  ( 36.76746430747500938, 51.63176190406337440, -10.00000000000000000 ) ) ;
#71441=ADVANCED_FACE ( 'NONE', ( #25188 ), #9511, .F. ) ;
#71461=CARTESIAN_POINT ( 'NONE',  ( -19.65312891409030271, 93.06504152958497400, 177.5919119679930134 ) ) ;
#71465=CARTESIAN_POINT ( 'NONE',  ( -5.008551768858394482, 80.94865873146321178, 13.45811050236818396 ) ) ;
#71477=VERTEX_POINT ( 'NONE', #17087 ) ;
#71486=DIRECTION ( 'NONE',  ( -0.000000000000000000, -0.000000000000000000, -1.000000000000000000 ) ) ;
#71489=ORIENTED_EDGE ( 'NONE', *, *, #81177, .F. ) ;
#71493=VERTEX_POINT ( 'NONE', #95143 ) ;
#71499=ADVANCED_FACE ( 'NONE', ( #11018 ), #34295, .F. ) ;
#71506=ORIENTED_EDGE ( 'NONE', *, *, #38757, .F. ) ;
#71509=LINE ( 'NONE', #63885, #11569 ) ;
#71520=DIRECTION ( 'NONE',  ( 0.3984034379158949979, -0.9172102815913020235, 0.000000000000000000 ) ) ;
#71522=ORIENTED_EDGE ( 'NONE', *, *, #92720, .F. ) ;
#71526=DIRECTION ( 'NONE',  ( 0.000000000000000000, 0.000000000000000000, 1.000000000000000000 ) ) ;
#71536=DIRECTION ( 'NONE',  ( -0.000000000000000000, -0.000000000000000000, -1.000000000000000000 ) ) ;
#71541=EDGE_LOOP ( 'NONE', ( #18581, #52895, #95635, #16666 ) ) ;
#71549=PLANE ( 'NONE',  #41760 ) ;
#71564=EDGE_LOOP ( 'NONE', ( #74884, #92240, #43302, #51811 ) ) ;
#71565=EDGE_CURVE ( 'NONE', #41961, #20907, #16592, .T. ) ;
#71589=DIRECTION ( 'NONE',  ( 0.000000000000000000, 0.000000000000000000, 1.000000000000000000 ) ) ;
#71598=CARTESIAN_POINT ( 'NONE',  ( 48.92549481379852949, 97.87922363803308201, -10.00000000000000000 ) ) ;
#71605=DIRECTION ( 'NONE',  ( 0.000000000000000000, 0.000000000000000000, 1.000000000000000000 ) ) ;
#71606=ORIENTED_EDGE ( 'NONE', *, *, #65687, .F. ) ;
#71612=CARTESIAN_POINT ( 'NONE',  ( -3.153128914090298274, 64.48620320469859735, 0.000000000000000000 ) ) ;
#71613=ORIENTED_EDGE ( 'NONE', *, *, #14542, .T. ) ;
#71618=VERTEX_POINT ( 'NONE', #7368 ) ;
#71622=CARTESIAN_POINT ( 'NONE',  ( 45.88188149789386472, 72.29567966924399514, -10.00000000000000000 ) ) ;
#71633=EDGE_CURVE ( 'NONE', #82108, #15950, #67684, .T. ) ;
#71634=DIRECTION ( 'NONE',  ( 0.000000000000000000, 0.000000000000000000, 1.000000000000000000 ) ) ;
#71637=ORIENTED_EDGE ( 'NONE', *, *, #61017, .T. ) ;
#71638=ORIENTED_EDGE ( 'NONE', *, *, #17605, .F. ) ;
#71640=ORIENTED_EDGE ( 'NONE', *, *, #34946, .T. ) ;
#71651=CIRCLE ( 'NONE', #18264, 0.1418229129681487788 ) ;
#71653=CARTESIAN_POINT ( 'NONE',  ( -19.52673012263424113, 93.12936169874843984, 59.99999999999999289 ) ) ;
#71660=ORIENTED_EDGE ( 'NONE', *, *, #42865, .T. ) ;
#71665=CARTESIAN_POINT ( 'NONE',  ( -68.10632939235270555, 44.28490124273479012, -10.00000000000000000 ) ) ;
#71667=LINE ( 'NONE', #39212, #85519 ) ;
#71672=EDGE_CURVE ( 'NONE', #80413, #10181, #91027, .T. ) ;
#71682=EDGE_LOOP ( 'NONE', ( #34377, #37949, #94361, #77267 ) ) ;
#71694=EDGE_CURVE ( 'NONE', #68946, #31611, #23553, .T. ) ;
#71698=AXIS2_PLACEMENT_3D ( 'NONE', #33833, #49020, #26714 ) ;
#71700=DIRECTION ( 'NONE',  ( -1.000000000000000000, 0.000000000000000000, 0.000000000000000000 ) ) ;
#71705=DIRECTION ( 'NONE',  ( 1.000000000000000000, 0.000000000000000000, 0.000000000000000000 ) ) ;
#71707=ADVANCED_FACE ( 'NONE', ( #60557 ), #52474, .T. ) ;
#71710=ORIENTED_EDGE ( 'NONE', *, *, #33570, .T. ) ;
#71711=EDGE_CURVE ( 'NONE', #90103, #83863, #32211, .T. ) ;
#71712=DIRECTION ( 'NONE',  ( 0.8660254037844379305, 0.5000000000000011102, 0.000000000000000000 ) ) ;
#71715=DIRECTION ( 'NONE',  ( -1.000000000000000000, 0.000000000000000000, 0.000000000000000000 ) ) ;
#71717=VECTOR ( 'NONE', #42400, 1000.000000000000227 ) ;
#71725=ORIENTED_EDGE ( 'NONE', *, *, #36985, .F. ) ;
#71726=LINE ( 'NONE', #49400, #84584 ) ;
#71731=DIRECTION ( 'NONE',  ( 0.000000000000000000, 0.000000000000000000, 1.000000000000000000 ) ) ;
#71738=EDGE_LOOP ( 'NONE', ( #29759, #7097, #3254, #69380 ) ) ;
#71744=DIRECTION ( 'NONE',  ( -0.9086904199442051855, 0.4174706225611858335, 0.000000000000000000 ) ) ;
#71754=ORIENTED_EDGE ( 'NONE', *, *, #26528, .T. ) ;
#71762=PLANE ( 'NONE',  #35345 ) ;
#71764=DIRECTION ( 'NONE',  ( -0.000000000000000000, 0.000000000000000000, -1.000000000000000000 ) ) ;
#71771=VECTOR ( 'NONE', #44395, 1000.000000000000114 ) ;
#71786=CARTESIAN_POINT ( 'NONE',  ( -59.87889494062799400, 37.30571521936384016, -10.00000000000000000 ) ) ;
#71787=VECTOR ( 'NONE', #94937, 1000.000000000000000 ) ;
#71795=EDGE_LOOP ( 'NONE', ( #46547, #97999, #63511, #22924 ) ) ;
#71797=PRODUCT_DEFINITION_SHAPE ( 'NONE', 'NONE',  #80580 ) ;
#71824=EDGE_CURVE ( 'NONE', #4560, #65492, #2804, .T. ) ;
#71833=DIRECTION ( 'NONE',  ( 0.000000000000000000, 0.000000000000000000, 1.000000000000000000 ) ) ;
#71834=FACE_OUTER_BOUND ( 'NONE', #47403, .T. ) ;
#71837=FACE_OUTER_BOUND ( 'NONE', #72410, .T. ) ;
#71845=CARTESIAN_POINT ( 'NONE',  ( 50.32263495959776378, 94.90690751109829648, 177.5919119679930134 ) ) ;
#71847=DIRECTION ( 'NONE',  ( -0.8434505012732950169, 0.5372068985985076761, 0.000000000000000000 ) ) ;
#71856=CARTESIAN_POINT ( 'NONE',  ( -19.79442730923454263, 93.05285538284211100, 59.99999999999999289 ) ) ;
#71858=ORIENTED_EDGE ( 'NONE', *, *, #19912, .F. ) ;
#71860=VECTOR ( 'NONE', #84466, 1000.000000000000000 ) ;
#71861=ORIENTED_EDGE ( 'NONE', *, *, #79595, .T. ) ;
#71865=VERTEX_POINT ( 'NONE', #54963 ) ;
#71872=VERTEX_POINT ( 'NONE', #78287 ) ;
#71879=CARTESIAN_POINT ( 'NONE',  ( 47.54560441532652959, 78.55524412553474178, 10.00000000000000000 ) ) ;
#71884=ORIENTED_EDGE ( 'NONE', *, *, #30739, .F. ) ;
#71891=ORIENTED_EDGE ( 'NONE', *, *, #18384, .T. ) ;
#71898=ORIENTED_EDGE ( 'NONE', *, *, #37497, .F. ) ;
#71914=AXIS2_PLACEMENT_3D ( 'NONE', #72556, #19357, #27436 ) ;
#71915=DIRECTION ( 'NONE',  ( 0.000000000000000000, -0.000000000000000000, 1.000000000000000000 ) ) ;
#71916=VERTEX_POINT ( 'NONE', #9895 ) ;
#71923=DIRECTION ( 'NONE',  ( 0.9985437513708439461, 0.05394790633789421641, 0.000000000000000000 ) ) ;
#71925=AXIS2_PLACEMENT_3D ( 'NONE', #58397, #89372, #97432 ) ;
#71930=DIRECTION ( 'NONE',  ( -0.000000000000000000, -0.000000000000000000, -1.000000000000000000 ) ) ;
#71950=DIRECTION ( 'NONE',  ( -1.000000000000000000, 0.000000000000000000, 0.000000000000000000 ) ) ;
#71954=DIRECTION ( 'NONE',  ( -0.1580495287025983631, -0.9874311856918873698, 0.000000000000000000 ) ) ;
#71957=DIRECTION ( 'NONE',  ( -0.000000000000000000, -0.000000000000000000, 1.000000000000000000 ) ) ;
#71960=ORIENTED_EDGE ( 'NONE', *, *, #5199, .T. ) ;
#71961=CARTESIAN_POINT ( 'NONE',  ( -15.89092471255436401, 83.83718066579119466, 14.94482985791953489 ) ) ;
#71963=LINE ( 'NONE', #62327, #61197 ) ;
#71968=CARTESIAN_POINT ( 'NONE',  ( -19.79289719785049328, 93.08909491806775804, 59.99999999999999289 ) ) ;
#71973=ORIENTED_EDGE ( 'NONE', *, *, #94328, .F. ) ;
#71978=LINE ( 'NONE', #25359, #36868 ) ;
#71984=ORIENTED_EDGE ( 'NONE', *, *, #27472, .T. ) ;
#71993=VECTOR ( 'NONE', #77927, 1000.000000000000000 ) ;
#71997=VERTEX_POINT ( 'NONE', #73191 ) ;
#72003=ADVANCED_FACE ( 'NONE', ( #73682 ), #67056, .F. ) ;
#72008=DIRECTION ( 'NONE',  ( 0.02225111142181396620, 0.9997524133706775507, 0.000000000000000000 ) ) ;
#72013=CARTESIAN_POINT ( 'NONE',  ( 46.54103524584391494, 115.8319611975524595, 177.5919119679930134 ) ) ;
#72014=EDGE_LOOP ( 'NONE', ( #47581, #92671, #43077, #3238 ) ) ;
#72022=VECTOR ( 'NONE', #91163, 1000.000000000000227 ) ;
#72031=CARTESIAN_POINT ( 'NONE',  ( -79.43448886220070904, 56.15136215343108717, -10.00000000000000000 ) ) ;
#72032=EDGE_CURVE ( 'NONE', #54142, #62846, #97021, .T. ) ;
#72040=LINE ( 'NONE', #10236, #73505 ) ;
#72042=CARTESIAN_POINT ( 'NONE',  ( -74.97640825042664403, 52.25402898078436920, -10.00000000000000000 ) ) ;
#72043=CARTESIAN_POINT ( 'NONE',  ( 24.79662394327660024, 66.59991831601136880, 59.99999999999999289 ) ) ;
#72051=LINE ( 'NONE', #2654, #49908 ) ;
#72054=LINE ( 'NONE', #33548, #83893 ) ;
#72059=ORIENTED_EDGE ( 'NONE', *, *, #95683, .F. ) ;
#72062=CARTESIAN_POINT ( 'NONE',  ( -15.10528209597770299, 24.46087392797020499, -10.00000000000000000 ) ) ;
#72071=EDGE_CURVE ( 'NONE', #43154, #100075, #35164, .T. ) ;
#72072=DIRECTION ( 'NONE',  ( 0.2803049773603249473, -0.9599109957006575211, 0.000000000000000000 ) ) ;
#72085=CARTESIAN_POINT ( 'NONE',  ( -61.68394390806074057, 53.17837850769589636, 59.99999999999999289 ) ) ;
#72091=DIRECTION ( 'NONE',  ( 0.000000000000000000, -0.000000000000000000, 1.000000000000000000 ) ) ;
#72106=CIRCLE ( 'NONE', #54265, 70.00000000000001421 ) ;
#72111=VERTEX_POINT ( 'NONE', #96023 ) ;
#72113=ORIENTED_EDGE ( 'NONE', *, *, #5138, .F. ) ;
#72117=DIRECTION ( 'NONE',  ( -0.9994626398093606756, -0.03277852384266338737, 0.000000000000000000 ) ) ;
#72124=CARTESIAN_POINT ( 'NONE',  ( 16.05454730341465464, 46.50537555954188917, 59.99999999999999289 ) ) ;
#72125=DIRECTION ( 'NONE',  ( 1.000000000000000000, 0.000000000000000000, 0.000000000000000000 ) ) ;
#72129=ORIENTED_EDGE ( 'NONE', *, *, #76964, .T. ) ;
#72130=ORIENTED_EDGE ( 'NONE', *, *, #45812, .T. ) ;
#72132=AXIS2_PLACEMENT_3D ( 'NONE', #17717, #11624, #49599 ) ;
#72135=ORIENTED_EDGE ( 'NONE', *, *, #92872, .F. ) ;
#72142=EDGE_CURVE ( 'NONE', #61085, #65492, #80835, .T. ) ;
#72145=EDGE_LOOP ( 'NONE', ( #4597, #63633, #47116, #29649 ) ) ;
#72146=CARTESIAN_POINT ( 'NONE',  ( -50.19188543474569997, 43.82156839606978593, 59.99999999999999289 ) ) ;
#72150=DIRECTION ( 'NONE',  ( 1.000000000000000000, 0.000000000000000000, 0.000000000000000000 ) ) ;
#72152=ORIENTED_EDGE ( 'NONE', *, *, #73646, .T. ) ;
#72158=CYLINDRICAL_SURFACE ( 'NONE', #53804, 6.749999999999988454 ) ;
#72161=DIRECTION ( 'NONE',  ( 0.000000000000000000, -0.000000000000000000, 1.000000000000000000 ) ) ;
#72173=VECTOR ( 'NONE', #15050, 1000.000000000000114 ) ;
#72174=DIRECTION ( 'NONE',  ( -0.9682419296822714072, -0.2500151307524236532, 0.000000000000000000 ) ) ;
#72197=VECTOR ( 'NONE', #53578, 1000.000000000000000 ) ;
#72200=ADVANCED_FACE ( 'NONE', ( #93390 ), #8752, .F. ) ;
#72206=CIRCLE ( 'NONE', #34923, 70.00000000000001421 ) ;
#72220=LINE ( 'NONE', #64606, #33788 ) ;
#72222=EDGE_LOOP ( 'NONE', ( #84982, #49909, #90740, #9572 ) ) ;
#72231=VERTEX_POINT ( 'NONE', #85298 ) ;
#72236=ORIENTED_EDGE ( 'NONE', *, *, #56572, .F. ) ;
#72245=CIRCLE ( 'NONE', #90046, 70.00000000000001421 ) ;
#72246=DIRECTION ( 'NONE',  ( -0.7909930170786232395, 0.6118251767726273771, 0.000000000000000000 ) ) ;
#72250=DIRECTION ( 'NONE',  ( 1.000000000000000000, 3.241454723682375892E-13, 0.000000000000000000 ) ) ;
#72251=VERTEX_POINT ( 'NONE', #15841 ) ;
#72257=VERTEX_POINT ( 'NONE', #79200 ) ;
#72260=ORIENTED_EDGE ( 'NONE', *, *, #40470, .F. ) ;
#72268=EDGE_CURVE ( 'NONE', #32592, #96097, #39623, .T. ) ;
#72275=VECTOR ( 'NONE', #28769, 1000.000000000000114 ) ;
#72284=VECTOR ( 'NONE', #86689, 1000.000000000000114 ) ;
#72286=EDGE_CURVE ( 'NONE', #77851, #38792, #93792, .T. ) ;
#72287=CYLINDRICAL_SURFACE ( 'NONE', #30481, 70.00000000000002842 ) ;
#72303=CARTESIAN_POINT ( 'NONE',  ( 2.552633344394289239, 68.33802890835346489, -10.00000000000000000 ) ) ;
#72315=CARTESIAN_POINT ( 'NONE',  ( -19.66365018104914242, 92.92360942013182523, 59.99999999999999289 ) ) ;
#72316=VECTOR ( 'NONE', #10709, 1000.000000000000227 ) ;
#72325=DIRECTION ( 'NONE',  ( 0.000000000000000000, 0.000000000000000000, 1.000000000000000000 ) ) ;
#72338=CARTESIAN_POINT ( 'NONE',  ( 24.55112987542764458, 40.41347472807389352, -10.00000000000000000 ) ) ;
#72349=VECTOR ( 'NONE', #87539, 1000.000000000000000 ) ;
#72353=AXIS2_PLACEMENT_3D ( 'NONE', #70208, #30227, #15504 ) ;
#72354=DIRECTION ( 'NONE',  ( -0.9954322480537355355, -0.09547062131716983757, 0.000000000000000000 ) ) ;
#72363=DIRECTION ( 'NONE',  ( -0.9963824715083249295, 0.08498217737244645464, 0.000000000000000000 ) ) ;
#72364=EDGE_CURVE ( 'NONE', #45522, #66829, #51755, .T. ) ;
#72365=DIRECTION ( 'NONE',  ( -0.000000000000000000, -0.000000000000000000, 1.000000000000000000 ) ) ;
#72366=ORIENTED_EDGE ( 'NONE', *, *, #88355, .F. ) ;
#72372=ORIENTED_EDGE ( 'NONE', *, *, #99840, .F. ) ;
#72384=DIRECTION ( 'NONE',  ( -0.9291732088853876803, 0.3696446237802353818, 0.000000000000000000 ) ) ;
#72388=DIRECTION ( 'NONE',  ( -0.8769651246872924855, 0.4805540241036398985, 0.000000000000000000 ) ) ;
#72391=ORIENTED_EDGE ( 'NONE', *, *, #83883, .F. ) ;
#72392=LINE ( 'NONE', #26274, #56076 ) ;
#72396=VECTOR ( 'NONE', #21721, 1000.000000000000114 ) ;
#72401=CYLINDRICAL_SURFACE ( 'NONE', #46595, 70.00000000000002842 ) ;
#72407=ADVANCED_FACE ( 'NONE', ( #5637 ), #13263, .F. ) ;
#72408=CIRCLE ( 'NONE', #67523, 70.00000000000001421 ) ;
#72410=EDGE_LOOP ( 'NONE', ( #7577, #8227, #66869, #14702 ) ) ;
#72412=EDGE_CURVE ( 'NONE', #37985, #17180, #90552, .T. ) ;
#72427=CARTESIAN_POINT ( 'NONE',  ( -19.65312891409030271, 93.06504152958497400, 177.5919119679930134 ) ) ;
#72428=DIRECTION ( 'NONE',  ( -0.9994626398093606756, -0.03277852384266338737, 0.000000000000000000 ) ) ;
#72429=EDGE_LOOP ( 'NONE', ( #54253, #26245, #16661, #77998 ) ) ;
#72443=DIRECTION ( 'NONE',  ( 1.000000000000000000, 5.352861011585574712E-15, 0.000000000000000000 ) ) ;
#72451=CIRCLE ( 'NONE', #41907, 50.00000000000000711 ) ;
#72455=LINE ( 'NONE', #3547, #40382 ) ;
#72458=EDGE_CURVE ( 'NONE', #20973, #24937, #77924, .T. ) ;
#72471=CARTESIAN_POINT ( 'NONE',  ( 2.064617007569734319, 27.83817977871672511, 10.00000000000000000 ) ) ;
#72472=CARTESIAN_POINT ( 'NONE',  ( -78.57153713424663977, 57.64153020465174393, 10.00000000000000000 ) ) ;
#72477=CARTESIAN_POINT ( 'NONE',  ( -11.87431992379006296, 23.49859753039504895, -10.00000000000000000 ) ) ;
#72480=VERTEX_POINT ( 'NONE', #91272 ) ;
#72491=AXIS2_PLACEMENT_3D ( 'NONE', #16671, #31858, #47565 ) ;
#72496=DIRECTION ( 'NONE',  ( 0.000000000000000000, 0.000000000000000000, 1.000000000000000000 ) ) ;
#72499=CARTESIAN_POINT ( 'NONE',  ( -19.76587483483573138, 92.97900609503616920, 59.99999999999999289 ) ) ;
#72502=LINE ( 'NONE', #3108, #52361 ) ;
#72515=ORIENTED_EDGE ( 'NONE', *, *, #82372, .T. ) ;
#72522=DIRECTION ( 'NONE',  ( -0.000000000000000000, 0.000000000000000000, -1.000000000000000000 ) ) ;
#72528=ORIENTED_EDGE ( 'NONE', *, *, #21544, .F. ) ;
#72535=VECTOR ( 'NONE', #85754, 1000.000000000000114 ) ;
#72539=CARTESIAN_POINT ( 'NONE',  ( 49.09806598349715046, 107.5461990276917845, 10.00000000000000000 ) ) ;
#72543=ORIENTED_EDGE ( 'NONE', *, *, #59510, .F. ) ;
#72556=CARTESIAN_POINT ( 'NONE',  ( -19.65312891409030271, 93.06504152958497400, 10.00000000000000888 ) ) ;
#72558=CIRCLE ( 'NONE', #48228, 70.00000000000001421 ) ;
#72559=DIRECTION ( 'NONE',  ( -0.7352104281592295454, 0.6778389383370672094, 0.000000000000000000 ) ) ;
#72560=LINE ( 'NONE', #3163, #87116 ) ;
#72568=DIRECTION ( 'NONE',  ( -1.000000000000000000, 0.000000000000000000, 0.000000000000000000 ) ) ;
#72569=AXIS2_PLACEMENT_3D ( 'NONE', #23229, #85076, #77459 ) ;
#72572=VERTEX_POINT ( 'NONE', #88077 ) ;
#72576=EDGE_CURVE ( 'NONE', #91263, #3024, #79457, .T. ) ;
#72588=LINE ( 'NONE', #73566, #1353 ) ;
#72594=VECTOR ( 'NONE', #22900, 1000.000000000000000 ) ;
#72601=CARTESIAN_POINT ( 'NONE',  ( -42.47074677134370546, 28.21475011077167849, 10.00000000000000000 ) ) ;
#72604=DIRECTION ( 'NONE',  ( -0.9922852870422774751, 0.1239754375649672058, 0.000000000000000000 ) ) ;
#72605=LINE ( 'NONE', #41661, #191 ) ;
#72613=CARTESIAN_POINT ( 'NONE',  ( 45.29894525614688661, 66.96469553601603764, 10.00000000000000000 ) ) ;
#72619=DIRECTION ( 'NONE',  ( -1.000000000000000000, 0.000000000000000000, 0.000000000000000000 ) ) ;
#72621=VECTOR ( 'NONE', #87523, 1000.000000000000114 ) ;
#72622=ORIENTED_EDGE ( 'NONE', *, *, #11100, .F. ) ;
#72632=CIRCLE ( 'NONE', #95288, 70.00000000000001421 ) ;
#72634=VERTEX_POINT ( 'NONE', #19136 ) ;
#72639=ORIENTED_EDGE ( 'NONE', *, *, #71138, .F. ) ;
#72640=EDGE_CURVE ( 'NONE', #40956, #44226, #50009, .T. ) ;
#72644=ORIENTED_EDGE ( 'NONE', *, *, #14955, .T. ) ;
#72647=ORIENTED_EDGE ( 'NONE', *, *, #94473, .F. ) ;
#72649=EDGE_LOOP ( 'NONE', ( #39812, #100135, #25490, #96985 ) ) ;
#72655=LINE ( 'NONE', #42696, #71208 ) ;
#72659=ORIENTED_EDGE ( 'NONE', *, *, #51159, .F. ) ;
#72660=CARTESIAN_POINT ( 'NONE',  ( -9.693023484072631035, 23.77726266618848072, 10.00000000000000000 ) ) ;
#72666=EDGE_CURVE ( 'NONE', #100031, #43051, #72754, .T. ) ;
#72669=EDGE_CURVE ( 'NONE', #85106, #55654, #41395, .T. ) ;
#72677=AXIS2_PLACEMENT_3D ( 'NONE', #53317, #75641, #6734 ) ;
#72694=PLANE ( 'NONE',  #46632 ) ;
#72698=DIRECTION ( 'NONE',  ( 1.000000000000000000, 0.000000000000000000, 0.000000000000000000 ) ) ;
#72702=EDGE_LOOP ( 'NONE', ( #69742, #31013, #56123, #56673 ) ) ;
#72707=EDGE_CURVE ( 'NONE', #66378, #46791, #64720, .T. ) ;
#72718=VERTEX_POINT ( 'NONE', #34309 ) ;
#72720=LINE ( 'NONE', #35678, #57887 ) ;
#72727=CARTESIAN_POINT ( 'NONE',  ( 49.87168060777529632, 103.2007005253944385, 10.00000000000000000 ) ) ;
#72729=ORIENTED_EDGE ( 'NONE', *, *, #83127, .T. ) ;
#72735=ORIENTED_EDGE ( 'NONE', *, *, #55087, .F. ) ;
#72736=DIRECTION ( 'NONE',  ( -0.5803476755362181327, -0.8143688203140567738, 0.000000000000000000 ) ) ;
#72743=PLANE ( 'NONE',  #10555 ) ;
#72754=CIRCLE ( 'NONE', #74331, 0.1418229129681522482 ) ;
#72762=VERTEX_POINT ( 'NONE', #85440 ) ;
#72763=EDGE_CURVE ( 'NONE', #29268, #45532, #14979, .T. ) ;
#72764=VERTEX_POINT ( 'NONE', #14001 ) ;
#72779=CARTESIAN_POINT ( 'NONE',  ( 50.12332653952446293, 98.65487733484056321, 177.5919119679930134 ) ) ;
#72786=ADVANCED_FACE ( 'NONE', ( #30190 ), #99114, .F. ) ;
#72790=EDGE_CURVE ( 'NONE', #44698, #48849, #69684, .T. ) ;
#72795=DIRECTION ( 'NONE',  ( -0.9879014915521906470, 0.1550826972584532504, 0.000000000000000000 ) ) ;
#72800=ORIENTED_EDGE ( 'NONE', *, *, #56572, .T. ) ;
#72801=DIRECTION ( 'NONE',  ( 1.000000000000000000, 0.000000000000000000, 0.000000000000000000 ) ) ;
#72811=CARTESIAN_POINT ( 'NONE',  ( -19.65312891409030271, 93.06504152958497400, -45.00000000000001421 ) ) ;
#72824=VECTOR ( 'NONE', #25781, 1000.000000000000227 ) ;
#72830=FACE_OUTER_BOUND ( 'NONE', #3951, .T. ) ;
#72833=DIRECTION ( 'NONE',  ( 0.000000000000000000, 0.000000000000000000, 1.000000000000000000 ) ) ;
#72834=CARTESIAN_POINT ( 'NONE',  ( -20.65464553008483151, 23.07220643578490993, 177.5919119679930134 ) ) ;
#72838=CARTESIAN_POINT ( 'NONE',  ( -78.71521058394758086, 57.86724000996476747, -10.00000000000000000 ) ) ;
#72839=EDGE_CURVE ( 'NONE', #5980, #14868, #41977, .T. ) ;
#72842=DIRECTION ( 'NONE',  ( 0.8816062427480149122, 0.4719856276919119353, 0.000000000000000000 ) ) ;
#72853=EDGE_CURVE ( 'NONE', #8078, #65825, #25599, .T. ) ;
#72854=ADVANCED_FACE ( 'NONE', ( #55466 ), #95035, .F. ) ;
#72861=DIRECTION ( 'NONE',  ( 1.000000000000000000, 0.000000000000000000, 0.000000000000000000 ) ) ;
#72867=CARTESIAN_POINT ( 'NONE',  ( -72.39633208959961053, 47.04162880533178992, 10.00000000000000000 ) ) ;
#72873=CARTESIAN_POINT ( 'NONE',  ( -19.65312891409030271, 93.06504152958497400, 59.99999999999999289 ) ) ;
#72875=VERTEX_POINT ( 'NONE', #71210 ) ;
#72893=AXIS2_PLACEMENT_3D ( 'NONE', #14759, #83708, #29466 ) ;
#72895=CARTESIAN_POINT ( 'NONE',  ( -2.330697855141256269, 26.52822386297705393, -10.00000000000000000 ) ) ;
#72898=EDGE_LOOP ( 'NONE', ( #3454, #12041, #29356, #66726 ) ) ;
#72899=LINE ( 'NONE', #11585, #75498 ) ;
#72901=ORIENTED_EDGE ( 'NONE', *, *, #5083, .T. ) ;
#72931=DIRECTION ( 'NONE',  ( -1.000000000000000000, 0.000000000000000000, 0.000000000000000000 ) ) ;
#72950=CARTESIAN_POINT ( 'NONE',  ( -28.04097607764120781, 24.82386083235215679, -10.00000000000000000 ) ) ;
#72951=VERTEX_POINT ( 'NONE', #27604 ) ;
#72955=LINE ( 'NONE', #18239, #56596 ) ;
#72963=LINE ( 'NONE', #49143, #67050 ) ;
#72968=VECTOR ( 'NONE', #51962, 1000.000000000000000 ) ;
#72973=CARTESIAN_POINT ( 'NONE',  ( -18.15312891409030982, 79.21382371532438071, 13.90677182048132998 ) ) ;
#72976=VERTEX_POINT ( 'NONE', #74713 ) ;
#72978=DIRECTION ( 'NONE',  ( 0.9041295198386993803, -0.4272584830711297910, 0.000000000000000000 ) ) ;
#72984=VERTEX_POINT ( 'NONE', #97035 ) ;
#72992=DIRECTION ( 'NONE',  ( -0.000000000000000000, -0.000000000000000000, -1.000000000000000000 ) ) ;
#72993=DIRECTION ( 'NONE',  ( -0.000000000000000000, 0.000000000000000000, 1.000000000000000000 ) ) ;
#72995=ORIENTED_EDGE ( 'NONE', *, *, #64630, .F. ) ;
#73005=EDGE_CURVE ( 'NONE', #93038, #25226, #81826, .T. ) ;
#73010=VERTEX_POINT ( 'NONE', #43267 ) ;
#73012=FACE_BOUND ( 'NONE', #50998, .T. ) ;
#73021=CARTESIAN_POINT ( 'NONE',  ( -46.74660806181546491, 29.87360136034011049, 10.00000000000000000 ) ) ;
#73029=ADVANCED_FACE ( 'NONE', ( #74213 ), #4803, .F. ) ;
#73048=CARTESIAN_POINT ( 'NONE',  ( -74.97640825042664403, 52.25402898078436920, -10.00000000000000000 ) ) ;
#73080=EDGE_CURVE ( 'NONE', #85089, #12428, #5290, .T. ) ;
#73103=PLANE ( 'NONE',  #42446 ) ;
#73111=DIRECTION ( 'NONE',  ( -0.9946578707245746775, -0.1032265479692855564, 0.000000000000000000 ) ) ;
#73113=AXIS2_PLACEMENT_3D ( 'NONE', #28454, #19405, #50756 ) ;
#73117=LINE ( 'NONE', #39786, #76846 ) ;
#73120=CARTESIAN_POINT ( 'NONE',  ( 46.50192534792603283, 74.36443251879779837, -10.00000000000000000 ) ) ;
#73130=DIRECTION ( 'NONE',  ( -0.000000000000000000, -0.000000000000000000, -1.000000000000000000 ) ) ;
#73131=EDGE_LOOP ( 'NONE', ( #5819, #73225, #48879, #94504 ) ) ;
#73134=EDGE_LOOP ( 'NONE', ( #55425, #76754, #68745, #18258 ) ) ;
#73136=ORIENTED_EDGE ( 'NONE', *, *, #90616, .F. ) ;
#73147=CARTESIAN_POINT ( 'NONE',  ( 38.52196584993465223, 56.41980893122115504, 10.00000000000000000 ) ) ;
#73149=ADVANCED_FACE ( 'NONE', ( #30072 ), #54345, .F. ) ;
#73152=LINE ( 'NONE', #88396, #56352 ) ;
#73154=ORIENTED_EDGE ( 'NONE', *, *, #88798, .F. ) ;
#73155=ORIENTED_EDGE ( 'NONE', *, *, #45758, .F. ) ;
#73158=CARTESIAN_POINT ( 'NONE',  ( 23.64814127513160358, 118.0650415295850166, 25.00000000000000000 ) ) ;
#73163=ORIENTED_EDGE ( 'NONE', *, *, #93807, .T. ) ;
#73172=LINE ( 'NONE', #34644, #13021 ) ;
#73191=CARTESIAN_POINT ( 'NONE',  ( -7.471379830813591916, 36.41558964265287557, 59.99999999999999289 ) ) ;
#73212=CARTESIAN_POINT ( 'NONE',  ( 45.19716250472275476, 70.24742367233086782, 10.00000000000000000 ) ) ;
#73217=VECTOR ( 'NONE', #51899, 1000.000000000000000 ) ;
#73225=ORIENTED_EDGE ( 'NONE', *, *, #70921, .F. ) ;
#73229=VERTEX_POINT ( 'NONE', #47753 ) ;
#73231=LINE ( 'NONE', #5317, #87266 ) ;
#73233=EDGE_LOOP ( 'NONE', ( #67221, #25210, #34505, #93832 ) ) ;
#73241=ORIENTED_EDGE ( 'NONE', *, *, #71633, .T. ) ;
#73242=ORIENTED_EDGE ( 'NONE', *, *, #19237, .T. ) ;
#73244=ORIENTED_EDGE ( 'NONE', *, *, #17691, .F. ) ;
#73249=ORIENTED_EDGE ( 'NONE', *, *, #27472, .F. ) ;
#73255=LINE ( 'NONE', #88506, #29122 ) ;
#73260=VERTEX_POINT ( 'NONE', #49280 ) ;
#73264=CARTESIAN_POINT ( 'NONE',  ( -19.65312891409030271, 93.06504152958497400, -10.00000000000000888 ) ) ;
#73266=ADVANCED_FACE ( 'NONE', ( #2691 ), #95438, .F. ) ;
#73277=ORIENTED_EDGE ( 'NONE', *, *, #52765, .F. ) ;
#73278=CARTESIAN_POINT ( 'NONE',  ( -39.52511050156712002, 25.94496742513405962, 177.5919119679930134 ) ) ;
#73281=CARTESIAN_POINT ( 'NONE',  ( -72.92390943388483038, 47.25396573843040926, 10.00000000000000000 ) ) ;
#73282=DIRECTION ( 'NONE',  ( -0.000000000000000000, 0.000000000000000000, -1.000000000000000000 ) ) ;
#73284=AXIS2_PLACEMENT_3D ( 'NONE', #71461, #9144, #68569 ) ;
#73293=CARTESIAN_POINT ( 'NONE',  ( -76.38857681351474582, 54.22815603855766398, -10.00000000000000000 ) ) ;
#73294=ADVANCED_FACE ( 'NONE', ( #95071 ), #87505, .F. ) ;
#73295=CARTESIAN_POINT ( 'NONE',  ( -35.82302091652844922, 24.69132351629776423, -10.00000000000000000 ) ) ;
#73297=CARTESIAN_POINT ( 'NONE',  ( 49.03918259513507394, 79.59780946358316100, 10.00000000000000000 ) ) ;
#73305=VECTOR ( 'NONE', #60088, 1000.000000000000000 ) ;
#73306=DIRECTION ( 'NONE',  ( 0.06415622980647768536, -0.9979398670145503969, 0.000000000000000000 ) ) ;
#73317=EDGE_CURVE ( 'NONE', #24915, #3476, #51413, .T. ) ;
#73323=CARTESIAN_POINT ( 'NONE',  ( 4.102725850843912170, 28.55253618238880620, -10.00000000000000000 ) ) ;
#73337=EDGE_CURVE ( 'NONE', #72572, #16478, #84117, .T. ) ;
#73348=VERTEX_POINT ( 'NONE', #16402 ) ;
#73353=FACE_OUTER_BOUND ( 'NONE', #74740, .T. ) ;
#73355=CARTESIAN_POINT ( 'NONE',  ( -19.65312891409030271, 93.06504152958497400, -10.00000000000000888 ) ) ;
#73361=DIRECTION ( 'NONE',  ( -0.000000000000000000, -0.000000000000000000, -1.000000000000000000 ) ) ;
#73368=FACE_OUTER_BOUND ( 'NONE', #31363, .T. ) ;
#73370=LINE ( 'NONE', #88123, #86895 ) ;
#73374=VECTOR ( 'NONE', #31541, 1000.000000000000000 ) ;
#73378=DIRECTION ( 'NONE',  ( -0.09573633691163400961, -0.9954067278227238802, 0.000000000000000000 ) ) ;
#73382=ORIENTED_EDGE ( 'NONE', *, *, #186, .F. ) ;
#73389=ORIENTED_EDGE ( 'NONE', *, *, #49308, .F. ) ;
#73391=CARTESIAN_POINT ( 'NONE',  ( 48.95103868752454446, 97.61288834769685252, -10.00000000000000000 ) ) ;
#73402=ORIENTED_EDGE ( 'NONE', *, *, #70805, .F. ) ;
#73407=LINE ( 'NONE', #48606, #88566 ) ;
#73408=CARTESIAN_POINT ( 'NONE',  ( -37.40701240123934213, 25.35389310390295137, -10.00000000000000000 ) ) ;
#73409=EDGE_CURVE ( 'NONE', #19773, #179, #81248, .T. ) ;
#73425=CARTESIAN_POINT ( 'NONE',  ( -19.65312891409030271, 93.06504152958497400, -10.00000000000000888 ) ) ;
#73428=AXIS2_PLACEMENT_3D ( 'NONE', #43037, #58744, #89717 ) ;
#73431=VECTOR ( 'NONE', #59694, 1000.000000000000000 ) ;
#73450=EDGE_CURVE ( 'NONE', #55017, #6693, #24265, .T. ) ;
#73454=PLANE ( 'NONE',  #32049 ) ;
#73455=EDGE_LOOP ( 'NONE', ( #98766, #67113, #10160, #40192 ) ) ;
#73457=VERTEX_POINT ( 'NONE', #95212 ) ;
#73473=DIRECTION ( 'NONE',  ( -1.000000000000000000, 0.000000000000000000, 0.000000000000000000 ) ) ;
#73475=CARTESIAN_POINT ( 'NONE',  ( 15.11407551230992041, 32.30945333909092909, 177.5919119679930134 ) ) ;
#73478=VERTEX_POINT ( 'NONE', #23745 ) ;
#73479=ORIENTED_EDGE ( 'NONE', *, *, #19412, .F. ) ;
#73482=CARTESIAN_POINT ( 'NONE',  ( 30.68386671255119325, 44.42157463747831514, 10.00000000000000000 ) ) ;
#73483=ORIENTED_EDGE ( 'NONE', *, *, #32635, .F. ) ;
#73485=CARTESIAN_POINT ( 'NONE',  ( 13.90223112049948639, 33.06302660730329279, -10.00000000000000000 ) ) ;
#73488=EDGE_CURVE ( 'NONE', #49704, #43692, #63260, .T. ) ;
#73495=ORIENTED_EDGE ( 'NONE', *, *, #88252, .F. ) ;
#73504=ORIENTED_EDGE ( 'NONE', *, *, #53760, .T. ) ;
#73505=VECTOR ( 'NONE', #8726, 1000.000000000000000 ) ;
#73506=DIRECTION ( 'NONE',  ( -0.7909930170786166892, 0.6118251767726361479, 0.000000000000000000 ) ) ;
#73518=CARTESIAN_POINT ( 'NONE',  ( -63.60198981653986294, 65.77656800267020287, 59.99999999999999289 ) ) ;
#73522=ORIENTED_EDGE ( 'NONE', *, *, #50727, .T. ) ;
#73524=DIRECTION ( 'NONE',  ( -0.3105719460338643989, -0.9505498757754579087, 0.000000000000000000 ) ) ;
#73530=DIRECTION ( 'NONE',  ( -0.000000000000000000, -0.000000000000000000, -1.000000000000000000 ) ) ;
#73531=EDGE_LOOP ( 'NONE', ( #85591, #29987, #28565, #61251 ) ) ;
#73534=LINE ( 'NONE', #96867, #25218 ) ;
#73543=DIRECTION ( 'NONE',  ( 0.3400251696390308997, -0.9404163354663445107, 0.000000000000000000 ) ) ;
#73545=CARTESIAN_POINT ( 'NONE',  ( -55.24278990345137430, 55.52121124131609520, 59.99999999999999289 ) ) ;
#73546=CARTESIAN_POINT ( 'NONE',  ( -65.04438592786723916, 55.88340059208193367, 59.99999999999999289 ) ) ;
#73547=EDGE_CURVE ( 'NONE', #95263, #70646, #27268, .T. ) ;
#73557=PLANE ( 'NONE',  #46454 ) ;
#73566=CARTESIAN_POINT ( 'NONE',  ( -21.31413092498266693, 24.33771760303832465, -10.00000000000000000 ) ) ;
#73577=AXIS2_PLACEMENT_3D ( 'NONE', #82760, #89852, #14306 ) ;
#73583=ADVANCED_FACE ( 'NONE', ( #96700 ), #58636, .F. ) ;
#73591=CARTESIAN_POINT ( 'NONE',  ( -4.653128914090328472, 78.77562236714182120, 13.81405534229504717 ) ) ;
#73593=ORIENTED_EDGE ( 'NONE', *, *, #68385, .F. ) ;
#73598=ORIENTED_EDGE ( 'NONE', *, *, #89652, .F. ) ;
#73603=VERTEX_POINT ( 'NONE', #35353 ) ;
#73604=DIRECTION ( 'NONE',  ( 0.000000000000000000, 0.000000000000000000, 1.000000000000000000 ) ) ;
#73607=CARTESIAN_POINT ( 'NONE',  ( -19.15453390681661716, 24.31945705462846163, 10.00000000000000000 ) ) ;
#73615=ORIENTED_EDGE ( 'NONE', *, *, #73695, .T. ) ;
#73622=ORIENTED_EDGE ( 'NONE', *, *, #65240, .F. ) ;
#73638=ORIENTED_EDGE ( 'NONE', *, *, #31697, .T. ) ;
#73640=CARTESIAN_POINT ( 'NONE',  ( -71.45866285464214229, 45.60329508610311677, 10.00000000000000000 ) ) ;
#73646=EDGE_CURVE ( 'NONE', #91333, #39135, #4971, .T. ) ;
#73663=LINE ( 'NONE', #2780, #44595 ) ;
#73666=DIRECTION ( 'NONE',  ( -0.8393827800519415572, -0.5435407515102007592, 0.000000000000000000 ) ) ;
#73676=ORIENTED_EDGE ( 'NONE', *, *, #81736, .F. ) ;
#73678=VECTOR ( 'NONE', #81152, 1000.000000000000000 ) ;
#73682=FACE_OUTER_BOUND ( 'NONE', #18298, .T. ) ;
#73684=CARTESIAN_POINT ( 'NONE',  ( -57.88150100324660485, 35.92665207732902388, 10.00000000000000000 ) ) ;
#73688=VERTEX_POINT ( 'NONE', #63138 ) ;
#73690=CYLINDRICAL_SURFACE ( 'NONE', #51453, 70.00000000000002842 ) ;
#73695=EDGE_CURVE ( 'NONE', #89109, #76961, #32238, .T. ) ;
#73712=AXIS2_PLACEMENT_3D ( 'NONE', #62284, #96750, #19236 ) ;
#73731=CARTESIAN_POINT ( 'NONE',  ( 41.82599275875796252, 62.29945068332010294, -10.00000000000000000 ) ) ;
#73736=ORIENTED_EDGE ( 'NONE', *, *, #27275, .F. ) ;
#73745=PLANE ( 'NONE',  #20396 ) ;
#73747=CARTESIAN_POINT ( 'NONE',  ( -19.60707684373364046, 93.19917931493495189, 59.99999999999999289 ) ) ;
#73754=VECTOR ( 'NONE', #60264, 1000.000000000000000 ) ;
#73755=PLANE ( 'NONE',  #89914 ) ;
#73758=DIRECTION ( 'NONE',  ( 0.9874311856918874808, -0.1580495287025984186, 0.000000000000000000 ) ) ;
#73759=EDGE_CURVE ( 'NONE', #49794, #8436, #27536, .T. ) ;
#73771=ORIENTED_EDGE ( 'NONE', *, *, #720, .F. ) ;
#73774=EDGE_CURVE ( 'NONE', #77218, #78854, #46942, .T. ) ;
#73776=DIRECTION ( 'NONE',  ( -1.000000000000000000, 0.000000000000000000, 0.000000000000000000 ) ) ;
#73782=ORIENTED_EDGE ( 'NONE', *, *, #16681, .T. ) ;
#73787=VECTOR ( 'NONE', #9884, 1000.000000000000227 ) ;
#73790=FACE_OUTER_BOUND ( 'NONE', #77488, .T. ) ;
#73793=LINE ( 'NONE', #98605, #66116 ) ;
#73795=CARTESIAN_POINT ( 'NONE',  ( -19.65312891409030271, 93.06504152958497400, 10.00000000000000888 ) ) ;
#73799=DIRECTION ( 'NONE',  ( -0.2473641778533918756, -0.9689225787001330970, 0.000000000000000000 ) ) ;
#73813=CIRCLE ( 'NONE', #75487, 70.00000000000001421 ) ;
#73814=ADVANCED_FACE ( 'NONE', ( #24637 ), #23126, .T. ) ;
#73821=AXIS2_PLACEMENT_3D ( 'NONE', #98690, #76850, #7447 ) ;
#73825=ORIENTED_EDGE ( 'NONE', *, *, #92683, .F. ) ;
#73826=AXIS2_PLACEMENT_3D ( 'NONE', #88009, #79886, #96088 ) ;
#73842=ORIENTED_EDGE ( 'NONE', *, *, #13412, .F. ) ;
#73848=CARTESIAN_POINT ( 'NONE',  ( -19.65312891409030271, 93.06504152958497400, 59.99999999999999289 ) ) ;
#73850=AXIS2_PLACEMENT_3D ( 'NONE', #56582, #33812, #62672 ) ;
#73852=CYLINDRICAL_SURFACE ( 'NONE', #44961, 70.00000000000002842 ) ;
#73856=ORIENTED_EDGE ( 'NONE', *, *, #31023, .T. ) ;
#73857=ORIENTED_EDGE ( 'NONE', *, *, #60899, .F. ) ;
#73869=EDGE_LOOP ( 'NONE', ( #84702, #39444, #62892, #72528 ) ) ;
#73872=ORIENTED_EDGE ( 'NONE', *, *, #8000, .F. ) ;
#73873=ORIENTED_EDGE ( 'NONE', *, *, #92441, .T. ) ;
#73874=EDGE_CURVE ( 'NONE', #51421, #28368, #24144, .T. ) ;
#73876=EDGE_CURVE ( 'NONE', #22609, #27174, #69735, .T. ) ;
#73882=ORIENTED_EDGE ( 'NONE', *, *, #10017, .F. ) ;
#73883=EDGE_CURVE ( 'NONE', #6477, #98545, #93577, .T. ) ;
#73887=EDGE_CURVE ( 'NONE', #42808, #59347, #78360, .T. ) ;
#73896=ORIENTED_EDGE ( 'NONE', *, *, #21394, .T. ) ;
#73897=VECTOR ( 'NONE', #23123, 1000.000000000000000 ) ;
#73906=DIRECTION ( 'NONE',  ( 0.000000000000000000, 0.000000000000000000, 1.000000000000000000 ) ) ;
#73907=DIRECTION ( 'NONE',  ( -0.000000000000000000, -0.000000000000000000, -1.000000000000000000 ) ) ;
#73920=CARTESIAN_POINT ( 'NONE',  ( -50.36082798260552806, 30.16005589317048674, 10.00000000000000000 ) ) ;
#73922=LINE ( 'NONE', #48632, #66311 ) ;
#73923=VECTOR ( 'NONE', #77201, 1000.000000000000114 ) ;
#73926=LINE ( 'NONE', #19253, #46827 ) ;
#73932=EDGE_CURVE ( 'NONE', #99285, #79909, #89496, .T. ) ;
#73939=LINE ( 'NONE', #27831, #55398 ) ;
#73943=CARTESIAN_POINT ( 'NONE',  ( -8.669243101527598583, 25.19333184544593252, -10.00000000000000000 ) ) ;
#73947=FACE_OUTER_BOUND ( 'NONE', #24377, .T. ) ;
#73949=VERTEX_POINT ( 'NONE', #26151 ) ;
#73954=EDGE_CURVE ( 'NONE', #17465, #44815, #10961, .T. ) ;
#73956=ORIENTED_EDGE ( 'NONE', *, *, #56591, .T. ) ;
#73959=DIRECTION ( 'NONE',  ( 0.000000000000000000, 0.000000000000000000, 1.000000000000000000 ) ) ;
#73964=CARTESIAN_POINT ( 'NONE',  ( -66.69146994933839778, 41.22495595238228105, -10.00000000000000000 ) ) ;
#73965=EDGE_LOOP ( 'NONE', ( #24981, #76028, #6917, #7031 ) ) ;
#73966=VECTOR ( 'NONE', #79467, 1000.000000000000114 ) ;
#73970=DIRECTION ( 'NONE',  ( -0.6141984594095519778, -0.7891516029629116469, 0.000000000000000000 ) ) ;
#73971=EDGE_CURVE ( 'NONE', #77610, #73457, #73255, .T. ) ;
#73977=ORIENTED_EDGE ( 'NONE', *, *, #69517, .F. ) ;
#73979=AXIS2_PLACEMENT_3D ( 'NONE', #83750, #71526, #56289 ) ;
#73981=CARTESIAN_POINT ( 'NONE',  ( -19.65312891409030271, 93.06504152958497400, -20.00000000000000355 ) ) ;
#73986=CARTESIAN_POINT ( 'NONE',  ( -19.65312891409030271, 93.06504152958497400, 177.5919119679930134 ) ) ;
#73990=CARTESIAN_POINT ( 'NONE',  ( 42.76202708541288899, 64.24573752441608576, -10.00000000000000000 ) ) ;
#73998=ADVANCED_FACE ( 'NONE', ( #42327 ), #25656, .F. ) ;
#73999=FACE_BOUND ( 'NONE', #50676, .T. ) ;
#74008=EDGE_CURVE ( 'NONE', #76358, #16775, #96089, .T. ) ;
#74016=EDGE_CURVE ( 'NONE', #2736, #17295, #40445, .T. ) ;
#74019=FACE_OUTER_BOUND ( 'NONE', #70048, .T. ) ;
#74024=VERTEX_POINT ( 'NONE', #64142 ) ;
#74026=CARTESIAN_POINT ( 'NONE',  ( 37.34220537994157496, 54.61056725541210710, 10.00000000000000000 ) ) ;
#74030=PLANE ( 'NONE',  #68023 ) ;
#74039=DIRECTION ( 'NONE',  ( -0.000000000000000000, -0.000000000000000000, -1.000000000000000000 ) ) ;
#74041=AXIS2_PLACEMENT_3D ( 'NONE', #89695, #20254, #20758 ) ;
#74050=AXIS2_PLACEMENT_3D ( 'NONE', #7485, #38377, #15573 ) ;
#74053=ORIENTED_EDGE ( 'NONE', *, *, #18748, .F. ) ;
#74054=VECTOR ( 'NONE', #44428, 1000.000000000000227 ) ;
#74069=CARTESIAN_POINT ( 'NONE',  ( 36.10619739613039059, 52.83927550304669296, -10.00000000000000000 ) ) ;
#74074=CARTESIAN_POINT ( 'NONE',  ( 33.92732256784238132, 47.61654385008751689, 10.00000000000000000 ) ) ;
#74081=EDGE_CURVE ( 'NONE', #25798, #65437, #56536, .T. ) ;
#74101=ORIENTED_EDGE ( 'NONE', *, *, #8863, .T. ) ;
#74106=VERTEX_POINT ( 'NONE', #22021 ) ;
#74108=AXIS2_PLACEMENT_3D ( 'NONE', #12904, #36162, #26594 ) ;
#74111=ORIENTED_EDGE ( 'NONE', *, *, #64828, .T. ) ;
#74112=DIRECTION ( 'NONE',  ( 0.5078630399532038098, 0.8614378286617615510, 0.000000000000000000 ) ) ;
#74115=VECTOR ( 'NONE', #58800, 1000.000000000000000 ) ;
#74122=VERTEX_POINT ( 'NONE', #82878 ) ;
#74128=ORIENTED_EDGE ( 'NONE', *, *, #70159, .T. ) ;
#74137=CARTESIAN_POINT ( 'NONE',  ( -19.65312891409030271, 93.06504152958497400, -10.00000000000000888 ) ) ;
#74141=AXIS2_PLACEMENT_3D ( 'NONE', #25200, #86077, #38895 ) ;
#74146=LINE ( 'NONE', #27543, #49940 ) ;
#74148=DIRECTION ( 'NONE',  ( 0.7751245550734536804, 0.6318084552474590998, 0.000000000000000000 ) ) ;
#74152=ADVANCED_FACE ( 'NONE', ( #44318 ), #6824, .T. ) ;
#74157=ORIENTED_EDGE ( 'NONE', *, *, #97779, .F. ) ;
#74159=FACE_OUTER_BOUND ( 'NONE', #11175, .T. ) ;
#74161=CARTESIAN_POINT ( 'NONE',  ( 49.91331508509971115, 100.8438505198844553, 10.00000000000000000 ) ) ;
#74169=CARTESIAN_POINT ( 'NONE',  ( 26.37028381016232004, 40.32183835407518302, 10.00000000000000000 ) ) ;
#74171=CARTESIAN_POINT ( 'NONE',  ( 15.59500490259069139, 53.45320653094265140, 59.99999999999999289 ) ) ;
#74183=CARTESIAN_POINT ( 'NONE',  ( 47.28113444070024229, 72.57591296950350568, 10.00000000000000000 ) ) ;
#74187=EDGE_CURVE ( 'NONE', #63013, #3586, #32621, .T. ) ;
#74189=AXIS2_PLACEMENT_3D ( 'NONE', #54729, #1054, #39027 ) ;
#74191=CARTESIAN_POINT ( 'NONE',  ( 38.52196584993465223, 56.41980893122115504, -10.00000000000000000 ) ) ;
#74192=VECTOR ( 'NONE', #26443, 1000.000000000000000 ) ;
#74213=FACE_OUTER_BOUND ( 'NONE', #26601, .T. ) ;
#74217=EDGE_LOOP ( 'NONE', ( #10547, #68609, #85470, #82379 ) ) ;
#74224=ORIENTED_EDGE ( 'NONE', *, *, #10832, .T. ) ;
#74233=DIRECTION ( 'NONE',  ( -0.9879428538673736826, -0.1548189829846108034, 0.000000000000000000 ) ) ;
#74239=ORIENTED_EDGE ( 'NONE', *, *, #11339, .F. ) ;
#74240=DIRECTION ( 'NONE',  ( 1.000000000000000000, 0.000000000000000000, 0.000000000000000000 ) ) ;
#74249=CARTESIAN_POINT ( 'NONE',  ( 32.07315653955451040, 47.77038272570916888, -10.00000000000000000 ) ) ;
#74250=ORIENTED_EDGE ( 'NONE', *, *, #16187, .T. ) ;
#74255=ORIENTED_EDGE ( 'NONE', *, *, #3970, .T. ) ;
#74271=VECTOR ( 'NONE', #66308, 1000.000000000000227 ) ;
#74272=CARTESIAN_POINT ( 'NONE',  ( -44.49648453423615990, 28.96346851210257611, -10.00000000000000000 ) ) ;
#74278=VECTOR ( 'NONE', #87643, 1000.000000000000114 ) ;
#74279=ORIENTED_EDGE ( 'NONE', *, *, #38510, .T. ) ;
#74281=VECTOR ( 'NONE', #27870, 1000.000000000000000 ) ;
#74290=CARTESIAN_POINT ( 'NONE',  ( -23.47208873469913115, 24.42380372261332155, -10.00000000000000000 ) ) ;
#74292=VERTEX_POINT ( 'NONE', #41711 ) ;
#74298=CARTESIAN_POINT ( 'NONE',  ( -57.88150100324660485, 35.92665207732902388, -10.00000000000000000 ) ) ;
#74300=EDGE_CURVE ( 'NONE', #88206, #46023, #94962, .T. ) ;
#74304=VECTOR ( 'NONE', #60924, 1000.000000000000000 ) ;
#74308=ORIENTED_EDGE ( 'NONE', *, *, #73887, .F. ) ;
#74309=DIRECTION ( 'NONE',  ( -1.000000000000000000, 0.000000000000000000, 0.000000000000000000 ) ) ;
#74314=FACE_OUTER_BOUND ( 'NONE', #59878, .T. ) ;
#74325=CARTESIAN_POINT ( 'NONE',  ( 32.07315653955450330, 47.77038272570916888, -10.00000000000000000 ) ) ;
#74331=AXIS2_PLACEMENT_3D ( 'NONE', #49019, #71833, #10519 ) ;
#74341=ORIENTED_EDGE ( 'NONE', *, *, #90386, .F. ) ;
#74343=AXIS2_PLACEMENT_3D ( 'NONE', #68026, #52321, #44215 ) ;
#74346=LINE ( 'NONE', #96660, #39618 ) ;
#74347=VERTEX_POINT ( 'NONE', #48839 ) ;
#74348=EDGE_CURVE ( 'NONE', #98895, #88538, #72655, .T. ) ;
#74363=DIRECTION ( 'NONE',  ( -0.000000000000000000, -0.000000000000000000, -1.000000000000000000 ) ) ;
#74365=EDGE_CURVE ( 'NONE', #77218, #58030, #3738, .T. ) ;
#74368=ORIENTED_EDGE ( 'NONE', *, *, #43760, .F. ) ;
#74372=CARTESIAN_POINT ( 'NONE',  ( 25.34687108590969729, 93.06504152958497400, 45.00000000000000711 ) ) ;
#74378=DIRECTION ( 'NONE',  ( 0.3103181967972123423, -0.9506327454577433445, 0.000000000000000000 ) ) ;
#74380=VERTEX_POINT ( 'NONE', #34615 ) ;
#74392=VERTEX_POINT ( 'NONE', #11837 ) ;
#74393=DIRECTION ( 'NONE',  ( 0.000000000000000000, 0.000000000000000000, 1.000000000000000000 ) ) ;
#74396=ORIENTED_EDGE ( 'NONE', *, *, #34932, .F. ) ;
#74402=VERTEX_POINT ( 'NONE', #58405 ) ;
#74405=ORIENTED_EDGE ( 'NONE', *, *, #61760, .F. ) ;
#74406=VECTOR ( 'NONE', #35236, 1000.000000000000000 ) ;
#74415=ORIENTED_EDGE ( 'NONE', *, *, #37950, .T. ) ;
#74419=DIRECTION ( 'NONE',  ( 1.000000000000000000, 0.000000000000000000, 0.000000000000000000 ) ) ;
#74433=AXIS2_PLACEMENT_3D ( 'NONE', #55978, #38796, #9923 ) ;
#74434=DIRECTION ( 'NONE',  ( -0.4621356007560455392, 0.8868092729070039537, 0.000000000000000000 ) ) ;
#74441=FACE_OUTER_BOUND ( 'NONE', #86355, .T. ) ;
#74445=ORIENTED_EDGE ( 'NONE', *, *, #87798, .T. ) ;
#74460=EDGE_CURVE ( 'NONE', #67048, #57230, #1624, .T. ) ;
#74467=ORIENTED_EDGE ( 'NONE', *, *, #67191, .T. ) ;
#74470=CARTESIAN_POINT ( 'NONE',  ( 46.80963145949300497, 71.09457308843315104, 10.00000000000000000 ) ) ;
#74472=AXIS2_PLACEMENT_3D ( 'NONE', #53739, #37547, #29960 ) ;
#74473=DIRECTION ( 'NONE',  ( -0.3371987438498166290, 0.9414334852479520066, 0.000000000000000000 ) ) ;
#74478=FACE_OUTER_BOUND ( 'NONE', #55439, .T. ) ;
#74480=CARTESIAN_POINT ( 'NONE',  ( 0.1270659342858249108, 66.35802143352867688, -10.00000000000000000 ) ) ;
#74483=ORIENTED_EDGE ( 'NONE', *, *, #7153, .F. ) ;
#74485=CARTESIAN_POINT ( 'NONE',  ( 5.476650724650769853, 71.31612877608863243, -10.00000000000000000 ) ) ;
#74487=LINE ( 'NONE', #43546, #55310 ) ;
#74488=ORIENTED_EDGE ( 'NONE', *, *, #34307, .F. ) ;
#74492=AXIS2_PLACEMENT_3D ( 'NONE', #11123, #73907, #66298 ) ;
#74495=DIRECTION ( 'NONE',  ( -0.000000000000000000, -0.000000000000000000, -1.000000000000000000 ) ) ;
#74503=DIRECTION ( 'NONE',  ( -0.000000000000000000, -0.000000000000000000, 1.000000000000000000 ) ) ;
#74505=ORIENTED_EDGE ( 'NONE', *, *, #83747, .F. ) ;
#74513=DIRECTION ( 'NONE',  ( 0.000000000000000000, 0.000000000000000000, 1.000000000000000000 ) ) ;
#74528=EDGE_CURVE ( 'NONE', #8947, #2862, #45681, .T. ) ;
#74534=PLANE ( 'NONE',  #40005 ) ;
#74537=CARTESIAN_POINT ( 'NONE',  ( 44.18794977381975286, 118.5901545549086791, -10.00000000000000000 ) ) ;
#74540=LINE ( 'NONE', #98327, #3335 ) ;
#74544=DIRECTION ( 'NONE',  ( -0.3473448497826262527, 0.9377374661009790779, 0.000000000000000000 ) ) ;
#74547=EDGE_CURVE ( 'NONE', #29146, #88681, #93873, .T. ) ;
#74551=FACE_OUTER_BOUND ( 'NONE', #48034, .T. ) ;
#74565=CARTESIAN_POINT ( 'NONE',  ( -19.65312891409030271, 93.06504152958497400, 59.99999999999999289 ) ) ;
#74590=EDGE_CURVE ( 'NONE', #71916, #32467, #51706, .T. ) ;
#74599=DIRECTION ( 'NONE',  ( 0.000000000000000000, 0.000000000000000000, -1.000000000000000000 ) ) ;
#74616=CARTESIAN_POINT ( 'NONE',  ( 21.15788363470973366, 37.74176219324818504, -10.00000000000000000 ) ) ;
#74623=ORIENTED_EDGE ( 'NONE', *, *, #16964, .T. ) ;
#74624=CARTESIAN_POINT ( 'NONE',  ( -36.26652983198114555, 26.35523046909639788, 10.00000000000000000 ) ) ;
#74633=PLANE ( 'NONE',  #88775 ) ;
#74637=CIRCLE ( 'NONE', #30918, 70.00000000000001421 ) ;
#74647=ORIENTED_EDGE ( 'NONE', *, *, #75166, .F. ) ;
#74654=EDGE_LOOP ( 'NONE', ( #96122, #73977, #95976, #52399 ) ) ;
#74668=EDGE_CURVE ( 'NONE', #43732, #32399, #36984, .T. ) ;
#74676=VERTEX_POINT ( 'NONE', #44570 ) ;
#74679=ADVANCED_FACE ( 'NONE', ( #35982 ), #90746, .F. ) ;
#74686=DIRECTION ( 'NONE',  ( 0.000000000000000000, 0.000000000000000000, 1.000000000000000000 ) ) ;
#74694=CARTESIAN_POINT ( 'NONE',  ( -69.42519150082246426, 45.64199051378594874, 10.00000000000000000 ) ) ;
#74712=LINE ( 'NONE', #37656, #52974 ) ;
#74713=CARTESIAN_POINT ( 'NONE',  ( 23.64814127513158937, 118.0650415295850451, 20.00000000000000355 ) ) ;
#74715=EDGE_CURVE ( 'NONE', #81514, #14058, #6090, .T. ) ;
#74726=ADVANCED_FACE ( 'NONE', ( #66395 ), #97323, .T. ) ;
#74733=DIRECTION ( 'NONE',  ( -0.9302793824855948301, 0.3668518372888711077, 0.000000000000000000 ) ) ;
#74739=PLANE ( 'NONE',  #53203 ) ;
#74740=EDGE_LOOP ( 'NONE', ( #61717, #50935, #27453, #23367 ) ) ;
#74753=VERTEX_POINT ( 'NONE', #12718 ) ;
#74755=ORIENTED_EDGE ( 'NONE', *, *, #26886, .F. ) ;
#74770=VERTEX_POINT ( 'NONE', #64223 ) ;
#74773=ORIENTED_EDGE ( 'NONE', *, *, #77997, .T. ) ;
#74779=LINE ( 'NONE', #4872, #81956 ) ;
#74783=LINE ( 'NONE', #43844, #78528 ) ;
#74795=FACE_OUTER_BOUND ( 'NONE', #27623, .T. ) ;
#74798=LINE ( 'NONE', #82912, #56516 ) ;
#74800=EDGE_CURVE ( 'NONE', #5467, #31605, #89096, .T. ) ;
#74804=ADVANCED_FACE ( 'NONE', ( #40899 ), #2958, .F. ) ;
#74822=CARTESIAN_POINT ( 'NONE',  ( 27.58098951138967436, 43.10352854649765675, -10.00000000000000000 ) ) ;
#74823=EDGE_CURVE ( 'NONE', #44698, #12428, #50509, .T. ) ;
#74831=CARTESIAN_POINT ( 'NONE',  ( 8.106622824862185439, 30.17147933776454494, -10.00000000000000000 ) ) ;
#74836=CARTESIAN_POINT ( 'NONE',  ( -71.61465314115659453, 63.06504152958490295, 25.00000000000000000 ) ) ;
#74854=ORIENTED_EDGE ( 'NONE', *, *, #59683, .T. ) ;
#74856=ORIENTED_EDGE ( 'NONE', *, *, #49055, .T. ) ;
#74857=DIRECTION ( 'NONE',  ( -0.1654779384134469067, 0.9862134920484689760, 0.000000000000000000 ) ) ;
#74861=DIRECTION ( 'NONE',  ( -0.8653701635463872943, 0.5011331959107268030, 0.000000000000000000 ) ) ;
#74868=ORIENTED_EDGE ( 'NONE', *, *, #83291, .F. ) ;
#74873=CARTESIAN_POINT ( 'NONE',  ( 43.16562282991919375, 123.9487658730721904, 10.00000000000000000 ) ) ;
#74879=CARTESIAN_POINT ( 'NONE',  ( -36.70227853217910763, 37.68578735097466392, 59.99999999999999289 ) ) ;
#74884=ORIENTED_EDGE ( 'NONE', *, *, #38972, .F. ) ;
#74891=ORIENTED_EDGE ( 'NONE', *, *, #7775, .F. ) ;
#74892=ORIENTED_EDGE ( 'NONE', *, *, #63303, .T. ) ;
#74894=EDGE_LOOP ( 'NONE', ( #71131, #12316, #8419, #19210 ) ) ;
#74895=AXIS2_PLACEMENT_3D ( 'NONE', #91989, #53426, #56922 ) ;
#74897=CARTESIAN_POINT ( 'NONE',  ( -80.08603253397792798, 57.73992072201551906, -10.00000000000000000 ) ) ;
#74901=CARTESIAN_POINT ( 'NONE',  ( 27.76992210170819675, 43.29297894285233639, 10.00000000000000000 ) ) ;
#74908=ADVANCED_FACE ( 'NONE', ( #41409 ), #81460, .F. ) ;
#74911=ADVANCED_FACE ( 'NONE', ( #64735 ), #12034, .F. ) ;
#74932=DIRECTION ( 'NONE',  ( 0.000000000000000000, 0.000000000000000000, 1.000000000000000000 ) ) ;
#74949=DIRECTION ( 'NONE',  ( 0.000000000000000000, 0.000000000000000000, 1.000000000000000000 ) ) ;
#74953=VERTEX_POINT ( 'NONE', #52017 ) ;
#74958=CYLINDRICAL_SURFACE ( 'NONE', #58041, 70.00000000000002842 ) ;
#74959=VERTEX_POINT ( 'NONE', #44399 ) ;
#74960=VECTOR ( 'NONE', #31332, 1000.000000000000114 ) ;
#74963=CYLINDRICAL_SURFACE ( 'NONE', #78280, 70.00000000000002842 ) ;
#74965=CARTESIAN_POINT ( 'NONE',  ( -28.78582490886478240, 40.83341904737610406, 59.99999999999999289 ) ) ;
#74967=EDGE_CURVE ( 'NONE', #14070, #72951, #7919, .T. ) ;
#74974=ORIENTED_EDGE ( 'NONE', *, *, #18531, .F. ) ;
#74983=PLANE ( 'NONE',  #5981 ) ;
#74984=CARTESIAN_POINT ( 'NONE',  ( -57.46197106626858186, 34.15416430719361074, -10.00000000000000000 ) ) ;
#74986=ADVANCED_FACE ( 'NONE', ( #94419 ), #48289, .F. ) ;
#74991=LINE ( 'NONE', #65377, #28533 ) ;
#74995=ORIENTED_EDGE ( 'NONE', *, *, #63540, .T. ) ;
#74998=DIRECTION ( 'NONE',  ( -0.8492021815265757834, 0.5280678506503729830, 0.000000000000000000 ) ) ;
#75006=VERTEX_POINT ( 'NONE', #24973 ) ;
#75010=ORIENTED_EDGE ( 'NONE', *, *, #31526, .T. ) ;
#75011=CARTESIAN_POINT ( 'NONE',  ( 36.25628400652970384, 53.06077264917335867, 10.00000000000000000 ) ) ;
#75013=CARTESIAN_POINT ( 'NONE',  ( 24.86884376670136021, 66.72197582601074828, 59.99999999999999289 ) ) ;
#75018=ORIENTED_EDGE ( 'NONE', *, *, #27574, .T. ) ;
#75021=VERTEX_POINT ( 'NONE', #79234 ) ;
#75029=VECTOR ( 'NONE', #75198, 1000.000000000000114 ) ;
#75030=CYLINDRICAL_SURFACE ( 'NONE', #4913, 70.00000000000002842 ) ;
#75034=VECTOR ( 'NONE', #98635, 1000.000000000000114 ) ;
#75038=EDGE_CURVE ( 'NONE', #66534, #2736, #31193, .T. ) ;
#75039=AXIS2_PLACEMENT_3D ( 'NONE', #94889, #77678, #9262 ) ;
#75040=LINE ( 'NONE', #14216, #61056 ) ;
#75075=LINE ( 'NONE', #98876, #83969 ) ;
#75082=LINE ( 'NONE', #92666, #66173 ) ;
#75084=EDGE_CURVE ( 'NONE', #45792, #3742, #87854, .T. ) ;
#75093=CARTESIAN_POINT ( 'NONE',  ( -19.65312891409030271, 93.06504152958497400, -10.00000000000000888 ) ) ;
#75097=CIRCLE ( 'NONE', #47516, 70.00000000000001421 ) ;
#75098=ORIENTED_EDGE ( 'NONE', *, *, #68953, .T. ) ;
#75110=AXIS2_PLACEMENT_3D ( 'NONE', #17748, #70950, #25330 ) ;
#75123=CARTESIAN_POINT ( 'NONE',  ( 45.57373283677818421, 114.7827874512443032, -10.00000000000000000 ) ) ;
#75124=ORIENTED_EDGE ( 'NONE', *, *, #82629, .T. ) ;
#75130=DIRECTION ( 'NONE',  ( -1.000000000000000000, 0.000000000000000000, 0.000000000000000000 ) ) ;
#75138=DIRECTION ( 'NONE',  ( -0.9607486656258038549, -0.2774202615135334948, 0.000000000000000000 ) ) ;
#75140=VERTEX_POINT ( 'NONE', #72613 ) ;
#75151=LINE ( 'NONE', #50333, #54839 ) ;
#75157=ADVANCED_FACE ( 'NONE', ( #61349 ), #45641, .F. ) ;
#75163=CARTESIAN_POINT ( 'NONE',  ( 27.58098951138967436, 43.10352854649765675, -10.00000000000000000 ) ) ;
#75165=LINE ( 'NONE', #90897, #12288 ) ;
#75166=EDGE_CURVE ( 'NONE', #57534, #78966, #91299, .T. ) ;
#75179=VECTOR ( 'NONE', #81257, 999.9999999999998863 ) ;
#75190=DIRECTION ( 'NONE',  ( -0.000000000000000000, 0.000000000000000000, -1.000000000000000000 ) ) ;
#75198=DIRECTION ( 'NONE',  ( -0.3653410243663964274, -0.9308737486442036912, 0.000000000000000000 ) ) ;
#75203=ORIENTED_EDGE ( 'NONE', *, *, #57683, .T. ) ;
#75206=DIRECTION ( 'NONE',  ( -0.9874733399847777093, -0.1577859398657163736, 0.000000000000000000 ) ) ;
#75209=VERTEX_POINT ( 'NONE', #52747 ) ;
#75220=ORIENTED_EDGE ( 'NONE', *, *, #46920, .T. ) ;
#75225=ADVANCED_FACE ( 'NONE', ( #61842 ), #14266, .F. ) ;
#75227=CYLINDRICAL_SURFACE ( 'NONE', #50785, 70.00000000000002842 ) ;
#75236=VERTEX_POINT ( 'NONE', #67464 ) ;
#75240=EDGE_CURVE ( 'NONE', #56390, #99391, #69594, .T. ) ;
#75243=VECTOR ( 'NONE', #34503, 1000.000000000000000 ) ;
#75247=LINE ( 'NONE', #90484, #23285 ) ;
#75249=LINE ( 'NONE', #68120, #64061 ) ;
#75265=CARTESIAN_POINT ( 'NONE',  ( 27.76992210170820030, 43.29297894285232928, -10.00000000000000000 ) ) ;
#75267=LINE ( 'NONE', #74290, #1152 ) ;
#75272=ORIENTED_EDGE ( 'NONE', *, *, #46143, .F. ) ;
#75283=AXIS2_PLACEMENT_3D ( 'NONE', #93045, #53515, #54493 ) ;
#75287=ORIENTED_EDGE ( 'NONE', *, *, #56923, .F. ) ;
#75288=DIRECTION ( 'NONE',  ( -0.000000000000000000, 0.000000000000000000, -1.000000000000000000 ) ) ;
#75289=LINE ( 'NONE', #69650, #82049 ) ;
#75309=DIRECTION ( 'NONE',  ( 1.000000000000000000, 0.000000000000000000, 0.000000000000000000 ) ) ;
#75312=LINE ( 'NONE', #82935, #20598 ) ;
#75319=DIRECTION ( 'NONE',  ( 0.3400251696390308997, -0.9404163354663445107, 0.000000000000000000 ) ) ;
#75326=CARTESIAN_POINT ( 'NONE',  ( -19.79170892150624894, 93.03488659321679677, 59.99999999999999289 ) ) ;
#75327=CARTESIAN_POINT ( 'NONE',  ( 48.43557798863805886, 76.81918075477977936, 10.00000000000000000 ) ) ;
#75330=PLANE ( 'NONE',  #49113 ) ;
#75340=ORIENTED_EDGE ( 'NONE', *, *, #40958, .F. ) ;
#75354=AXIS2_PLACEMENT_3D ( 'NONE', #61151, #12212, #12723 ) ;
#75357=DIRECTION ( 'NONE',  ( -1.000000000000000000, 0.000000000000000000, 0.000000000000000000 ) ) ;
#75358=EDGE_CURVE ( 'NONE', #18338, #34850, #84961, .T. ) ;
#75376=DIRECTION ( 'NONE',  ( -1.000000000000000000, 0.000000000000000000, 0.000000000000000000 ) ) ;
#75385=ORIENTED_EDGE ( 'NONE', *, *, #50876, .F. ) ;
#75386=VECTOR ( 'NONE', #55500, 999.9999999999998863 ) ;
#75388=ADVANCED_FACE ( 'NONE', ( #77842 ), #63620, .T. ) ;
#75395=DIRECTION ( 'NONE',  ( -0.7299047266382303611, 0.6835488936653839609, 0.000000000000000000 ) ) ;
#75416=DIRECTION ( 'NONE',  ( -1.000000000000000000, 0.000000000000000000, 0.000000000000000000 ) ) ;
#75425=EDGE_CURVE ( 'NONE', #98025, #8702, #56586, .T. ) ;
#75426=CARTESIAN_POINT ( 'NONE',  ( -19.65312891409030271, 93.06504152958497400, -10.00000000000000888 ) ) ;
#75427=DIRECTION ( 'NONE',  ( 0.000000000000000000, -0.000000000000000000, -1.000000000000000000 ) ) ;
#75428=FACE_OUTER_BOUND ( 'NONE', #7457, .T. ) ;
#75449=ORIENTED_EDGE ( 'NONE', *, *, #26886, .T. ) ;
#75453=ORIENTED_EDGE ( 'NONE', *, *, #80226, .T. ) ;
#75469=CARTESIAN_POINT ( 'NONE',  ( 33.30115378465513487, 95.78395070760240060, 59.99999999999999289 ) ) ;
#75477=EDGE_CURVE ( 'NONE', #38318, #60221, #79337, .T. ) ;
#75487=AXIS2_PLACEMENT_3D ( 'NONE', #54251, #85222, #46674 ) ;
#75489=VECTOR ( 'NONE', #52062, 1000.000000000000114 ) ;
#75496=PLANE ( 'NONE',  #54688 ) ;
#75498=VECTOR ( 'NONE', #73378, 999.9999999999998863 ) ;
#75501=ORIENTED_EDGE ( 'NONE', *, *, #66557, .T. ) ;
#75507=DIRECTION ( 'NONE',  ( 0.000000000000000000, 0.000000000000000000, 1.000000000000000000 ) ) ;
#75510=CARTESIAN_POINT ( 'NONE',  ( -64.94778771796556782, 41.33875607593970614, -10.00000000000000000 ) ) ;
#75513=VECTOR ( 'NONE', #90237, 1000.000000000000000 ) ;
#75519=DIRECTION ( 'NONE',  ( -0.7957378174433876739, 0.6056412518070690698, 0.000000000000000000 ) ) ;
#75544=PLANE ( 'NONE',  #4709 ) ;
#75548=VECTOR ( 'NONE', #98310, 1000.000000000000000 ) ;
#75557=AXIS2_PLACEMENT_3D ( 'NONE', #18813, #65891, #12210 ) ;
#75585=DIRECTION ( 'NONE',  ( 0.000000000000000000, 0.000000000000000000, 1.000000000000000000 ) ) ;
#75587=EDGE_LOOP ( 'NONE', ( #40126, #13332, #94544, #67274 ) ) ;
#75588=EDGE_LOOP ( 'NONE', ( #46287, #95252, #90205, #19897 ) ) ;
#75591=CARTESIAN_POINT ( 'NONE',  ( 1.813001633210440833, 27.74720351945396857, -10.00000000000000000 ) ) ;
#75594=CARTESIAN_POINT ( 'NONE',  ( 46.32860941106299890, 116.4404604047837779, -10.00000000000000000 ) ) ;
#75596=LINE ( 'NONE', #98903, #58059 ) ;
#75602=CARTESIAN_POINT ( 'NONE',  ( -56.23827824165702793, 48.13106613502690578, 59.99999999999999289 ) ) ;
#75606=ORIENTED_EDGE ( 'NONE', *, *, #35387, .T. ) ;
#75609=FACE_OUTER_BOUND ( 'NONE', #2604, .T. ) ;
#75616=CARTESIAN_POINT ( 'NONE',  ( -22.09748208295713567, 35.17237849129525529, 59.99999999999999289 ) ) ;
#75621=VECTOR ( 'NONE', #43881, 1000.000000000000000 ) ;
#75624=CARTESIAN_POINT ( 'NONE',  ( 42.16454434324482747, 125.9067112960471349, 10.00000000000000000 ) ) ;
#75633=LINE ( 'NONE', #6219, #78062 ) ;
#75641=DIRECTION ( 'NONE',  ( 0.2473641778533817170, 0.9689225787001356505, 0.000000000000000000 ) ) ;
#75645=DIRECTION ( 'NONE',  ( -0.000000000000000000, -0.000000000000000000, -1.000000000000000000 ) ) ;
#75650=EDGE_CURVE ( 'NONE', #48026, #36578, #8855, .T. ) ;
#75651=LINE ( 'NONE', #90397, #68901 ) ;
#75653=ORIENTED_EDGE ( 'NONE', *, *, #78939, .F. ) ;
#75659=EDGE_CURVE ( 'NONE', #66853, #81845, #84399, .T. ) ;
#75666=EDGE_CURVE ( 'NONE', #65627, #59009, #77778, .T. ) ;
#75686=VECTOR ( 'NONE', #75519, 1000.000000000000000 ) ;
#75704=AXIS2_PLACEMENT_3D ( 'NONE', #53508, #14530, #62093 ) ;
#75715=ORIENTED_EDGE ( 'NONE', *, *, #81366, .F. ) ;
#75716=DIRECTION ( 'NONE',  ( 0.9999986627203610867, -0.001635407438361276495, 0.000000000000000000 ) ) ;
#75719=ORIENTED_EDGE ( 'NONE', *, *, #61527, .F. ) ;
#75723=ORIENTED_EDGE ( 'NONE', *, *, #35055, .F. ) ;
#75736=ORIENTED_EDGE ( 'NONE', *, *, #33722, .F. ) ;
#75761=FACE_OUTER_BOUND ( 'NONE', #84734, .T. ) ;
#75764=DIRECTION ( 'NONE',  ( -1.000000000000000000, 0.000000000000000000, 0.000000000000000000 ) ) ;
#75774=VECTOR ( 'NONE', #68418, 1000.000000000000000 ) ;
#75779=AXIS2_PLACEMENT_3D ( 'NONE', #63543, #94484, #1257 ) ;
#75786=AXIS2_PLACEMENT_3D ( 'NONE', #83756, #75138, #20948 ) ;
#75787=VERTEX_POINT ( 'NONE', #35148 ) ;
#75788=DIRECTION ( 'NONE',  ( -0.4621356007560363244, 0.8868092729070087277, 0.000000000000000000 ) ) ;
#75791=DIRECTION ( 'NONE',  ( -0.8495546651763560275, -0.5275005885087612478, 0.000000000000000000 ) ) ;
#75797=DIRECTION ( 'NONE',  ( -0.9172102815912978047, -0.3984034379159046568, 0.000000000000000000 ) ) ;
#75801=VECTOR ( 'NONE', #94965, 1000.000000000000114 ) ;
#75810=DIRECTION ( 'NONE',  ( -0.01068548594337170865, 0.9999429085653609439, 0.000000000000000000 ) ) ;
#75812=EDGE_CURVE ( 'NONE', #78693, #55881, #83278, .T. ) ;
#75813=PLANE ( 'NONE',  #60989 ) ;
#75814=VECTOR ( 'NONE', #21329, 999.9999999999998863 ) ;
#75827=LINE ( 'NONE', #75326, #11144 ) ;
#75828=CARTESIAN_POINT ( 'NONE',  ( -78.57153713424663977, 57.64153020465174393, -10.00000000000000000 ) ) ;
#75840=CARTESIAN_POINT ( 'NONE',  ( -13.42108286626701386, 23.34301056334149038, -10.00000000000000000 ) ) ;
#75842=EDGE_CURVE ( 'NONE', #24595, #6796, #58442, .T. ) ;
#75843=EDGE_LOOP ( 'NONE', ( #59230, #61983, #3458, #99996 ) ) ;
#75851=ORIENTED_EDGE ( 'NONE', *, *, #95301, .F. ) ;
#75854=ADVANCED_FACE ( 'NONE', ( #22439 ), #45234, .F. ) ;
#75860=VECTOR ( 'NONE', #41345, 1000.000000000000114 ) ;
#75863=DIRECTION ( 'NONE',  ( 1.000000000000000000, 0.000000000000000000, 0.000000000000000000 ) ) ;
#75865=CARTESIAN_POINT ( 'NONE',  ( -72.30469571560091424, 48.86078274006646183, -10.00000000000000000 ) ) ;
#75870=DIRECTION ( 'NONE',  ( -0.000000000000000000, -0.000000000000000000, -1.000000000000000000 ) ) ;
#75873=FACE_OUTER_BOUND ( 'NONE', #19426, .T. ) ;
#75875=DIRECTION ( 'NONE',  ( 1.000000000000000000, 0.000000000000000000, 0.000000000000000000 ) ) ;
#75887=ORIENTED_EDGE ( 'NONE', *, *, #91423, .F. ) ;
#75897=VERTEX_POINT ( 'NONE', #69029 ) ;
#75899=ORIENTED_EDGE ( 'NONE', *, *, #99840, .T. ) ;
#75907=VERTEX_POINT ( 'NONE', #60922 ) ;
#75915=DIRECTION ( 'NONE',  ( -0.2575544297740129385, 0.9662637919863205083, 0.000000000000000000 ) ) ;
#75923=DIRECTION ( 'NONE',  ( 0.6544109481086042290, 0.7561390817803280706, 0.000000000000000000 ) ) ;
#75925=EDGE_CURVE ( 'NONE', #62719, #17777, #60420, .T. ) ;
#75926=AXIS2_PLACEMENT_3D ( 'NONE', #93631, #24198, #86065 ) ;
#75929=DIRECTION ( 'NONE',  ( 0.3103181967972122313, -0.9506327454577433445, 0.000000000000000000 ) ) ;
#75933=ADVANCED_FACE ( 'NONE', ( #39111 ), #78151, .T. ) ;
#75939=VECTOR ( 'NONE', #6182, 1000.000000000000114 ) ;
#75947=VECTOR ( 'NONE', #83189, 1000.000000000000000 ) ;
#75954=CARTESIAN_POINT ( 'NONE',  ( 32.18695666311190706, 46.02670049433633181, 10.00000000000000000 ) ) ;
#75963=EDGE_CURVE ( 'NONE', #11410, #36862, #91887, .T. ) ;
#75969=FACE_OUTER_BOUND ( 'NONE', #68588, .T. ) ;
#75974=EDGE_CURVE ( 'NONE', #32652, #87428, #76644, .T. ) ;
#75976=DIRECTION ( 'NONE',  ( 1.000000000000000000, 0.000000000000000000, 0.000000000000000000 ) ) ;
#75978=CYLINDRICAL_SURFACE ( 'NONE', #11743, 45.00000000000000000 ) ;
#75984=EDGE_CURVE ( 'NONE', #78709, #95321, #6748, .T. ) ;
#75985=EDGE_LOOP ( 'NONE', ( #70401, #35952, #12252, #26358 ) ) ;
#75990=CARTESIAN_POINT ( 'NONE',  ( 47.89168550319194395, 74.68847913791599069, 10.00000000000000000 ) ) ;
#75993=CARTESIAN_POINT ( 'NONE',  ( -40.67952639183666008, 27.60432558407080350, -10.00000000000000000 ) ) ;
#75997=AXIS2_PLACEMENT_3D ( 'NONE', #91919, #69569, #91410 ) ;
#76001=ORIENTED_EDGE ( 'NONE', *, *, #13925, .F. ) ;
#76003=DIRECTION ( 'NONE',  ( -0.2502735827033040761, -0.9681751565707790164, 0.000000000000000000 ) ) ;
#76004=EDGE_LOOP ( 'NONE', ( #14408, #92613, #14438, #42409 ) ) ;
#76005=AXIS2_PLACEMENT_3D ( 'NONE', #91758, #22322, #53224 ) ;
#76008=FACE_BOUND ( 'NONE', #37165, .T. ) ;
#76015=EDGE_LOOP ( 'NONE', ( #3590, #46210, #54946, #3283 ) ) ;
#76016=AXIS2_PLACEMENT_3D ( 'NONE', #39420, #70338, #69345 ) ;
#76017=PLANE ( 'NONE',  #17104 ) ;
#76028=ORIENTED_EDGE ( 'NONE', *, *, #93985, .T. ) ;
#76032=CIRCLE ( 'NONE', #35579, 11.89249999999999652 ) ;
#76041=ORIENTED_EDGE ( 'NONE', *, *, #75963, .T. ) ;
#76046=EDGE_CURVE ( 'NONE', #40956, #99081, #46533, .T. ) ;
#76048=CARTESIAN_POINT ( 'NONE',  ( 41.50249547274756878, 124.4848494355456836, -10.00000000000000000 ) ) ;
#76055=CARTESIAN_POINT ( 'NONE',  ( 3.113790753877909712, 26.87087736965101570, -10.00000000000000000 ) ) ;
#76057=ORIENTED_EDGE ( 'NONE', *, *, #22610, .T. ) ;
#76069=CYLINDRICAL_SURFACE ( 'NONE', #39979, 70.00000000000002842 ) ;
#76073=AXIS2_PLACEMENT_3D ( 'NONE', #51105, #43994, #59186 ) ;
#76076=CARTESIAN_POINT ( 'NONE',  ( 40.48539884740146277, 126.3902902409112556, 10.00000000000000000 ) ) ;
#76080=LINE ( 'NONE', #7134, #77938 ) ;
#76094=ORIENTED_EDGE ( 'NONE', *, *, #76964, .F. ) ;
#76098=DIRECTION ( 'NONE',  ( -0.7226656227773308183, -0.6911977992267138715, 0.000000000000000000 ) ) ;
#76099=ORIENTED_EDGE ( 'NONE', *, *, #90386, .T. ) ;
#76100=CARTESIAN_POINT ( 'NONE',  ( -68.37628875030422648, 42.44405361048389125, -10.00000000000000000 ) ) ;
#76104=ORIENTED_EDGE ( 'NONE', *, *, #23068, .F. ) ;
#76105=ORIENTED_EDGE ( 'NONE', *, *, #83815, .T. ) ;
#76107=FACE_OUTER_BOUND ( 'NONE', #73233, .T. ) ;
#76108=EDGE_LOOP ( 'NONE', ( #19208, #92877, #100014, #97097 ) ) ;
#76120=ORIENTED_EDGE ( 'NONE', *, *, #94321, .F. ) ;
#76124=CARTESIAN_POINT ( 'NONE',  ( -38.61298035630893111, 26.97617139035147460, -10.00000000000000000 ) ) ;
#76127=DIRECTION ( 'NONE',  ( 0.9681751565707763518, -0.2502735827033140681, 0.000000000000000000 ) ) ;
#76128=VERTEX_POINT ( 'NONE', #68290 ) ;
#76129=ORIENTED_EDGE ( 'NONE', *, *, #60755, .T. ) ;
#76141=CARTESIAN_POINT ( 'NONE',  ( 49.04287251715432205, 95.72274150194785136, 10.00000000000000000 ) ) ;
#76146=EDGE_LOOP ( 'NONE', ( #75715, #21285, #70763, #46522 ) ) ;
#76161=CYLINDRICAL_SURFACE ( 'NONE', #91519, 70.00000000000002842 ) ;
#76167=ORIENTED_EDGE ( 'NONE', *, *, #28011, .T. ) ;
#76171=DIRECTION ( 'NONE',  ( -0.000000000000000000, -0.000000000000000000, -1.000000000000000000 ) ) ;
#76175=LINE ( 'NONE', #13371, #82314 ) ;
#76203=DIRECTION ( 'NONE',  ( -0.1860369090531061032, -0.9825427565607341984, 0.000000000000000000 ) ) ;
#76207=( LENGTH_UNIT ( ) NAMED_UNIT ( * ) SI_UNIT ( .MILLI., .METRE. ) );
#76209=CARTESIAN_POINT ( 'NONE',  ( -0.2492734796364602656, 27.10516647459198225, 10.00000000000000000 ) ) ;
#76213=LINE ( 'NONE', #44771, #84662 ) ;
#76218=VECTOR ( 'NONE', #30965, 1000.000000000000114 ) ;
#76223=FACE_OUTER_BOUND ( 'NONE', #2501, .T. ) ;
#76224=ORIENTED_EDGE ( 'NONE', *, *, #6148, .F. ) ;
#76226=DIRECTION ( 'NONE',  ( -0.4897629171537585258, 0.8718556560469402639, 0.000000000000000000 ) ) ;
#76243=VERTEX_POINT ( 'NONE', #13612 ) ;
#76248=ORIENTED_EDGE ( 'NONE', *, *, #6359, .T. ) ;
#76251=ADVANCED_FACE ( 'NONE', ( #6990 ), #83040, .T. ) ;
#76254=ORIENTED_EDGE ( 'NONE', *, *, #72268, .T. ) ;
#76267=VERTEX_POINT ( 'NONE', #60174 ) ;
#76281=ORIENTED_EDGE ( 'NONE', *, *, #57987, .F. ) ;
#76282=DIRECTION ( 'NONE',  ( -0.6303371332823576312, -0.7763215174174805666, 0.000000000000000000 ) ) ;
#76284=EDGE_CURVE ( 'NONE', #73229, #18285, #59168, .T. ) ;
#76287=CARTESIAN_POINT ( 'NONE',  ( -40.67952639183666008, 27.60432558407080350, 10.00000000000000000 ) ) ;
#76295=EDGE_CURVE ( 'NONE', #38684, #30963, #5015, .T. ) ;
#76297=ADVANCED_FACE ( 'NONE', ( #99212 ), #90142, .F. ) ;
#76302=CARTESIAN_POINT ( 'NONE',  ( 41.85954357502988898, 126.4744881464662001, 177.5919119679930134 ) ) ;
#76309=CARTESIAN_POINT ( 'NONE',  ( 48.73804053012794668, 107.9864336245683631, -10.00000000000000000 ) ) ;
#76333=PLANE ( 'NONE',  #86603 ) ;
#76337=VERTEX_POINT ( 'NONE', #44986 ) ;
#76340=EDGE_LOOP ( 'NONE', ( #11601, #95724, #44411, #74854 ) ) ;
#76344=CARTESIAN_POINT ( 'NONE',  ( -21.31413092498267048, 24.33771760303831755, -10.00000000000000000 ) ) ;
#76345=DIRECTION ( 'NONE',  ( -0.3402761906661271873, -0.9403255362191060840, 0.000000000000000000 ) ) ;
#76358=VERTEX_POINT ( 'NONE', #63693 ) ;
#76362=FACE_OUTER_BOUND ( 'NONE', #38680, .T. ) ;
#76368=EDGE_CURVE ( 'NONE', #30353, #68986, #47976, .T. ) ;
#76376=ORIENTED_EDGE ( 'NONE', *, *, #14781, .F. ) ;
#76384=ORIENTED_EDGE ( 'NONE', *, *, #33054, .T. ) ;
#76385=CARTESIAN_POINT ( 'NONE',  ( -36.56673362314461428, 37.64405826905806407, 59.99999999999999289 ) ) ;
#76387=CARTESIAN_POINT ( 'NONE',  ( -4.653128914090328472, 78.77562236714182120, 59.99999999999999289 ) ) ;
#76392=CARTESIAN_POINT ( 'NONE',  ( 15.77038241084232517, 34.14663330942826747, 10.00000000000000000 ) ) ;
#76401=EDGE_CURVE ( 'NONE', #91080, #61231, #77287, .T. ) ;
#76409=CARTESIAN_POINT ( 'NONE',  ( -75.18208942163933273, 50.44421862632484022, 177.5919119679930134 ) ) ;
#76416=EDGE_CURVE ( 'NONE', #87878, #8862, #43539, .T. ) ;
#76439=CARTESIAN_POINT ( 'NONE',  ( 7.225231395932167899, 28.43104314603600358, -10.00000000000000000 ) ) ;
#76447=ORIENTED_EDGE ( 'NONE', *, *, #70999, .T. ) ;
#76464=VERTEX_POINT ( 'NONE', #74965 ) ;
#76466=DIRECTION ( 'NONE',  ( -0.1550826972584531394, -0.9879014915521905360, 0.000000000000000000 ) ) ;
#76468=ORIENTED_EDGE ( 'NONE', *, *, #79784, .T. ) ;
#76474=CARTESIAN_POINT ( 'NONE',  ( -72.81784413424504976, 47.52919789448971244, -10.00000000000000000 ) ) ;
#76480=AXIS2_PLACEMENT_3D ( 'NONE', #78954, #100242, #1438 ) ;
#76487=CARTESIAN_POINT ( 'NONE',  ( 44.95821123098110661, 116.5722627105190270, -10.00000000000000000 ) ) ;
#76488=ORIENTED_EDGE ( 'NONE', *, *, #8360, .T. ) ;
#76495=LINE ( 'NONE', #38462, #20483 ) ;
#76499=VERTEX_POINT ( 'NONE', #7534 ) ;
#76506=ORIENTED_EDGE ( 'NONE', *, *, #87123, .F. ) ;
#76516=EDGE_CURVE ( 'NONE', #8092, #22139, #52626, .T. ) ;
#76524=EDGE_CURVE ( 'NONE', #79765, #3024, #14647, .T. ) ;
#76530=ADVANCED_FACE ( 'NONE', ( #56998 ), #25102, .T. ) ;
#76535=DIRECTION ( 'NONE',  ( 0.8599083858334038988, -0.5104483989331241034, 0.000000000000000000 ) ) ;
#76538=CARTESIAN_POINT ( 'NONE',  ( 13.18854085237251539, 31.24736827225017777, 10.00000000000000000 ) ) ;
#76555=DIRECTION ( 'NONE',  ( 0.000000000000000000, -0.000000000000000000, -1.000000000000000000 ) ) ;
#76556=EDGE_CURVE ( 'NONE', #24006, #8092, #26121, .T. ) ;
#76578=ORIENTED_EDGE ( 'NONE', *, *, #64377, .F. ) ;
#76584=FACE_OUTER_BOUND ( 'NONE', #59623, .T. ) ;
#76588=ORIENTED_EDGE ( 'NONE', *, *, #88569, .T. ) ;
#76593=CARTESIAN_POINT ( 'NONE',  ( -58.10760318826260118, 36.06970723555269842, -10.00000000000000000 ) ) ;
#76594=ORIENTED_EDGE ( 'NONE', *, *, #69077, .F. ) ;
#76596=CARTESIAN_POINT ( 'NONE',  ( -6.015783505528726316, 74.68510901943744784, 14.77481591981949016 ) ) ;
#76598=CARTESIAN_POINT ( 'NONE',  ( 48.74043828842092552, 100.0309547576005258, 10.00000000000000000 ) ) ;
#76600=ORIENTED_EDGE ( 'NONE', *, *, #94219, .F. ) ;
#76602=ORIENTED_EDGE ( 'NONE', *, *, #23058, .F. ) ;
#76607=DIRECTION ( 'NONE',  ( 1.000000000000000000, -4.369520618346150875E-13, 0.000000000000000000 ) ) ;
#76610=VECTOR ( 'NONE', #83220, 1000.000000000000000 ) ;
#76625=LINE ( 'NONE', #21431, #1380 ) ;
#76640=ORIENTED_EDGE ( 'NONE', *, *, #42382, .F. ) ;
#76644=LINE ( 'NONE', #92868, #2914 ) ;
#76650=CARTESIAN_POINT ( 'NONE',  ( 9.837252142675989575, 71.98620320469845524, 1.836970198720989751E-15 ) ) ;
#76654=ADVANCED_FACE ( 'NONE', ( #6302 ), #5314, .F. ) ;
#76659=CARTESIAN_POINT ( 'NONE',  ( 49.07419501245632176, 91.40403951869188859, 10.00000000000000000 ) ) ;
#76666=VERTEX_POINT ( 'NONE', #44290 ) ;
#76667=AXIS2_PLACEMENT_3D ( 'NONE', #14772, #68466, #99394 ) ;
#76679=LINE ( 'NONE', #6779, #8546 ) ;
#76681=VERTEX_POINT ( 'NONE', #43291 ) ;
#76683=DIRECTION ( 'NONE',  ( 1.000000000000000000, -6.145877457746401150E-15, 0.000000000000000000 ) ) ;
#76686=ORIENTED_EDGE ( 'NONE', *, *, #82448, .F. ) ;
#76688=DIRECTION ( 'NONE',  ( -0.1172721027424030449, -0.9930998207221544138, 0.000000000000000000 ) ) ;
#76691=CARTESIAN_POINT ( 'NONE',  ( 44.35815684012577265, 67.96982248125696913, -10.00000000000000000 ) ) ;
#76694=LINE ( 'NONE', #7287, #90781 ) ;
#76706=VERTEX_POINT ( 'NONE', #27627 ) ;
#76708=DIRECTION ( 'NONE',  ( 0.000000000000000000, 0.000000000000000000, 1.000000000000000000 ) ) ;
#76712=VERTEX_POINT ( 'NONE', #89466 ) ;
#76722=EDGE_CURVE ( 'NONE', #26122, #26501, #51400, .T. ) ;
#76731=DIRECTION ( 'NONE',  ( 0.1577859398657057155, -0.9874733399847793747, 0.000000000000000000 ) ) ;
#76738=CIRCLE ( 'NONE', #71914, 70.00000000000001421 ) ;
#76745=VECTOR ( 'NONE', #80774, 1000.000000000000114 ) ;
#76754=ORIENTED_EDGE ( 'NONE', *, *, #84524, .F. ) ;
#76783=DIRECTION ( 'NONE',  ( 0.000000000000000000, 0.000000000000000000, 1.000000000000000000 ) ) ;
#76798=EDGE_LOOP ( 'NONE', ( #10293, #297, #19089, #18442 ) ) ;
#76805=CARTESIAN_POINT ( 'NONE',  ( -73.83803415018344651, 50.74234351129840093, 10.00000000000000000 ) ) ;
#76808=DIRECTION ( 'NONE',  ( 0.4270171210482450741, -0.9042435392811321027, 0.000000000000000000 ) ) ;
#76809=ORIENTED_EDGE ( 'NONE', *, *, #43684, .F. ) ;
#76827=DIRECTION ( 'NONE',  ( 0.9681751565707763518, -0.2502735827033140681, 0.000000000000000000 ) ) ;
#76831=CARTESIAN_POINT ( 'NONE',  ( -19.77365603540006944, 93.13978744366448836, 59.99999999999999289 ) ) ;
#76832=DIRECTION ( 'NONE',  ( 0.06142469166373833167, 0.9981117208278915687, 0.000000000000000000 ) ) ;
#76833=DIRECTION ( 'NONE',  ( -0.9946578707245746775, -0.1032265479692855564, 0.000000000000000000 ) ) ;
#76846=VECTOR ( 'NONE', #24119, 1000.000000000000000 ) ;
#76848=CARTESIAN_POINT ( 'NONE',  ( 36.10619739613039769, 52.83927550304669296, 10.00000000000000000 ) ) ;
#76850=DIRECTION ( 'NONE',  ( 0.000000000000000000, 0.000000000000000000, 1.000000000000000000 ) ) ;
#76858=PLANE ( 'NONE',  #75354 ) ;
#76859=DIRECTION ( 'NONE',  ( 1.000000000000000000, 1.048764250047692355E-13, 0.000000000000000000 ) ) ;
#76860=ORIENTED_EDGE ( 'NONE', *, *, #32493, .F. ) ;
#76864=DIRECTION ( 'NONE',  ( -0.8903844177683322147, -0.4552093898365321412, 0.000000000000000000 ) ) ;
#76883=DIRECTION ( 'NONE',  ( -0.7561390817803280706, 0.6544109481086042290, 0.000000000000000000 ) ) ;
#76885=ADVANCED_FACE ( 'NONE', ( #76223 ), #92434, .T. ) ;
#76889=DIRECTION ( 'NONE',  ( -0.6386832404231509441, -0.7694697644498993405, 0.000000000000000000 ) ) ;
#76901=CARTESIAN_POINT ( 'NONE',  ( -9.693023484072631035, 23.77726266618847717, 177.5919119679930134 ) ) ;
#76909=CARTESIAN_POINT ( 'NONE',  ( -49.78034631855285141, 29.87998972566341749, 177.5919119679930134 ) ) ;
#76916=VECTOR ( 'NONE', #68148, 1000.000000000000114 ) ;
#76923=ORIENTED_EDGE ( 'NONE', *, *, #69056, .F. ) ;
#76935=AXIS2_PLACEMENT_3D ( 'NONE', #4552, #43544, #28343 ) ;
#76936=PLANE ( 'NONE',  #89386 ) ;
#76938=EDGE_CURVE ( 'NONE', #23598, #18450, #40985, .T. ) ;
#76941=CARTESIAN_POINT ( 'NONE',  ( 46.43574122514301195, 74.10519008736565638, -10.00000000000000000 ) ) ;
#76942=AXIS2_PLACEMENT_3D ( 'NONE', #2525, #18718, #95763 ) ;
#76944=EDGE_CURVE ( 'NONE', #52938, #12952, #38506, .T. ) ;
#76948=CARTESIAN_POINT ( 'NONE',  ( 47.66616421796181413, 112.2513067263565034, 10.00000000000000000 ) ) ;
#76953=EDGE_CURVE ( 'NONE', #45907, #14302, #88698, .T. ) ;
#76960=DIRECTION ( 'NONE',  ( -0.9681751565707790164, 0.2502735827033040761, 0.000000000000000000 ) ) ;
#76961=VERTEX_POINT ( 'NONE', #88675 ) ;
#76964=EDGE_CURVE ( 'NONE', #19465, #60481, #69255, .T. ) ;
#76970=DIRECTION ( 'NONE',  ( -0.5000000000000013323, 0.8660254037844380415, 0.000000000000000000 ) ) ;
#76974=VERTEX_POINT ( 'NONE', #3049 ) ;
#76975=ORIENTED_EDGE ( 'NONE', *, *, #16900, .T. ) ;
#76977=ORIENTED_EDGE ( 'NONE', *, *, #98597, .F. ) ;
#76978=CARTESIAN_POINT ( 'NONE',  ( -42.18065534595050536, 68.63081177882914119, -10.00000000000000000 ) ) ;
#76979=CARTESIAN_POINT ( 'NONE',  ( -28.04097607764120781, 24.82386083235215679, 10.00000000000000000 ) ) ;
#76980=AXIS2_PLACEMENT_3D ( 'NONE', #57164, #3503, #88145 ) ;
#76991=VERTEX_POINT ( 'NONE', #56711 ) ;
#76993=CARTESIAN_POINT ( 'NONE',  ( -19.65312891409030271, 93.06504152958497400, 10.00000000000000888 ) ) ;
#77002=VECTOR ( 'NONE', #36131, 1000.000000000000000 ) ;
#77008=LINE ( 'NONE', #52212, #30584 ) ;
#77016=EDGE_CURVE ( 'NONE', #4561, #23431, #81067, .T. ) ;
#77018=FACE_OUTER_BOUND ( 'NONE', #80874, .T. ) ;
#77029=EDGE_CURVE ( 'NONE', #861, #71916, #95769, .T. ) ;
#77036=DIRECTION ( 'NONE',  ( -1.000000000000000000, -4.892646582057397676E-14, 0.000000000000000000 ) ) ;
#77042=DIRECTION ( 'NONE',  ( -0.000000000000000000, 0.000000000000000000, -1.000000000000000000 ) ) ;
#77048=VECTOR ( 'NONE', #88137, 1000.000000000000000 ) ;
#77052=CARTESIAN_POINT ( 'NONE',  ( 48.29091023345864642, 82.53782597618220507, 10.00000000000000000 ) ) ;
#77055=ORIENTED_EDGE ( 'NONE', *, *, #35387, .F. ) ;
#77056=CARTESIAN_POINT ( 'NONE',  ( 32.06367262104295435, 91.81775857601540736, 59.99999999999999289 ) ) ;
#77058=AXIS2_PLACEMENT_3D ( 'NONE', #33508, #57288, #95853 ) ;
#77066=ORIENTED_EDGE ( 'NONE', *, *, #540, .T. ) ;
#77073=EDGE_CURVE ( 'NONE', #38281, #97061, #6005, .T. ) ;
#77075=ORIENTED_EDGE ( 'NONE', *, *, #37389, .T. ) ;
#77076=AXIS2_PLACEMENT_3D ( 'NONE', #44099, #68905, #5618 ) ;
#77078=EDGE_CURVE ( 'NONE', #31865, #98895, #66313, .T. ) ;
#77079=CIRCLE ( 'NONE', #43081, 0.1418229129681591871 ) ;
#77082=DIRECTION ( 'NONE',  ( -0.5895128895116622525, -0.8077589696806904973, 0.000000000000000000 ) ) ;
#77085=CARTESIAN_POINT ( 'NONE',  ( -16.46315656107408287, 74.30252503275481502, 13.46087100379897450 ) ) ;
#77089=VECTOR ( 'NONE', #71386, 1000.000000000000114 ) ;
#77091=VERTEX_POINT ( 'NONE', #83044 ) ;
#77102=DIRECTION ( 'NONE',  ( -0.7440200784635719877, -0.6681572590663519273, 0.000000000000000000 ) ) ;
#77108=CARTESIAN_POINT ( 'NONE',  ( 19.31801425620940194, 115.5650415295850451, 20.00000000000000355 ) ) ;
#77114=EDGE_LOOP ( 'NONE', ( #60847, #69726, #97671, #51945 ) ) ;
#77125=AXIS2_PLACEMENT_3D ( 'NONE', #97816, #5100, #59777 ) ;
#77127=AXIS2_PLACEMENT_3D ( 'NONE', #56761, #33991, #95823 ) ;
#77133=DIRECTION ( 'NONE',  ( -1.000000000000000000, 0.000000000000000000, -0.000000000000000000 ) ) ;
#77135=FACE_OUTER_BOUND ( 'NONE', #53991, .T. ) ;
#77136=DIRECTION ( 'NONE',  ( -0.5609510170580174204, -0.8278489937552475642, 0.000000000000000000 ) ) ;
#77140=CARTESIAN_POINT ( 'NONE',  ( 41.50249547274756878, 124.4848494355456836, 10.00000000000000000 ) ) ;
#77149=AXIS2_PLACEMENT_3D ( 'NONE', #65393, #73506, #4090 ) ;
#77158=EDGE_CURVE ( 'NONE', #43692, #15769, #12118, .T. ) ;
#77162=AXIS2_PLACEMENT_3D ( 'NONE', #24365, #55237, #94795 ) ;
#77174=DIRECTION ( 'NONE',  ( 1.000000000000000000, 3.548748596569695807E-14, 0.000000000000000000 ) ) ;
#77184=LINE ( 'NONE', #46262, #39578 ) ;
#77196=EDGE_LOOP ( 'NONE', ( #59639, #57051, #35632, #73598 ) ) ;
#77199=EDGE_CURVE ( 'NONE', #20907, #84697, #49815, .T. ) ;
#77201=DIRECTION ( 'NONE',  ( 0.8074371744834156761, 0.5899535653441194683, 0.000000000000000000 ) ) ;
#77207=VECTOR ( 'NONE', #96688, 1000.000000000000000 ) ;
#77210=LINE ( 'NONE', #23488, #47721 ) ;
#77211=ORIENTED_EDGE ( 'NONE', *, *, #19298, .F. ) ;
#77218=VERTEX_POINT ( 'NONE', #73920 ) ;
#77220=AXIS2_PLACEMENT_3D ( 'NONE', #26796, #81050, #26304 ) ;
#77225=PLANE ( 'NONE',  #70630 ) ;
#77230=VERTEX_POINT ( 'NONE', #13617 ) ;
#77236=EDGE_CURVE ( 'NONE', #31865, #70938, #44490, .T. ) ;
#77242=DIRECTION ( 'NONE',  ( 0.1473778574936430164, 0.9890802632347809320, 0.000000000000000000 ) ) ;
#77243=LINE ( 'NONE', #69635, #79117 ) ;
#77248=DIRECTION ( 'NONE',  ( -0.8393827800519415572, -0.5435407515102007592, 0.000000000000000000 ) ) ;
#77261=DIRECTION ( 'NONE',  ( -0.8450603975019854719, 0.5346708562973919721, 0.000000000000000000 ) ) ;
#77267=ORIENTED_EDGE ( 'NONE', *, *, #83014, .F. ) ;
#77269=DIRECTION ( 'NONE',  ( -0.5000000000000013323, 0.8660254037844380415, 0.000000000000000000 ) ) ;
#77272=VECTOR ( 'NONE', #99861, 999.9999999999998863 ) ;
#77283=DIRECTION ( 'NONE',  ( 0.8080546441192343332, -0.5891075386695857619, 0.000000000000000000 ) ) ;
#77287=CIRCLE ( 'NONE', #74050, 70.00000000000001421 ) ;
#77300=CARTESIAN_POINT ( 'NONE',  ( -19.65312891409030271, 93.06504152958497400, 10.00000000000000888 ) ) ;
#77302=DIRECTION ( 'NONE',  ( -1.000000000000000000, 0.000000000000000000, 0.000000000000000000 ) ) ;
#77304=ORIENTED_EDGE ( 'NONE', *, *, #5915, .F. ) ;
#77311=CARTESIAN_POINT ( 'NONE',  ( 30.13368333964083590, 79.01311634467327849, 59.99999999999999289 ) ) ;
#77321=ORIENTED_EDGE ( 'NONE', *, *, #44572, .T. ) ;
#77329=DIRECTION ( 'NONE',  ( 0.000000000000000000, 0.000000000000000000, 1.000000000000000000 ) ) ;
#77330=DIRECTION ( 'NONE',  ( -0.000000000000000000, -0.000000000000000000, -1.000000000000000000 ) ) ;
#77343=CYLINDRICAL_SURFACE ( 'NONE', #78819, 70.00000000000002842 ) ;
#77345=AXIS2_PLACEMENT_3D ( 'NONE', #88962, #66084, #51883 ) ;
#77354=VECTOR ( 'NONE', #39603, 1000.000000000000000 ) ;
#77355=EDGE_CURVE ( 'NONE', #72111, #41570, #57909, .T. ) ;
#77357=AXIS2_PLACEMENT_3D ( 'NONE', #90971, #37701, #28618 ) ;
#77358=VERTEX_POINT ( 'NONE', #26206 ) ;
#77367=CARTESIAN_POINT ( 'NONE',  ( 50.18541494347880416, 88.31343213334855591, 177.5919119679930134 ) ) ;
#77372=LINE ( 'NONE', #60147, #18794 ) ;
#77373=EDGE_LOOP ( 'NONE', ( #37849, #84106, #58859, #92120 ) ) ;
#77379=CARTESIAN_POINT ( 'NONE',  ( -13.12676960854360786, 60.47780990635891385, -10.00000000000000000 ) ) ;
#77384=VERTEX_POINT ( 'NONE', #56592 ) ;
#77404=VECTOR ( 'NONE', #90779, 1000.000000000000114 ) ;
#77413=EDGE_CURVE ( 'NONE', #15552, #77091, #95658, .T. ) ;
#77420=EDGE_CURVE ( 'NONE', #55128, #69980, #8383, .T. ) ;
#77424=VECTOR ( 'NONE', #53824, 1000.000000000000114 ) ;
#77427=LINE ( 'NONE', #69803, #84649 ) ;
#77428=AXIS2_PLACEMENT_3D ( 'NONE', #55396, #39193, #25012 ) ;
#77447=EDGE_LOOP ( 'NONE', ( #96961, #7087, #99028, #24008 ) ) ;
#77450=VERTEX_POINT ( 'NONE', #39250 ) ;
#77456=ORIENTED_EDGE ( 'NONE', *, *, #50746, .T. ) ;
#77459=DIRECTION ( 'NONE',  ( 1.000000000000000000, 0.000000000000000000, 0.000000000000000000 ) ) ;
#77461=ORIENTED_EDGE ( 'NONE', *, *, #32593, .F. ) ;
#77465=FACE_OUTER_BOUND ( 'NONE', #72222, .T. ) ;
#77487=CARTESIAN_POINT ( 'NONE',  ( -50.41871976035449165, 31.58591985673634639, -10.00000000000000000 ) ) ;
#77488=EDGE_LOOP ( 'NONE', ( #40397, #38919, #23718, #68879 ) ) ;
#77493=LINE ( 'NONE', #69867, #66071 ) ;
#77506=CIRCLE ( 'NONE', #59449, 70.00000000000001421 ) ;
#77510=DIRECTION ( 'NONE',  ( 0.000000000000000000, 0.000000000000000000, 1.000000000000000000 ) ) ;
#77511=AXIS2_PLACEMENT_3D ( 'NONE', #43353, #13964, #97592 ) ;
#77512=ORIENTED_EDGE ( 'NONE', *, *, #86226, .F. ) ;
#77523=DIRECTION ( 'NONE',  ( 0.9681751565707763518, -0.2502735827033140681, 0.000000000000000000 ) ) ;
#77526=CARTESIAN_POINT ( 'NONE',  ( -27.23710841895085721, 23.47708815495369450, 177.5919119679930134 ) ) ;
#77537=DIRECTION ( 'NONE',  ( 1.000000000000000000, -3.152240373489283172E-13, 0.000000000000000000 ) ) ;
#77541=EDGE_LOOP ( 'NONE', ( #75723, #18458, #56787, #13482 ) ) ;
#77542=EDGE_CURVE ( 'NONE', #77961, #93808, #97024, .T. ) ;
#77543=EDGE_CURVE ( 'NONE', #84457, #33337, #82330, .T. ) ;
#77562=CARTESIAN_POINT ( 'NONE',  ( 49.06003799288187395, 95.45573527953635562, 10.00000000000000000 ) ) ;
#77565=PLANE ( 'NONE',  #74189 ) ;
#77574=ORIENTED_EDGE ( 'NONE', *, *, #11962, .T. ) ;
#77579=CARTESIAN_POINT ( 'NONE',  ( -56.06787742410712383, 34.75406423768147590, 10.00000000000000000 ) ) ;
#77592=VERTEX_POINT ( 'NONE', #89432 ) ;
#77602=ORIENTED_EDGE ( 'NONE', *, *, #36924, .F. ) ;
#77610=VERTEX_POINT ( 'NONE', #13866 ) ;
#77615=VERTEX_POINT ( 'NONE', #77684 ) ;
#77616=ORIENTED_EDGE ( 'NONE', *, *, #23058, .T. ) ;
#77618=CARTESIAN_POINT ( 'NONE',  ( 5.783292089056025098, 27.85010085989871698, 177.5919119679930134 ) ) ;
#77643=ORIENTED_EDGE ( 'NONE', *, *, #81244, .T. ) ;
#77649=VECTOR ( 'NONE', #66262, 1000.000000000000000 ) ;
#77652=DIRECTION ( 'NONE',  ( -0.3668518372888710521, -0.9302793824855948301, 0.000000000000000000 ) ) ;
#77673=EDGE_CURVE ( 'NONE', #52913, #48736, #93902, .T. ) ;
#77678=DIRECTION ( 'NONE',  ( -0.9762722099447411761, -0.2165469281463284212, 0.000000000000000000 ) ) ;
#77684=CARTESIAN_POINT ( 'NONE',  ( 32.18695666311190706, 46.02670049433633181, -10.00000000000000000 ) ) ;
#77704=CARTESIAN_POINT ( 'NONE',  ( 24.35067441160642687, 40.23626134430271861, -10.00000000000000000 ) ) ;
#77728=LINE ( 'NONE', #95471, #50982 ) ;
#77730=ORIENTED_EDGE ( 'NONE', *, *, #85069, .T. ) ;
#77734=ORIENTED_EDGE ( 'NONE', *, *, #83156, .F. ) ;
#77737=ORIENTED_EDGE ( 'NONE', *, *, #98923, .F. ) ;
#77755=FACE_OUTER_BOUND ( 'NONE', #83338, .T. ) ;
#77758=LINE ( 'NONE', #8341, #17617 ) ;
#77763=DIRECTION ( 'NONE',  ( -0.000000000000000000, 0.000000000000000000, -1.000000000000000000 ) ) ;
#77778=LINE ( 'NONE', #54429, #64772 ) ;
#77780=DIRECTION ( 'NONE',  ( -0.000000000000000000, -0.000000000000000000, -1.000000000000000000 ) ) ;
#77793=LINE ( 'NONE', #78788, #1459 ) ;
#77797=EDGE_CURVE ( 'NONE', #78204, #166, #64725, .T. ) ;
#77806=CIRCLE ( 'NONE', #30854, 70.00000000000001421 ) ;
#77807=DIRECTION ( 'NONE',  ( -0.8916269620120497175, 0.4527707594502572430, 0.000000000000000000 ) ) ;
#77811=DIRECTION ( 'NONE',  ( -0.8614378286617615510, 0.5078630399532039208, 0.000000000000000000 ) ) ;
#77837=EDGE_LOOP ( 'NONE', ( #67969, #5681, #4962, #15017 ) ) ;
#77839=DIRECTION ( 'NONE',  ( -0.9879428538673719062, -0.1548189829846212673, 0.000000000000000000 ) ) ;
#77842=FACE_OUTER_BOUND ( 'NONE', #96828, .T. ) ;
#77851=VERTEX_POINT ( 'NONE', #2435 ) ;
#77867=ORIENTED_EDGE ( 'NONE', *, *, #41272, .T. ) ;
#77876=CARTESIAN_POINT ( 'NONE',  ( -50.41871976035449165, 31.58591985673634639, 10.00000000000000000 ) ) ;
#77894=LINE ( 'NONE', #61665, #51336 ) ;
#77896=DIRECTION ( 'NONE',  ( -1.000000000000000000, 0.000000000000000000, 0.000000000000000000 ) ) ;
#77902=DIRECTION ( 'NONE',  ( 0.9213551052231946370, -0.3887219701523905724, 0.000000000000000000 ) ) ;
#77903=EDGE_CURVE ( 'NONE', #14650, #5695, #20834, .T. ) ;
#77924=LINE ( 'NONE', #44123, #6404 ) ;
#77926=ADVANCED_FACE ( 'NONE', ( #71837 ), #57599, .F. ) ;
#77927=DIRECTION ( 'NONE',  ( -0.000000000000000000, 0.000000000000000000, 1.000000000000000000 ) ) ;
#77938=VECTOR ( 'NONE', #99857, 999.9999999999998863 ) ;
#77951=ORIENTED_EDGE ( 'NONE', *, *, #9867, .T. ) ;
#77956=PLANE ( 'NONE',  #69281 ) ;
#77961=VERTEX_POINT ( 'NONE', #56611 ) ;
#77977=ORIENTED_EDGE ( 'NONE', *, *, #52200, .T. ) ;
#77984=ORIENTED_EDGE ( 'NONE', *, *, #17117, .F. ) ;
#77986=DIRECTION ( 'NONE',  ( -0.6363689690731114679, -0.7713848165480218233, 0.000000000000000000 ) ) ;
#77989=CARTESIAN_POINT ( 'NONE',  ( 40.34888600819125060, 126.6204015641749834, -10.00000000000000000 ) ) ;
#77992=CARTESIAN_POINT ( 'NONE',  ( -21.31413092498266693, 24.33771760303832465, -10.00000000000000000 ) ) ;
#77994=ORIENTED_EDGE ( 'NONE', *, *, #56591, .F. ) ;
#77995=EDGE_CURVE ( 'NONE', #51013, #2862, #97155, .T. ) ;
#77997=EDGE_CURVE ( 'NONE', #49393, #71997, #75827, .T. ) ;
#77998=ORIENTED_EDGE ( 'NONE', *, *, #36213, .F. ) ;
#78005=ORIENTED_EDGE ( 'NONE', *, *, #93241, .T. ) ;
#78010=SHAPE_REPRESENTATION ( 'Middle Movable Base', ( #68784 ), #81782 ) ;
#78017=FACE_OUTER_BOUND ( 'NONE', #11568, .T. ) ;
#78030=CARTESIAN_POINT ( 'NONE',  ( -19.65312891409030271, 93.06504152958497400, 10.00000000000000888 ) ) ;
#78042=EDGE_CURVE ( 'NONE', #4283, #8200, #7389, .T. ) ;
#78054=CARTESIAN_POINT ( 'NONE',  ( -19.65312891409030271, 93.06504152958497400, 20.00000000000000355 ) ) ;
#78062=VECTOR ( 'NONE', #68018, 1000.000000000000000 ) ;
#78081=ORIENTED_EDGE ( 'NONE', *, *, #211, .F. ) ;
#78082=ORIENTED_EDGE ( 'NONE', *, *, #21384, .T. ) ;
#78091=DIRECTION ( 'NONE',  ( 0.9458118053197297481, -0.3247153044096220409, 0.000000000000000000 ) ) ;
#78101=EDGE_LOOP ( 'NONE', ( #3439, #3004, #81967, #4478 ) ) ;
#78102=CARTESIAN_POINT ( 'NONE',  ( -15.49391466533604067, 73.38841914279046819, 13.64384121658392246 ) ) ;
#78114=DIRECTION ( 'NONE',  ( -0.000000000000000000, -0.000000000000000000, -1.000000000000000000 ) ) ;
#78119=AXIS2_PLACEMENT_3D ( 'NONE', #64091, #41781, #9909 ) ;
#78123=LINE ( 'NONE', #39580, #36377 ) ;
#78142=VECTOR ( 'NONE', #17649, 1000.000000000000000 ) ;
#78148=ORIENTED_EDGE ( 'NONE', *, *, #35203, .T. ) ;
#78151=CYLINDRICAL_SURFACE ( 'NONE', #36863, 70.00000000000002842 ) ;
#78155=LINE ( 'NONE', #1150, #90016 ) ;
#78166=DIRECTION ( 'NONE',  ( -0.6855440362341554961, 0.7280311630581363103, 0.000000000000000000 ) ) ;
#78172=DIRECTION ( 'NONE',  ( 0.000000000000000000, -0.000000000000000000, 1.000000000000000000 ) ) ;
#78173=DIRECTION ( 'NONE',  ( -0.8769651246872975925, 0.4805540241036304616, 0.000000000000000000 ) ) ;
#78175=ORIENTED_EDGE ( 'NONE', *, *, #15891, .T. ) ;
#78183=ADVANCED_FACE ( 'NONE', ( #84932 ), #30197, .T. ) ;
#78191=CARTESIAN_POINT ( 'NONE',  ( -59.87889494062799400, 37.30571521936384016, 10.00000000000000000 ) ) ;
#78193=CARTESIAN_POINT ( 'NONE',  ( -27.23710841895085011, 23.47708815495369450, -10.00000000000000000 ) ) ;
#78203=ORIENTED_EDGE ( 'NONE', *, *, #78563, .T. ) ;
#78204=VERTEX_POINT ( 'NONE', #34204 ) ;
#78206=VECTOR ( 'NONE', #9401, 1000.000000000000114 ) ;
#78209=PLANE ( 'NONE',  #20823 ) ;
#78222=DIRECTION ( 'NONE',  ( 1.000000000000000000, -7.930164461608259651E-15, 0.000000000000000000 ) ) ;
#78225=EDGE_CURVE ( 'NONE', #66499, #28990, #72220, .T. ) ;
#78227=ORIENTED_EDGE ( 'NONE', *, *, #6967, .F. ) ;
#78230=VERTEX_POINT ( 'NONE', #44767 ) ;
#78232=ORIENTED_EDGE ( 'NONE', *, *, #6359, .F. ) ;
#78238=EDGE_CURVE ( 'NONE', #34378, #46023, #96538, .T. ) ;
#78249=ADVANCED_FACE ( 'NONE', ( #83323 ), #28088, .F. ) ;
#78257=DIRECTION ( 'NONE',  ( -0.6444573283589029034, 0.7646402761589956576, 0.000000000000000000 ) ) ;
#78258=DIRECTION ( 'NONE',  ( 0.9008877160804890094, 0.4340522123146939859, 0.000000000000000000 ) ) ;
#78261=DIRECTION ( 'NONE',  ( -0.9778746070300391446, 0.2091919045418505763, 0.000000000000000000 ) ) ;
#78268=ORIENTED_EDGE ( 'NONE', *, *, #26705, .T. ) ;
#78272=CIRCLE ( 'NONE', #55599, 49.99999999999999289 ) ;
#78280=AXIS2_PLACEMENT_3D ( 'NONE', #58725, #90699, #89700 ) ;
#78287=CARTESIAN_POINT ( 'NONE',  ( -34.06669189922481422, 36.18719137533145158, 59.99999999999999289 ) ) ;
#78296=ORIENTED_EDGE ( 'NONE', *, *, #11455, .F. ) ;
#78304=ADVANCED_FACE ( 'NONE', ( #85850 ), #30080, .F. ) ;
#78313=CARTESIAN_POINT ( 'NONE',  ( 45.66470909604093720, 114.5311720768849995, 10.00000000000000000 ) ) ;
#78319=ORIENTED_EDGE ( 'NONE', *, *, #3505, .F. ) ;
#78320=EDGE_CURVE ( 'NONE', #91318, #78857, #22482, .T. ) ;
#78326=ORIENTED_EDGE ( 'NONE', *, *, #57873, .F. ) ;
#78343=ORIENTED_EDGE ( 'NONE', *, *, #53512, .F. ) ;
#78348=VECTOR ( 'NONE', #15075, 1000.000000000000114 ) ;
#78353=EDGE_CURVE ( 'NONE', #27025, #95233, #61470, .T. ) ;
#78360=LINE ( 'NONE', #72779, #74406 ) ;
#78372=DIRECTION ( 'NONE',  ( -0.8143688203140632131, 0.5803476755362092510, 0.000000000000000000 ) ) ;
#78390=CARTESIAN_POINT ( 'NONE',  ( 17.38248943320504836, 35.13769309531819829, -10.00000000000000000 ) ) ;
#78391=ORIENTED_EDGE ( 'NONE', *, *, #20877, .T. ) ;
#78395=DIRECTION ( 'NONE',  ( 0.000000000000000000, -0.000000000000000000, 1.000000000000000000 ) ) ;
#78418=CARTESIAN_POINT ( 'NONE',  ( -15.10528209597770299, 24.46087392797018722, -10.00000000000000000 ) ) ;
#78419=CIRCLE ( 'NONE', #33137, 70.00000000000001421 ) ;
#78424=CARTESIAN_POINT ( 'NONE',  ( 3.854092266844447501, 28.45370138451378850, -10.00000000000000000 ) ) ;
#78430=DIRECTION ( 'NONE',  ( -0.000000000000000000, -0.000000000000000000, -1.000000000000000000 ) ) ;
#78448=ORIENTED_EDGE ( 'NONE', *, *, #24112, .F. ) ;
#78455=ORIENTED_EDGE ( 'NONE', *, *, #42236, .F. ) ;
#78468=CYLINDRICAL_SURFACE ( 'NONE', #9328, 70.00000000000002842 ) ;
#78472=EDGE_CURVE ( 'NONE', #77592, #35956, #97392, .T. ) ;
#78482=VERTEX_POINT ( 'NONE', #59851 ) ;
#78484=LINE ( 'NONE', #24270, #67401 ) ;
#78486=ORIENTED_EDGE ( 'NONE', *, *, #81005, .F. ) ;
#78492=FACE_OUTER_BOUND ( 'NONE', #64576, .T. ) ;
#78499=CIRCLE ( 'NONE', #7310, 0.1418229129680793899 ) ;
#78503=ORIENTED_EDGE ( 'NONE', *, *, #64828, .F. ) ;
#78509=ORIENTED_EDGE ( 'NONE', *, *, #34398, .F. ) ;
#78516=EDGE_CURVE ( 'NONE', #5086, #14650, #51777, .T. ) ;
#78519=PLANE ( 'NONE',  #4099 ) ;
#78521=CARTESIAN_POINT ( 'NONE',  ( 19.31801425620940194, 115.5650415295850451, -45.00000000000001421 ) ) ;
#78528=VECTOR ( 'NONE', #90996, 1000.000000000000000 ) ;
#78554=EDGE_CURVE ( 'NONE', #95622, #3742, #23340, .T. ) ;
#78556=DIRECTION ( 'NONE',  ( -0.000000000000000000, 0.000000000000000000, -1.000000000000000000 ) ) ;
#78559=CARTESIAN_POINT ( 'NONE',  ( 30.62489312496363425, 46.16797101519271962, 10.00000000000000000 ) ) ;
#78563=EDGE_CURVE ( 'NONE', #43174, #6804, #40170, .T. ) ;
#78581=CARTESIAN_POINT ( 'NONE',  ( 38.70287833452073301, 99.18198963270081947, 59.99999999999999289 ) ) ;
#78582=ORIENTED_EDGE ( 'NONE', *, *, #27275, .T. ) ;
#78589=ORIENTED_EDGE ( 'NONE', *, *, #3104, .T. ) ;
#78590=LINE ( 'NONE', #95334, #34188 ) ;
#78596=CARTESIAN_POINT ( 'NONE',  ( 47.92671612011951510, 80.40884667711614497, -10.00000000000000000 ) ) ;
#78601=LINE ( 'NONE', #9187, #57489 ) ;
#78609=DIRECTION ( 'NONE',  ( 0.000000000000000000, -0.000000000000000000, -1.000000000000000000 ) ) ;
#78610=DIRECTION ( 'NONE',  ( -0.7646402761590023189, -0.6444573283588951318, 0.000000000000000000 ) ) ;
#78611=VECTOR ( 'NONE', #477, 1000.000000000000000 ) ;
#78614=LINE ( 'NONE', #69983, #25381 ) ;
#78615=DIRECTION ( 'NONE',  ( 0.000000000000000000, -0.000000000000000000, 1.000000000000000000 ) ) ;
#78631=AXIS2_PLACEMENT_3D ( 'NONE', #99454, #59416, #82794 ) ;
#78634=DIRECTION ( 'NONE',  ( 1.000000000000000000, 0.000000000000000000, 0.000000000000000000 ) ) ;
#78635=CARTESIAN_POINT ( 'NONE',  ( 26.18314342202568668, 41.82794442100486521, -10.00000000000000000 ) ) ;
#78654=DIRECTION ( 'NONE',  ( -0.8606332181800099290, 0.5092253565614338617, 0.000000000000000000 ) ) ;
#78662=ORIENTED_EDGE ( 'NONE', *, *, #47231, .T. ) ;
#78669=VECTOR ( 'NONE', #54289, 1000.000000000000114 ) ;
#78671=PLANE ( 'NONE',  #75039 ) ;
#78678=ORIENTED_EDGE ( 'NONE', *, *, #40432, .T. ) ;
#78689=CARTESIAN_POINT ( 'NONE',  ( 48.77433535142597520, 99.76555324011610537, -10.00000000000000000 ) ) ;
#78693=VERTEX_POINT ( 'NONE', #62116 ) ;
#78701=VECTOR ( 'NONE', #53457, 1000.000000000000114 ) ;
#78704=VECTOR ( 'NONE', #71605, 1000.000000000000000 ) ;
#78707=CARTESIAN_POINT ( 'NONE',  ( -61.39381520214497101, 38.43978098112751951, -10.00000000000000000 ) ) ;
#78708=EDGE_LOOP ( 'NONE', ( #99122, #9606, #8723, #20958 ) ) ;
#78709=VERTEX_POINT ( 'NONE', #7953 ) ;
#78710=DIRECTION ( 'NONE',  ( -0.9981280818701456781, -0.06115825522547174015, 0.000000000000000000 ) ) ;
#78712=ORIENTED_EDGE ( 'NONE', *, *, #20158, .T. ) ;
#78721=LINE ( 'NONE', #29247, #22324 ) ;
#78729=ORIENTED_EDGE ( 'NONE', *, *, #93807, .F. ) ;
#78730=CARTESIAN_POINT ( 'NONE',  ( 45.80758703142363686, 72.03864405183792030, 10.00000000000000000 ) ) ;
#78736=CARTESIAN_POINT ( 'NONE',  ( -76.38857681351474582, 54.22815603855766398, -10.00000000000000000 ) ) ;
#78738=ORIENTED_EDGE ( 'NONE', *, *, #70332, .T. ) ;
#78742=VECTOR ( 'NONE', #12328, 1000.000000000000000 ) ;
#78749=DIRECTION ( 'NONE',  ( -0.2471055264905585858, 0.9689885751534038638, 0.000000000000000000 ) ) ;
#78763=PLANE ( 'NONE',  #32526 ) ;
#78769=ORIENTED_EDGE ( 'NONE', *, *, #12930, .T. ) ;
#78775=AXIS2_PLACEMENT_3D ( 'NONE', #11608, #58664, #28781 ) ;
#78779=CARTESIAN_POINT ( 'NONE',  ( 48.95103868752454446, 97.61288834769685252, 10.00000000000000000 ) ) ;
#78788=CARTESIAN_POINT ( 'NONE',  ( 49.09245556086620610, 93.56363653685789927, 10.00000000000000000 ) ) ;
#78792=ADVANCED_FACE ( 'NONE', ( #18055 ), #71762, .F. ) ;
#78793=EDGE_CURVE ( 'NONE', #48146, #70901, #25653, .T. ) ;
#78805=CARTESIAN_POINT ( 'NONE',  ( -41.62359735524142934, 26.60228115600143184, -10.00000000000000000 ) ) ;
#78813=DIRECTION ( 'NONE',  ( -0.9414334852479556703, -0.3371987438498062484, 0.000000000000000000 ) ) ;
#78816=ORIENTED_EDGE ( 'NONE', *, *, #73080, .T. ) ;
#78817=DIRECTION ( 'NONE',  ( -0.8143688203140567738, 0.5803476755362181327, 0.000000000000000000 ) ) ;
#78819=AXIS2_PLACEMENT_3D ( 'NONE', #15518, #17535, #71257 ) ;
#78821=EDGE_CURVE ( 'NONE', #51318, #95480, #54264, .T. ) ;
#78829=CIRCLE ( 'NONE', #86976, 0.1418229129680828593 ) ;
#78830=EDGE_LOOP ( 'NONE', ( #25690, #81454, #14082, #30018 ) ) ;
#78836=LINE ( 'NONE', #24113, #49951 ) ;
#78837=CARTESIAN_POINT ( 'NONE',  ( -28.78056054657192320, 23.66266410781089391, 10.00000000000000000 ) ) ;
#78843=CARTESIAN_POINT ( 'NONE',  ( -19.65312891409030271, 93.06504152958497400, 60.00000000000000000 ) ) ;
#78849=ORIENTED_EDGE ( 'NONE', *, *, #39203, .T. ) ;
#78852=EDGE_LOOP ( 'NONE', ( #10533, #19300, #35729, #51705 ) ) ;
#78854=VERTEX_POINT ( 'NONE', #61872 ) ;
#78855=CARTESIAN_POINT ( 'NONE',  ( 30.65561236560288805, 105.1146769143126960, 59.99999999999999289 ) ) ;
#78856=FACE_OUTER_BOUND ( 'NONE', #29973, .T. ) ;
#78857=VERTEX_POINT ( 'NONE', #69488 ) ;
#78858=AXIS2_PLACEMENT_3D ( 'NONE', #91921, #22477, #45754 ) ;
#78877=EDGE_CURVE ( 'NONE', #26239, #39540, #62886, .T. ) ;
#78880=DIRECTION ( 'NONE',  ( -0.000000000000000000, -0.000000000000000000, -1.000000000000000000 ) ) ;
#78889=CARTESIAN_POINT ( 'NONE',  ( -40.42249077443060656, 27.53003111760058275, -10.00000000000000000 ) ) ;
#78894=CIRCLE ( 'NONE', #35185, 70.00000000000001421 ) ;
#78906=ADVANCED_FACE ( 'NONE', ( #102 ), #91833, .F. ) ;
#78917=CARTESIAN_POINT ( 'NONE',  ( -19.65312891409030271, 93.06504152958497400, 177.5919119679930134 ) ) ;
#78927=EDGE_CURVE ( 'NONE', #94071, #58717, #90854, .T. ) ;
#78928=PLANE ( 'NONE',  #65319 ) ;
#78932=ADVANCED_FACE ( 'NONE', ( #75609 ), #29497, .T. ) ;
#78934=CIRCLE ( 'NONE', #35232, 70.00000000000001421 ) ;
#78939=EDGE_CURVE ( 'NONE', #72976, #59430, #99908, .T. ) ;
#78948=VERTEX_POINT ( 'NONE', #30986 ) ;
#78951=DIRECTION ( 'NONE',  ( -0.8452030915256549815, -0.5344452582589497291, 0.000000000000000000 ) ) ;
#78954=CARTESIAN_POINT ( 'NONE',  ( -19.65312891409030271, 93.06504152958497400, 10.00000000000000888 ) ) ;
#78956=EDGE_CURVE ( 'NONE', #74106, #87650, #46686, .T. ) ;
#78957=FACE_OUTER_BOUND ( 'NONE', #13435, .T. ) ;
#78962=EDGE_LOOP ( 'NONE', ( #83233, #85307, #50500, #48927 ) ) ;
#78964=AXIS2_PLACEMENT_3D ( 'NONE', #78054, #71957, #94280 ) ;
#78966=VERTEX_POINT ( 'NONE', #61382 ) ;
#78971=FACE_OUTER_BOUND ( 'NONE', #18042, .T. ) ;
#78972=VERTEX_POINT ( 'NONE', #92336 ) ;
#78976=CIRCLE ( 'NONE', #14220, 0.1418229129684228651 ) ;
#78977=VERTEX_POINT ( 'NONE', #22884 ) ;
#78982=ORIENTED_EDGE ( 'NONE', *, *, #59685, .F. ) ;
#78983=DIRECTION ( 'NONE',  ( 0.000000000000000000, 0.000000000000000000, -1.000000000000000000 ) ) ;
#78986=ORIENTED_EDGE ( 'NONE', *, *, #75842, .F. ) ;
#78988=AXIS2_PLACEMENT_3D ( 'NONE', #2930, #80955, #64707 ) ;
#78991=DIRECTION ( 'NONE',  ( 0.000000000000000000, 0.000000000000000000, 1.000000000000000000 ) ) ;
#78995=CARTESIAN_POINT ( 'NONE',  ( 46.50192534792603283, 74.36443251879779837, -10.00000000000000000 ) ) ;
#78996=VECTOR ( 'NONE', #1229, 1000.000000000000114 ) ;
#79001=DIRECTION ( 'NONE',  ( 0.02225111142181396273, 0.9997524133706774396, 0.000000000000000000 ) ) ;
#79002=ORIENTED_EDGE ( 'NONE', *, *, #35552, .T. ) ;
#79004=ORIENTED_EDGE ( 'NONE', *, *, #67209, .F. ) ;
#79007=FACE_OUTER_BOUND ( 'NONE', #53654, .T. ) ;
#79013=ORIENTED_EDGE ( 'NONE', *, *, #24549, .T. ) ;
#79022=DIRECTION ( 'NONE',  ( -0.6303371332823575202, -0.7763215174174804556, 0.000000000000000000 ) ) ;
#79034=CYLINDRICAL_SURFACE ( 'NONE', #2528, 70.00000000000002842 ) ;
#79037=AXIS2_PLACEMENT_3D ( 'NONE', #41880, #19614, #11997 ) ;
#79042=VERTEX_POINT ( 'NONE', #87276 ) ;
#79043=AXIS2_PLACEMENT_3D ( 'NONE', #3082, #74473, #87725 ) ;
#79044=CIRCLE ( 'NONE', #17545, 70.00000000000001421 ) ;
#79054=DIRECTION ( 'NONE',  ( 0.000000000000000000, 0.000000000000000000, 1.000000000000000000 ) ) ;
#79059=EDGE_CURVE ( 'NONE', #24573, #94007, #49206, .T. ) ;
#79077=EDGE_CURVE ( 'NONE', #52870, #54113, #8694, .T. ) ;
#79088=CYLINDRICAL_SURFACE ( 'NONE', #36855, 70.00000000000002842 ) ;
#79102=DIRECTION ( 'NONE',  ( -0.009162850352621045372, 0.9999580202055561307, 0.000000000000000000 ) ) ;
#79103=ORIENTED_EDGE ( 'NONE', *, *, #85291, .T. ) ;
#79107=CARTESIAN_POINT ( 'NONE',  ( 35.43817338645654758, 49.87999306568067226, 177.5919119679930134 ) ) ;
#79115=ORIENTED_EDGE ( 'NONE', *, *, #65948, .T. ) ;
#79117=VECTOR ( 'NONE', #54414, 1000.000000000000114 ) ;
#79124=VECTOR ( 'NONE', #62290, 1000.000000000000000 ) ;
#79130=ORIENTED_EDGE ( 'NONE', *, *, #24972, .T. ) ;
#79144=LINE ( 'NONE', #72013, #57737 ) ;
#79150=EDGE_CURVE ( 'NONE', #57256, #74347, #26403, .T. ) ;
#79153=VECTOR ( 'NONE', #33947, 1000.000000000000227 ) ;
#79157=CARTESIAN_POINT ( 'NONE',  ( -19.65312891409030271, 93.06504152958497400, 10.00000000000000888 ) ) ;
#79159=ORIENTED_EDGE ( 'NONE', *, *, #39427, .F. ) ;
#79162=DIRECTION ( 'NONE',  ( 0.5011331959107180323, 0.8653701635463924013, 0.000000000000000000 ) ) ;
#79163=EDGE_CURVE ( 'NONE', #90523, #72718, #65881, .T. ) ;
#79183=CARTESIAN_POINT ( 'NONE',  ( 41.50249547274756878, 124.4848494355456836, -10.00000000000000000 ) ) ;
#79194=AXIS2_PLACEMENT_3D ( 'NONE', #40182, #76708, #84845 ) ;
#79200=CARTESIAN_POINT ( 'NONE',  ( 44.44706364856357084, 64.93738052781135650, 10.00000000000000000 ) ) ;
#79208=LINE ( 'NONE', #33058, #95411 ) ;
#79217=CARTESIAN_POINT ( 'NONE',  ( -57.88150100324660485, 35.92665207732901678, -10.00000000000000000 ) ) ;
#79218=LINE ( 'NONE', #48783, #35465 ) ;
#79224=DIRECTION ( 'NONE',  ( 0.8660254037844379305, 0.5000000000000011102, 0.000000000000000000 ) ) ;
#79232=VECTOR ( 'NONE', #58, 1000.000000000000000 ) ;
#79234=CARTESIAN_POINT ( 'NONE',  ( 45.80758703142364396, 72.03864405183792030, -10.00000000000000000 ) ) ;
#79236=ORIENTED_EDGE ( 'NONE', *, *, #35525, .F. ) ;
#79260=VERTEX_POINT ( 'NONE', #39449 ) ;
#79262=ORIENTED_EDGE ( 'NONE', *, *, #81189, .F. ) ;
#79264=CARTESIAN_POINT ( 'NONE',  ( -19.65312891409030271, 93.06504152958497400, 10.00000000000000888 ) ) ;
#79274=VECTOR ( 'NONE', #71764, 1000.000000000000000 ) ;
#79280=CARTESIAN_POINT ( 'NONE',  ( -50.66096862766640641, 31.69950886434491721, -10.00000000000000000 ) ) ;
#79283=VERTEX_POINT ( 'NONE', #93207 ) ;
#79284=EDGE_LOOP ( 'NONE', ( #31687, #64125, #34007, #20504 ) ) ;
#79288=DIRECTION ( 'NONE',  ( -0.09274582908234035861, -0.9956898167541080591, 0.000000000000000000 ) ) ;
#79293=VECTOR ( 'NONE', #84525, 1000.000000000000000 ) ;
#79300=EDGE_CURVE ( 'NONE', #65492, #37083, #12588, .T. ) ;
#79304=LINE ( 'NONE', #88414, #34057 ) ;
#79308=VECTOR ( 'NONE', #89099, 1000.000000000000000 ) ;
#79313=VECTOR ( 'NONE', #24810, 1000.000000000000000 ) ;
#79315=CARTESIAN_POINT ( 'NONE',  ( 23.64814127513158937, 118.0650415295850451, 60.00000000000000000 ) ) ;
#79317=DIRECTION ( 'NONE',  ( 1.000000000000000000, 0.000000000000000000, 0.000000000000000000 ) ) ;
#79337=CIRCLE ( 'NONE', #95551, 70.00000000000001421 ) ;
#79340=DIRECTION ( 'NONE',  ( -0.009162850352631533510, 0.9999580202055560196, 0.000000000000000000 ) ) ;
#79350=ORIENTED_EDGE ( 'NONE', *, *, #94138, .T. ) ;
#79353=DIRECTION ( 'NONE',  ( 0.000000000000000000, 0.000000000000000000, 1.000000000000000000 ) ) ;
#79359=AXIS2_PLACEMENT_3D ( 'NONE', #51725, #82668, #81655 ) ;
#79361=VERTEX_POINT ( 'NONE', #18187 ) ;
#79369=CARTESIAN_POINT ( 'NONE',  ( 39.77289032284285497, 58.49985355908045648, 10.00000000000000000 ) ) ;
#79371=ORIENTED_EDGE ( 'NONE', *, *, #89569, .F. ) ;
#79409=EDGE_LOOP ( 'NONE', ( #56364, #24619, #84622, #1216 ) ) ;
#79411=CARTESIAN_POINT ( 'NONE',  ( -42.18579364100346396, 26.51648975995176372, 10.00000000000000000 ) ) ;
#79426=CARTESIAN_POINT ( 'NONE',  ( 39.01205572417272549, 91.95295005193447935, 59.99999999999999289 ) ) ;
#79428=CARTESIAN_POINT ( 'NONE',  ( -76.38857681351474582, 54.22815603855766398, -10.00000000000000000 ) ) ;
#79431=VECTOR ( 'NONE', #59030, 1000.000000000000114 ) ;
#79432=CARTESIAN_POINT ( 'NONE',  ( 44.73065482718367747, 120.5373619841236774, 10.00000000000000000 ) ) ;
#79450=DIRECTION ( 'NONE',  ( 1.000000000000000000, 0.000000000000000000, 0.000000000000000000 ) ) ;
#79457=LINE ( 'NONE', #47997, #16087 ) ;
#79460=EDGE_CURVE ( 'NONE', #74753, #93745, #51568, .T. ) ;
#79467=DIRECTION ( 'NONE',  ( 0.8261602328994307465, -0.5634352399127678934, 0.000000000000000000 ) ) ;
#79477=ORIENTED_EDGE ( 'NONE', *, *, #50619, .F. ) ;
#79481=CARTESIAN_POINT ( 'NONE',  ( -71.61465314115659453, 63.06504152958490295, -10.00000000000000888 ) ) ;
#79482=EDGE_CURVE ( 'NONE', #3700, #38681, #56457, .T. ) ;
#79498=ORIENTED_EDGE ( 'NONE', *, *, #46049, .T. ) ;
#79499=VECTOR ( 'NONE', #68349, 1000.000000000000000 ) ;
#79500=VERTEX_POINT ( 'NONE', #46955 ) ;
#79504=LINE ( 'NONE', #87133, #27065 ) ;
#79515=LINE ( 'NONE', #93197, #70689 ) ;
#79532=ORIENTED_EDGE ( 'NONE', *, *, #57949, .T. ) ;
#79535=ADVANCED_FACE ( 'NONE', ( #89035 ), #2376, .F. ) ;
#79537=DIRECTION ( 'NONE',  ( -0.6911977992267216431, 0.7226656227773233798, 0.000000000000000000 ) ) ;
#79538=CARTESIAN_POINT ( 'NONE',  ( -19.65312891409030271, 93.06504152958497400, 60.00000000000000000 ) ) ;
#79540=ORIENTED_EDGE ( 'NONE', *, *, #42578, .F. ) ;
#79546=LINE ( 'NONE', #33917, #52918 ) ;
#79553=LINE ( 'NONE', #10108, #4249 ) ;
#79567=VECTOR ( 'NONE', #12533, 1000.000000000000000 ) ;
#79573=DIRECTION ( 'NONE',  ( -0.000000000000000000, 0.000000000000000000, -1.000000000000000000 ) ) ;
#79593=CARTESIAN_POINT ( 'NONE',  ( -8.440768550191725339, 84.85656262831267327, 13.91600492330110228 ) ) ;
#79595=EDGE_CURVE ( 'NONE', #21922, #6854, #10793, .T. ) ;
#79596=CARTESIAN_POINT ( 'NONE',  ( 32.61785165683026122, 46.50599740114041225, -10.00000000000000000 ) ) ;
#79601=CARTESIAN_POINT ( 'NONE',  ( -12.95261720355844126, 24.63757726406876714, -10.00000000000000000 ) ) ;
#79611=ORIENTED_EDGE ( 'NONE', *, *, #70651, .T. ) ;
#79615=CARTESIAN_POINT ( 'NONE',  ( -19.71336475592354986, 93.19343694228106756, 59.99999999999999289 ) ) ;
#79620=( NAMED_UNIT ( * ) PLANE_ANGLE_UNIT ( ) SI_UNIT ( $, .RADIAN. ) );
#79622=VERTEX_POINT ( 'NONE', #49288 ) ;
#79624=CARTESIAN_POINT ( 'NONE',  ( 48.98007068238331385, 88.97864505566217019, -10.00000000000000000 ) ) ;
#79630=ORIENTED_EDGE ( 'NONE', *, *, #64053, .F. ) ;
#79632=VERTEX_POINT ( 'NONE', #89812 ) ;
#79651=EDGE_CURVE ( 'NONE', #6303, #29146, #27963, .T. ) ;
#79656=DIRECTION ( 'NONE',  ( -0.9506327454577400138, -0.3103181967972222788, 0.000000000000000000 ) ) ;
#79658=DIRECTION ( 'NONE',  ( 1.000000000000000000, 0.000000000000000000, 0.000000000000000000 ) ) ;
#79665=DIRECTION ( 'NONE',  ( 0.8653701635463924013, -0.5011331959107180323, 0.000000000000000000 ) ) ;
#79669=VERTEX_POINT ( 'NONE', #21371 ) ;
#79675=CARTESIAN_POINT ( 'NONE',  ( -22.03161396778968140, 40.09437670360522077, 59.99999999999999289 ) ) ;
#79680=AXIS2_PLACEMENT_3D ( 'NONE', #20660, #51549, #28244 ) ;
#79714=DIRECTION ( 'NONE',  ( 0.3887219701523905169, 0.9213551052231946370, 0.000000000000000000 ) ) ;
#79715=FACE_OUTER_BOUND ( 'NONE', #39671, .T. ) ;
#79721=LINE ( 'NONE', #19884, #23859 ) ;
#79727=CARTESIAN_POINT ( 'NONE',  ( 11.76667899187106059, 31.90941714274742225, 10.00000000000000000 ) ) ;
#79731=ADVANCED_FACE ( 'NONE', ( #69453 ), #39034, .T. ) ;
#79735=CARTESIAN_POINT ( 'NONE',  ( 47.84007798744509898, 106.1754093786579318, 10.00000000000000000 ) ) ;
#79741=DIRECTION ( 'NONE',  ( 0.000000000000000000, 0.000000000000000000, 1.000000000000000000 ) ) ;
#79743=EDGE_LOOP ( 'NONE', ( #14908, #97783, #86389, #74445 ) ) ;
#79745=DIRECTION ( 'NONE',  ( -0.7510153523339188064, 0.6602847420308604054, 0.000000000000000000 ) ) ;
#79746=VERTEX_POINT ( 'NONE', #73964 ) ;
#79756=ORIENTED_EDGE ( 'NONE', *, *, #82136, .T. ) ;
#79761=ORIENTED_EDGE ( 'NONE', *, *, #92568, .F. ) ;
#79765=VERTEX_POINT ( 'NONE', #87734 ) ;
#79781=VERTEX_POINT ( 'NONE', #65353 ) ;
#79784=EDGE_CURVE ( 'NONE', #64892, #83079, #33461, .T. ) ;
#79786=CARTESIAN_POINT ( 'NONE',  ( -69.61464189717713680, 45.83092310410447112, -10.00000000000000000 ) ) ;
#79790=LINE ( 'NONE', #33658, #83471 ) ;
#79793=CARTESIAN_POINT ( 'NONE',  ( -5.997209913151932525, 43.16835788936899831, 59.99999999999999289 ) ) ;
#79796=FACE_OUTER_BOUND ( 'NONE', #25383, .T. ) ;
#79833=DIRECTION ( 'NONE',  ( -1.000000000000000000, -9.785293164094327883E-14, 0.000000000000000000 ) ) ;
#79836=DIRECTION ( 'NONE',  ( -1.000000000000000000, 0.000000000000000000, 0.000000000000000000 ) ) ;
#79838=VERTEX_POINT ( 'NONE', #6044 ) ;
#79857=EDGE_CURVE ( 'NONE', #10835, #1376, #69401, .T. ) ;
#79865=VERTEX_POINT ( 'NONE', #87499 ) ;
#79875=ORIENTED_EDGE ( 'NONE', *, *, #46640, .F. ) ;
#79886=DIRECTION ( 'NONE',  ( -0.000000000000000000, -0.000000000000000000, 1.000000000000000000 ) ) ;
#79887=DIRECTION ( 'NONE',  ( 0.9505498757754579087, -0.3105719460338643434, 0.000000000000000000 ) ) ;
#79892=EDGE_LOOP ( 'NONE', ( #57908, #61874, #21631, #37226 ) ) ;
#79893=CARTESIAN_POINT ( 'NONE',  ( -77.42978507651396569, 55.80833764325424085, -10.00000000000000000 ) ) ;
#79894=ORIENTED_EDGE ( 'NONE', *, *, #6952, .F. ) ;
#79901=CARTESIAN_POINT ( 'NONE',  ( -19.65312891409030271, 93.06504152958497400, 10.00000000000000888 ) ) ;
#79905=ORIENTED_EDGE ( 'NONE', *, *, #19477, .F. ) ;
#79906=LINE ( 'NONE', #27172, #70475 ) ;
#79908=AXIS2_PLACEMENT_3D ( 'NONE', #15996, #16985, #15478 ) ;
#79909=VERTEX_POINT ( 'NONE', #85984 ) ;
#79910=DIRECTION ( 'NONE',  ( -0.2168075248790319320, -0.9762143704923770260, 0.000000000000000000 ) ) ;
#79911=VECTOR ( 'NONE', #91319, 1000.000000000000114 ) ;
#79914=DIRECTION ( 'NONE',  ( -1.000000000000000000, 0.000000000000000000, 0.000000000000000000 ) ) ;
#79917=CARTESIAN_POINT ( 'NONE',  ( -19.76310821406011797, 93.15458644692216694, 59.99999999999999289 ) ) ;
#79933=DIRECTION ( 'NONE',  ( 1.000000000000000000, 0.000000000000000000, 0.000000000000000000 ) ) ;
#79935=CARTESIAN_POINT ( 'NONE',  ( 33.22460751122017086, 89.13141723973357955, 59.99999999999999289 ) ) ;
#79966=DIRECTION ( 'NONE',  ( 0.000000000000000000, 0.000000000000000000, 1.000000000000000000 ) ) ;
#79968=CARTESIAN_POINT ( 'NONE',  ( 0.2713214620000473087, 45.32428913435456508, 59.99999999999999289 ) ) ;
#79974=EDGE_LOOP ( 'NONE', ( #62533, #95594, #8254, #69224 ) ) ;
#79976=DIRECTION ( 'NONE',  ( -0.3956464567955659817, 0.9184028970038772277, 0.000000000000000000 ) ) ;
#79980=DIRECTION ( 'NONE',  ( 1.000000000000000000, 0.000000000000000000, 0.000000000000000000 ) ) ;
#79982=VERTEX_POINT ( 'NONE', #78837 ) ;
#79991=DIRECTION ( 'NONE',  ( -1.000000000000000000, 0.000000000000000000, 0.000000000000000000 ) ) ;
#79992=CARTESIAN_POINT ( 'NONE',  ( 17.60357497223980516, 35.28838536716092023, -10.00000000000000000 ) ) ;
#79993=ORIENTED_EDGE ( 'NONE', *, *, #2200, .T. ) ;
#80000=LINE ( 'NONE', #65254, #83683 ) ;
#80006=ORIENTED_EDGE ( 'NONE', *, *, #74081, .F. ) ;
#80008=LINE ( 'NONE', #62751, #98196 ) ;
#80015=LINE ( 'NONE', #24278, #22267 ) ;
#80021=EDGE_LOOP ( 'NONE', ( #65109, #96170, #68254, #37512 ) ) ;
#80031=ORIENTED_EDGE ( 'NONE', *, *, #85082, .T. ) ;
#80048=EDGE_CURVE ( 'NONE', #49899, #14660, #57504, .T. ) ;
#80059=DIRECTION ( 'NONE',  ( -1.000000000000000000, 0.000000000000000000, 0.000000000000000000 ) ) ;
#80064=CARTESIAN_POINT ( 'NONE',  ( -19.65312891409030271, 93.06504152958497400, 59.99999999999999289 ) ) ;
#80065=ORIENTED_EDGE ( 'NONE', *, *, #11339, .T. ) ;
#80071=FACE_OUTER_BOUND ( 'NONE', #72145, .T. ) ;
#80076=CARTESIAN_POINT ( 'NONE',  ( 44.18794977381974576, 118.5901545549086791, -10.00000000000000000 ) ) ;
#80077=DIRECTION ( 'NONE',  ( -0.5637708215276967527, 0.8259312688075115538, 0.000000000000000000 ) ) ;
#80078=ADVANCED_FACE ( 'NONE', ( #97060 ), #88482, .F. ) ;
#80082=ADVANCED_FACE ( 'NONE', ( #50407 ), #74739, .F. ) ;
#80085=CARTESIAN_POINT ( 'NONE',  ( 49.07456115661582174, 91.13648234292965356, -10.00000000000000000 ) ) ;
#80089=ORIENTED_EDGE ( 'NONE', *, *, #95683, .T. ) ;
#80090=CARTESIAN_POINT ( 'NONE',  ( -12.93060150105072559, 85.35421234851665417, 14.87203518896413357 ) ) ;
#80093=EDGE_CURVE ( 'NONE', #42773, #66517, #43295, .T. ) ;
#80094=ORIENTED_EDGE ( 'NONE', *, *, #50446, .F. ) ;
#80120=ORIENTED_EDGE ( 'NONE', *, *, #12713, .F. ) ;
#80126=VECTOR ( 'NONE', #55274, 1000.000000000000114 ) ;
#80130=ORIENTED_EDGE ( 'NONE', *, *, #99469, .T. ) ;
#80138=PLANE ( 'NONE',  #96854 ) ;
#80141=ORIENTED_EDGE ( 'NONE', *, *, #53379, .T. ) ;
#80145=VERTEX_POINT ( 'NONE', #2719 ) ;
#80152=EDGE_CURVE ( 'NONE', #23598, #99548, #56885, .T. ) ;
#80156=FACE_OUTER_BOUND ( 'NONE', #9199, .T. ) ;
#80158=ORIENTED_EDGE ( 'NONE', *, *, #59202, .F. ) ;
#80166=ORIENTED_EDGE ( 'NONE', *, *, #27009, .F. ) ;
#80178=EDGE_CURVE ( 'NONE', #92469, #34673, #59698, .T. ) ;
#80188=ORIENTED_EDGE ( 'NONE', *, *, #68378, .F. ) ;
#80200=DIRECTION ( 'NONE',  ( -0.9302793824855987159, 0.3668518372888612822, 0.000000000000000000 ) ) ;
#80205=CARTESIAN_POINT ( 'NONE',  ( 38.38820426754037385, 84.46014300635468430, 59.99999999999999289 ) ) ;
#80226=EDGE_CURVE ( 'NONE', #88881, #5812, #71115, .T. ) ;
#80230=ORIENTED_EDGE ( 'NONE', *, *, #14355, .T. ) ;
#80251=AXIS2_PLACEMENT_3D ( 'NONE', #31280, #93117, #52582 ) ;
#80278=ORIENTED_EDGE ( 'NONE', *, *, #287, .T. ) ;
#80286=VERTEX_POINT ( 'NONE', #48304 ) ;
#80288=DIRECTION ( 'NONE',  ( 0.000000000000000000, 0.000000000000000000, 1.000000000000000000 ) ) ;
#80296=VECTOR ( 'NONE', #93214, 1000.000000000000000 ) ;
#80298=ORIENTED_EDGE ( 'NONE', *, *, #39701, .F. ) ;
#80306=CARTESIAN_POINT ( 'NONE',  ( -19.79494373018473752, 93.06352608284200301, 59.99999999999999289 ) ) ;
#80321=FACE_OUTER_BOUND ( 'NONE', #14770, .T. ) ;
#80325=ORIENTED_EDGE ( 'NONE', *, *, #42972, .F. ) ;
#80326=VECTOR ( 'NONE', #70292, 1000.000000000000000 ) ;
#80328=ADVANCED_FACE ( 'NONE', ( #97905 ), #49305, .F. ) ;
#80359=ORIENTED_EDGE ( 'NONE', *, *, #76524, .F. ) ;
#80365=CARTESIAN_POINT ( 'NONE',  ( 50.18541494347881837, 88.31343213334855591, -10.00000000000000000 ) ) ;
#80368=VECTOR ( 'NONE', #34636, 1000.000000000000227 ) ;
#80370=CIRCLE ( 'NONE', #73821, 0.1418229129684298040 ) ;
#80376=PLANE ( 'NONE',  #95048 ) ;
#80377=VECTOR ( 'NONE', #95725, 1000.000000000000000 ) ;
#80384=ORIENTED_EDGE ( 'NONE', *, *, #92875, .T. ) ;
#80398=ORIENTED_EDGE ( 'NONE', *, *, #45087, .T. ) ;
#80400=ORIENTED_EDGE ( 'NONE', *, *, #7786, .T. ) ;
#80403=LINE ( 'NONE', #64665, #55996 ) ;
#80408=VECTOR ( 'NONE', #94700, 1000.000000000000114 ) ;
#80413=VERTEX_POINT ( 'NONE', #60358 ) ;
#80414=DIRECTION ( 'NONE',  ( -0.000000000000000000, -0.000000000000000000, -1.000000000000000000 ) ) ;
#80422=CARTESIAN_POINT ( 'NONE',  ( -19.65312891409030271, 93.06504152958497400, -10.00000000000000888 ) ) ;
#80424=DIRECTION ( 'NONE',  ( -1.000000000000000000, 0.000000000000000000, 0.000000000000000000 ) ) ;
#80425=VERTEX_POINT ( 'NONE', #68968 ) ;
#80428=EDGE_CURVE ( 'NONE', #61894, #16667, #29485, .T. ) ;
#80430=DIRECTION ( 'NONE',  ( 0.9662637919863205083, 0.2575544297740129385, 0.000000000000000000 ) ) ;
#80433=CARTESIAN_POINT ( 'NONE',  ( -19.75075453565523986, 93.16791512511277062, 59.99999999999999289 ) ) ;
#80440=CARTESIAN_POINT ( 'NONE',  ( 22.66956910419568061, 38.88013629349136835, 10.00000000000000000 ) ) ;
#80443=AXIS2_PLACEMENT_3D ( 'NONE', #73485, #12180, #43041 ) ;
#80451=EDGE_CURVE ( 'NONE', #63400, #55233, #61859, .T. ) ;
#80473=DIRECTION ( 'NONE',  ( -0.6361630342459823062, 0.7715546603183375263, 0.000000000000000000 ) ) ;
#80487=ORIENTED_EDGE ( 'NONE', *, *, #27009, .T. ) ;
#80492=EDGE_CURVE ( 'NONE', #20754, #68396, #15256, .T. ) ;
#80493=EDGE_LOOP ( 'NONE', ( #36421, #44664, #70453, #27999 ) ) ;
#80505=DIRECTION ( 'NONE',  ( 0.000000000000000000, 0.000000000000000000, 1.000000000000000000 ) ) ;
#80519=PLANE ( 'NONE',  #1359 ) ;
#80524=VECTOR ( 'NONE', #21939, 1000.000000000000000 ) ;
#80525=ORIENTED_EDGE ( 'NONE', *, *, #84765, .F. ) ;
#80527=ORIENTED_EDGE ( 'NONE', *, *, #46979, .T. ) ;
#80534=DIRECTION ( 'NONE',  ( -0.000000000000000000, -0.000000000000000000, 1.000000000000000000 ) ) ;
#80537=VECTOR ( 'NONE', #96858, 1000.000000000000114 ) ;
#80543=ADVANCED_FACE ( 'NONE', ( #76584 ), #59873, .F. ) ;
#80544=CARTESIAN_POINT ( 'NONE',  ( 41.71240375114939525, 62.05720181600818108, -10.00000000000000000 ) ) ;
#80546=EDGE_CURVE ( 'NONE', #58606, #46023, #17634, .T. ) ;
#80555=EDGE_CURVE ( 'NONE', #89858, #91333, #75596, .T. ) ;
#80562=FACE_OUTER_BOUND ( 'NONE', #8597, .T. ) ;
#80563=DIRECTION ( 'NONE',  ( -1.000000000000000000, 0.000000000000000000, 0.000000000000000000 ) ) ;
#80570=AXIS2_PLACEMENT_3D ( 'NONE', #56177, #94236, #71413 ) ;
#80575=AXIS2_PLACEMENT_3D ( 'NONE', #73264, #81889, #28144 ) ;
#80580=PRODUCT_DEFINITION ( 'UNKNOWN', '', #20351, #86920 ) ;
#80585=LINE ( 'NONE', #50134, #29515 ) ;
#80586=CARTESIAN_POINT ( 'NONE',  ( -63.30067564770008914, 39.94154026010144065, -10.00000000000000000 ) ) ;
#80587=VECTOR ( 'NONE', #55488, 1000.000000000000227 ) ;
#80593=CARTESIAN_POINT ( 'NONE',  ( -27.77457187288641904, 24.79904599702367562, 10.00000000000000000 ) ) ;
#80597=AXIS2_PLACEMENT_3D ( 'NONE', #96299, #72496, #55733 ) ;
#80606=EDGE_LOOP ( 'NONE', ( #62485, #92937, #85071, #5210 ) ) ;
#80609=DIRECTION ( 'NONE',  ( 0.7891516029629116469, -0.6141984594095519778, 0.000000000000000000 ) ) ;
#80610=ORIENTED_EDGE ( 'NONE', *, *, #32982, .F. ) ;
#80618=VECTOR ( 'NONE', #77261, 1000.000000000000114 ) ;
#80627=EDGE_CURVE ( 'NONE', #53524, #95233, #14374, .T. ) ;
#80634=ORIENTED_EDGE ( 'NONE', *, *, #89614, .F. ) ;
#80636=FACE_BOUND ( 'NONE', #8587, .T. ) ;
#80639=PLANE ( 'NONE',  #65941 ) ;
#80643=ORIENTED_EDGE ( 'NONE', *, *, #83127, .F. ) ;
#80646=VECTOR ( 'NONE', #34771, 1000.000000000000114 ) ;
#80653=VECTOR ( 'NONE', #26670, 999.9999999999998863 ) ;
#80660=CIRCLE ( 'NONE', #90344, 45.00000000000000000 ) ;
#80670=ORIENTED_EDGE ( 'NONE', *, *, #11107, .F. ) ;
#80674=CARTESIAN_POINT ( 'NONE',  ( 19.39999966495784989, 36.48715600906564305, -10.00000000000000000 ) ) ;
#80681=CARTESIAN_POINT ( 'NONE',  ( -19.65312891409030271, 93.06504152958497400, 40.00000000000000000 ) ) ;
#80695=DIRECTION ( 'NONE',  ( -0.000000000000000000, 0.000000000000000000, -1.000000000000000000 ) ) ;
#80698=VECTOR ( 'NONE', #16840, 1000.000000000000114 ) ;
#80710=CARTESIAN_POINT ( 'NONE',  ( 49.09806598349715046, 107.5461990276917845, -10.00000000000000000 ) ) ;
#80711=CARTESIAN_POINT ( 'NONE',  ( 41.71240375114938814, 62.05720181600818108, -10.00000000000000000 ) ) ;
#80718=VECTOR ( 'NONE', #5383, 1000.000000000000000 ) ;
#80728=DIRECTION ( 'NONE',  ( -0.9184028970038814466, -0.3956464567955564338, 0.000000000000000000 ) ) ;
#80736=EDGE_CURVE ( 'NONE', #46169, #70584, #94317, .T. ) ;
#80741=LINE ( 'NONE', #11314, #15452 ) ;
#80742=EDGE_CURVE ( 'NONE', #10473, #77961, #63875, .T. ) ;
#80743=ORIENTED_EDGE ( 'NONE', *, *, #43638, .T. ) ;
#80744=CARTESIAN_POINT ( 'NONE',  ( 34.81516168915606357, 51.10768172523390973, -10.00000000000000000 ) ) ;
#80750=ORIENTED_EDGE ( 'NONE', *, *, #33134, .F. ) ;
#80757=ORIENTED_EDGE ( 'NONE', *, *, #95672, .F. ) ;
#80759=CARTESIAN_POINT ( 'NONE',  ( -0.3272207041121033000, 38.43844835668754456, 59.99999999999999289 ) ) ;
#80767=VERTEX_POINT ( 'NONE', #43562 ) ;
#80773=VERTEX_POINT ( 'NONE', #13673 ) ;
#80774=DIRECTION ( 'NONE',  ( -0.7713848165480284846, 0.6363689690731033632, 0.000000000000000000 ) ) ;
#80775=ORIENTED_EDGE ( 'NONE', *, *, #3280, .F. ) ;
#80791=EDGE_CURVE ( 'NONE', #77592, #23277, #4694, .T. ) ;
#80794=CARTESIAN_POINT ( 'NONE',  ( -38.02969130575858259, 25.52022711230254970, 10.00000000000000000 ) ) ;
#80801=LINE ( 'NONE', #81285, #98121 ) ;
#80802=VECTOR ( 'NONE', #6843, 1000.000000000000000 ) ;
#80803=DIRECTION ( 'NONE',  ( 0.000000000000000000, 0.000000000000000000, 1.000000000000000000 ) ) ;
#80807=VECTOR ( 'NONE', #21025, 1000.000000000000000 ) ;
#80816=VECTOR ( 'NONE', #76864, 1000.000000000000227 ) ;
#80817=ORIENTED_EDGE ( 'NONE', *, *, #20929, .F. ) ;
#80835=LINE ( 'NONE', #57459, #85642 ) ;
#80837=FACE_OUTER_BOUND ( 'NONE', #17269, .T. ) ;
#80851=ORIENTED_EDGE ( 'NONE', *, *, #66425, .F. ) ;
#80854=CARTESIAN_POINT ( 'NONE',  ( -43.70040200909112116, 27.32518560721127088, 10.00000000000000000 ) ) ;
#80863=CARTESIAN_POINT ( 'NONE',  ( 50.51697681462041345, 96.61285555410614734, 10.00000000000000000 ) ) ;
#80867=CARTESIAN_POINT ( 'NONE',  ( 29.12701137275935181, 44.61184105132205957, 10.00000000000000000 ) ) ;
#80869=CARTESIAN_POINT ( 'NONE',  ( -19.65312891409030271, 93.06504152958497400, 177.5919119679930134 ) ) ;
#80874=EDGE_LOOP ( 'NONE', ( #48364, #93471, #43712, #30139 ) ) ;
#80875=EDGE_CURVE ( 'NONE', #23251, #59397, #65743, .T. ) ;
#80876=VECTOR ( 'NONE', #59829, 1000.000000000000114 ) ;
#80880=VECTOR ( 'NONE', #22822, 1000.000000000000114 ) ;
#80881=DIRECTION ( 'NONE',  ( 0.6118251767726274881, 0.7909930170786233505, 0.000000000000000000 ) ) ;
#80893=DIRECTION ( 'NONE',  ( -0.000000000000000000, 0.000000000000000000, -1.000000000000000000 ) ) ;
#80908=VECTOR ( 'NONE', #71731, 1000.000000000000000 ) ;
#80910=EDGE_LOOP ( 'NONE', ( #76447, #74467, #89839, #99799, #39902 ) ) ;
#80913=AXIS2_PLACEMENT_3D ( 'NONE', #61803, #85159, #77537 ) ;
#80921=DIRECTION ( 'NONE',  ( 0.000000000000000000, 0.000000000000000000, 1.000000000000000000 ) ) ;
#80924=ORIENTED_EDGE ( 'NONE', *, *, #66557, .F. ) ;
#80937=EDGE_CURVE ( 'NONE', #43692, #76267, #35351, .T. ) ;
#80940=CARTESIAN_POINT ( 'NONE',  ( -38.68484055605311056, 44.96122434458596473, 59.99999999999999289 ) ) ;
#80948=VECTOR ( 'NONE', #19069, 1000.000000000000000 ) ;
#80955=DIRECTION ( 'NONE',  ( -0.000000000000000000, -0.000000000000000000, -1.000000000000000000 ) ) ;
#80958=CIRCLE ( 'NONE', #19474, 50.00000000000000711 ) ;
#80971=VERTEX_POINT ( 'NONE', #71879 ) ;
#80975=LINE ( 'NONE', #4414, #71717 ) ;
#80990=EDGE_LOOP ( 'NONE', ( #49417, #9622, #74773, #5087 ) ) ;
#81005=EDGE_CURVE ( 'NONE', #79500, #42726, #85005, .T. ) ;
#81007=VERTEX_POINT ( 'NONE', #5977 ) ;
#81015=DIRECTION ( 'NONE',  ( -0.3696446237802353263, -0.9291732088853875693, 0.000000000000000000 ) ) ;
#81025=VERTEX_POINT ( 'NONE', #21682 ) ;
#81029=CARTESIAN_POINT ( 'NONE',  ( -19.65312891409030271, 93.06504152958497400, 59.99999999999999289 ) ) ;
#81034=CIRCLE ( 'NONE', #19538, 0.1418229129680863287 ) ;
#81035=ORIENTED_EDGE ( 'NONE', *, *, #35397, .F. ) ;
#81038=ORIENTED_EDGE ( 'NONE', *, *, #41742, .F. ) ;
#81045=DIRECTION ( 'NONE',  ( 1.000000000000000000, 0.000000000000000000, 0.000000000000000000 ) ) ;
#81050=DIRECTION ( 'NONE',  ( -0.000000000000000000, -0.000000000000000000, -1.000000000000000000 ) ) ;
#81052=CARTESIAN_POINT ( 'NONE',  ( 40.96864935082037817, 128.0650415295850735, 177.5919119679930134 ) ) ;
#81053=CARTESIAN_POINT ( 'NONE',  ( 5.871984111234073822, 29.22396284167520619, -10.00000000000000000 ) ) ;
#81062=EDGE_CURVE ( 'NONE', #98305, #68897, #6484, .T. ) ;
#81067=LINE ( 'NONE', #49608, #91941 ) ;
#81068=CARTESIAN_POINT ( 'NONE',  ( -73.66720466879951346, 50.53642055324488780, 10.00000000000000000 ) ) ;
#81073=VERTEX_POINT ( 'NONE', #60648 ) ;
#81093=EDGE_LOOP ( 'NONE', ( #10444, #24864, #30552, #89487 ) ) ;
#81096=CARTESIAN_POINT ( 'NONE',  ( -12.28238420462231950, 85.48259521052763432, 14.78036012837727142 ) ) ;
#81107=ORIENTED_EDGE ( 'NONE', *, *, #89571, .T. ) ;
#81121=DIRECTION ( 'NONE',  ( 0.9874311856918874808, -0.1580495287025984186, 0.000000000000000000 ) ) ;
#81133=ORIENTED_EDGE ( 'NONE', *, *, #40577, .F. ) ;
#81145=CARTESIAN_POINT ( 'NONE',  ( 40.48539884740146277, 126.3902902409112556, -10.00000000000000000 ) ) ;
#81152=DIRECTION ( 'NONE',  ( -0.000000000000000000, 0.000000000000000000, 1.000000000000000000 ) ) ;
#81155=CARTESIAN_POINT ( 'NONE',  ( -61.60412911085353471, 37.02832515102500111, -10.00000000000000000 ) ) ;
#81157=VERTEX_POINT ( 'NONE', #27182 ) ;
#81160=VERTEX_POINT ( 'NONE', #18589 ) ;
#81163=DIRECTION ( 'NONE',  ( -0.9862134920484688649, -0.1654779384134468789, 0.000000000000000000 ) ) ;
#81167=AXIS2_PLACEMENT_3D ( 'NONE', #37292, #68187, #46369 ) ;
#81168=CARTESIAN_POINT ( 'NONE',  ( -19.65312891409030271, 93.06504152958497400, 177.5919119679930134 ) ) ;
#81169=EDGE_LOOP ( 'NONE', ( #32914, #93195, #64010, #31102 ) ) ;
#81177=EDGE_CURVE ( 'NONE', #73688, #54866, #35766, .T. ) ;
#81184=CARTESIAN_POINT ( 'NONE',  ( -8.517573342504920930, 41.22347591502147424, 59.99999999999999289 ) ) ;
#81189=EDGE_CURVE ( 'NONE', #72634, #28659, #58554, .T. ) ;
#81201=CARTESIAN_POINT ( 'NONE',  ( -66.55019942848203129, 42.78701949053055387, -10.00000000000000000 ) ) ;
#81222=CARTESIAN_POINT ( 'NONE',  ( 12.00096474099108690, 32.03863464977599307, -10.00000000000000000 ) ) ;
#81227=EDGE_CURVE ( 'NONE', #11943, #43088, #49467, .T. ) ;
#81228=VERTEX_POINT ( 'NONE', #33798 ) ;
#81233=VECTOR ( 'NONE', #76555, 1000.000000000000000 ) ;
#81234=VERTEX_POINT ( 'NONE', #81908 ) ;
#81236=DIRECTION ( 'NONE',  ( -0.000000000000000000, -0.000000000000000000, -1.000000000000000000 ) ) ;
#81242=ORIENTED_EDGE ( 'NONE', *, *, #72364, .F. ) ;
#81244=EDGE_CURVE ( 'NONE', #22484, #44226, #32299, .T. ) ;
#81248=LINE ( 'NONE', #19439, #92149 ) ;
#81256=VERTEX_POINT ( 'NONE', #10479 ) ;
#81257=DIRECTION ( 'NONE',  ( -0.3177184104407523857, 0.9481851146622171100, 0.000000000000000000 ) ) ;
#81263=DIRECTION ( 'NONE',  ( -0.000000000000000000, -0.000000000000000000, -1.000000000000000000 ) ) ;
#81271=VECTOR ( 'NONE', #17923, 1000.000000000000000 ) ;
#81273=LINE ( 'NONE', #52309, #46059 ) ;
#81279=LINE ( 'NONE', #42222, #8496 ) ;
#81284=DIRECTION ( 'NONE',  ( -0.7561390817803280706, 0.6544109481086042290, 0.000000000000000000 ) ) ;
#81285=CARTESIAN_POINT ( 'NONE',  ( -56.14442822474985206, 33.32908021129814813, 177.5919119679930134 ) ) ;
#81286=VECTOR ( 'NONE', #21963, 1000.000000000000114 ) ;
#81300=DIRECTION ( 'NONE',  ( -0.5435407515102007592, 0.8393827800519415572, 0.000000000000000000 ) ) ;
#81302=EDGE_CURVE ( 'NONE', #84216, #54173, #64646, .T. ) ;
#81313=ADVANCED_FACE ( 'NONE', ( #81413 ), #26180, .F. ) ;
#81321=DIRECTION ( 'NONE',  ( -0.5000000000000012212, 0.8660254037844379305, 0.000000000000000000 ) ) ;
#81333=CARTESIAN_POINT ( 'NONE',  ( -7.521556465916533263, 24.12430647450514343, 177.5919119679930134 ) ) ;
#81336=DIRECTION ( 'NONE',  ( 0.000000000000000000, 0.000000000000000000, 1.000000000000000000 ) ) ;
#81337=ORIENTED_EDGE ( 'NONE', *, *, #41323, .F. ) ;
#81346=DIRECTION ( 'NONE',  ( 0.000000000000000000, 0.000000000000000000, 1.000000000000000000 ) ) ;
#81355=ADVANCED_FACE ( 'NONE', ( #23096 ), #60592, .F. ) ;
#81364=ORIENTED_EDGE ( 'NONE', *, *, #6952, .T. ) ;
#81366=EDGE_CURVE ( 'NONE', #81007, #3700, #100130, .T. ) ;
#81368=VECTOR ( 'NONE', #65040, 1000.000000000000000 ) ;
#81370=ORIENTED_EDGE ( 'NONE', *, *, #89907, .F. ) ;
#81373=LINE ( 'NONE', #73731, #53712 ) ;
#81388=DIRECTION ( 'NONE',  ( 0.000000000000000000, 0.000000000000000000, 1.000000000000000000 ) ) ;
#81394=EDGE_LOOP ( 'NONE', ( #12060, #43964, #70892, #15265 ) ) ;
#81395=CARTESIAN_POINT ( 'NONE',  ( -19.65312891409030271, 93.06504152958497400, -10.00000000000000888 ) ) ;
#81396=VERTEX_POINT ( 'NONE', #24104 ) ;
#81398=DIRECTION ( 'NONE',  ( -0.1550826972584532226, -0.9879014915521905360, 0.000000000000000000 ) ) ;
#81403=ORIENTED_EDGE ( 'NONE', *, *, #23068, .T. ) ;
#81406=ORIENTED_EDGE ( 'NONE', *, *, #60899, .T. ) ;
#81410=CARTESIAN_POINT ( 'NONE',  ( -35.27139336136212933, 24.82964151130203945, 177.5919119679930134 ) ) ;
#81412=AXIS2_PLACEMENT_3D ( 'NONE', #17069, #16573, #57064 ) ;
#81413=FACE_OUTER_BOUND ( 'NONE', #90981, .T. ) ;
#81415=EDGE_CURVE ( 'NONE', #81073, #83731, #31683, .T. ) ;
#81431=EDGE_CURVE ( 'NONE', #32592, #26456, #16504, .T. ) ;
#81439=CARTESIAN_POINT ( 'NONE',  ( 48.58805178314242568, 84.67719436603331928, -10.00000000000000000 ) ) ;
#81446=DIRECTION ( 'NONE',  ( 1.000000000000000000, 0.000000000000000000, 0.000000000000000000 ) ) ;
#81448=DIRECTION ( 'NONE',  ( 0.7440200784635646603, 0.6681572590663601430, 0.000000000000000000 ) ) ;
#81454=ORIENTED_EDGE ( 'NONE', *, *, #13247, .T. ) ;
#81460=PLANE ( 'NONE',  #93941 ) ;
#81469=ORIENTED_EDGE ( 'NONE', *, *, #46783, .T. ) ;
#81477=EDGE_CURVE ( 'NONE', #56511, #21034, #37141, .T. ) ;
#81487=VECTOR ( 'NONE', #73306, 1000.000000000000000 ) ;
#81490=ORIENTED_EDGE ( 'NONE', *, *, #69772, .T. ) ;
#81494=CYLINDRICAL_SURFACE ( 'NONE', #28151, 70.00000000000002842 ) ;
#81495=DIRECTION ( 'NONE',  ( 0.000000000000000000, 0.000000000000000000, 1.000000000000000000 ) ) ;
#81497=AXIS2_PLACEMENT_3D ( 'NONE', #68803, #45989, #67824 ) ;
#81503=DIRECTION ( 'NONE',  ( -0.000000000000000000, 0.000000000000000000, 1.000000000000000000 ) ) ;
#81507=ORIENTED_EDGE ( 'NONE', *, *, #79651, .F. ) ;
#81514=VERTEX_POINT ( 'NONE', #97053 ) ;
#81517=ORIENTED_EDGE ( 'NONE', *, *, #49835, .F. ) ;
#81538=CARTESIAN_POINT ( 'NONE',  ( -37.40701240123934213, 25.35389310390295137, 10.00000000000000000 ) ) ;
#81550=CARTESIAN_POINT ( 'NONE',  ( 38.90713690219553200, 54.71539658304152454, -10.00000000000000000 ) ) ;
#81552=CARTESIAN_POINT ( 'NONE',  ( 49.10122569834316408, 93.29622288527660601, -10.00000000000000000 ) ) ;
#81553=ADVANCED_FACE ( 'NONE', ( #43287 ), #5309, .F. ) ;
#81554=CIRCLE ( 'NONE', #97731, 0.1418229129680828593 ) ;
#81558=VECTOR ( 'NONE', #39293, 999.9999999999998863 ) ;
#81572=CARTESIAN_POINT ( 'NONE',  ( -34.16292631813981728, 25.86630820016799248, 10.00000000000000000 ) ) ;
#81580=ORIENTED_EDGE ( 'NONE', *, *, #24112, .T. ) ;
#81582=EDGE_LOOP ( 'NONE', ( #19005, #13314, #29570, #76129 ) ) ;
#81586=ORIENTED_EDGE ( 'NONE', *, *, #62011, .F. ) ;
#81589=DIRECTION ( 'NONE',  ( 1.000000000000000000, 7.930164461608259453E-16, 0.000000000000000000 ) ) ;
#81592=DIRECTION ( 'NONE',  ( 0.000000000000000000, -0.000000000000000000, -1.000000000000000000 ) ) ;
#81596=DIRECTION ( 'NONE',  ( -0.6544109481086123337, -0.7561390817803210762, 0.000000000000000000 ) ) ;
#81598=PLANE ( 'NONE',  #32695 ) ;
#81603=CARTESIAN_POINT ( 'NONE',  ( -40.14225747417106760, 26.13077817479420872, -10.00000000000000000 ) ) ;
#81604=VERTEX_POINT ( 'NONE', #77579 ) ;
#81610=FACE_OUTER_BOUND ( 'NONE', #18123, .T. ) ;
#81615=CYLINDRICAL_SURFACE ( 'NONE', #97445, 49.99999999999999289 ) ;
#81617=ORIENTED_EDGE ( 'NONE', *, *, #95627, .F. ) ;
#81619=VERTEX_POINT ( 'NONE', #94796 ) ;
#81621=FACE_BOUND ( 'NONE', #40286, .T. ) ;
#81634=CARTESIAN_POINT ( 'NONE',  ( 47.05668214639808156, 76.45164061169337799, 10.00000000000000000 ) ) ;
#81638=CARTESIAN_POINT ( 'NONE',  ( 44.08135397534552169, 118.8355609772188188, -10.00000000000000000 ) ) ;
#81642=CIRCLE ( 'NONE', #88171, 70.00000000000001421 ) ;
#81643=LINE ( 'NONE', #82152, #73678 ) ;
#81655=DIRECTION ( 'NONE',  ( -1.000000000000000000, 0.000000000000000000, 0.000000000000000000 ) ) ;
#81656=ORIENTED_EDGE ( 'NONE', *, *, #77673, .F. ) ;
#81694=DIRECTION ( 'NONE',  ( 0.03277852384265239616, -0.9994626398093610087, 0.000000000000000000 ) ) ;
#81696=VECTOR ( 'NONE', #91347, 1000.000000000000000 ) ;
#81709=DIRECTION ( 'NONE',  ( -0.000000000000000000, -0.000000000000000000, 1.000000000000000000 ) ) ;
#81714=DIRECTION ( 'NONE',  ( -0.000000000000000000, -0.000000000000000000, -1.000000000000000000 ) ) ;
#81716=ORIENTED_EDGE ( 'NONE', *, *, #67191, .F. ) ;
#81719=ORIENTED_EDGE ( 'NONE', *, *, #52413, .T. ) ;
#81736=EDGE_CURVE ( 'NONE', #63400, #32826, #88220, .T. ) ;
#81738=AXIS2_PLACEMENT_3D ( 'NONE', #90828, #6675, #61849 ) ;
#81739=ORIENTED_EDGE ( 'NONE', *, *, #59213, .T. ) ;
#81742=CYLINDRICAL_SURFACE ( 'NONE', #15392, 70.00000000000002842 ) ;
#81746=ORIENTED_EDGE ( 'NONE', *, *, #82570, .T. ) ;
#81749=CARTESIAN_POINT ( 'NONE',  ( -19.65312891409030271, 93.06504152958497400, 177.5919119679930134 ) ) ;
#81750=ORIENTED_EDGE ( 'NONE', *, *, #74547, .F. ) ;
#81751=CARTESIAN_POINT ( 'NONE',  ( 48.98810889288134263, 89.24608170897542436, 10.00000000000000000 ) ) ;
#81753=FACE_OUTER_BOUND ( 'NONE', #54483, .T. ) ;
#81769=CARTESIAN_POINT ( 'NONE',  ( -71.61465314115659453, 63.06504152958490295, -10.00000000000000888 ) ) ;
#81770=LINE ( 'NONE', #35125, #11757 ) ;
#81771=CIRCLE ( 'NONE', #89870, 70.00000000000001421 ) ;
#81782=( GEOMETRIC_REPRESENTATION_CONTEXT ( 3 ) GLOBAL_UNCERTAINTY_ASSIGNED_CONTEXT ( ( #95000 ) ) GLOBAL_UNIT_ASSIGNED_CONTEXT ( ( #76207, #84324, #61468 ) ) REPRESENTATION_CONTEXT ( 'NONE', 'WORKASPACE' ) );
#81789=EDGE_LOOP ( 'NONE', ( #1871, #45587, #15923, #78589 ) ) ;
#81790=VERTEX_POINT ( 'NONE', #64870 ) ;
#81791=LINE ( 'NONE', #63682, #81885 ) ;
#81795=CARTESIAN_POINT ( 'NONE',  ( -11.70629829599211646, 23.25616956148705938, -10.00000000000000000 ) ) ;
#81799=CARTESIAN_POINT ( 'NONE',  ( -62.95439910331221256, 68.06504152958493137, 25.00000000000000000 ) ) ;
#81804=EDGE_CURVE ( 'NONE', #38056, #74380, #11289, .T. ) ;
#81805=DIRECTION ( 'NONE',  ( -0.000000000000000000, 0.000000000000000000, -1.000000000000000000 ) ) ;
#81806=CARTESIAN_POINT ( 'NONE',  ( 23.64814127513154673, 118.0650415295851019, -20.00000000000000355 ) ) ;
#81807=VECTOR ( 'NONE', #34635, 1000.000000000000227 ) ;
#81810=DIRECTION ( 'NONE',  ( 0.000000000000000000, 0.000000000000000000, 1.000000000000000000 ) ) ;
#81826=LINE ( 'NONE', #51374, #63019 ) ;
#81837=CARTESIAN_POINT ( 'NONE',  ( 49.83874514172082826, 101.4840343560034057, 177.5919119679930134 ) ) ;
#81844=CARTESIAN_POINT ( 'NONE',  ( 19.18375657693640335, 36.32959363016014720, -10.00000000000000000 ) ) ;
#81845=VERTEX_POINT ( 'NONE', #89708 ) ;
#81850=CARTESIAN_POINT ( 'NONE',  ( -19.65312891409030271, 93.06504152958497400, 10.00000000000000888 ) ) ;
#81852=ORIENTED_EDGE ( 'NONE', *, *, #43882, .T. ) ;
#81857=DIRECTION ( 'NONE',  ( 0.000000000000000000, 0.000000000000000000, 1.000000000000000000 ) ) ;
#81864=ORIENTED_EDGE ( 'NONE', *, *, #16727, .T. ) ;
#81876=CARTESIAN_POINT ( 'NONE',  ( 45.11483101423407049, 69.99284853207299761, -10.00000000000000000 ) ) ;
#81879=CARTESIAN_POINT ( 'NONE',  ( 32.30839531297598910, 123.0650415295850593, 25.00000000000000000 ) ) ;
#81885=VECTOR ( 'NONE', #17584, 1000.000000000000341 ) ;
#81888=EDGE_LOOP ( 'NONE', ( #41299, #90194, #29873, #54535 ) ) ;
#81889=DIRECTION ( 'NONE',  ( -0.000000000000000000, -0.000000000000000000, -1.000000000000000000 ) ) ;
#81908=CARTESIAN_POINT ( 'NONE',  ( -20.01016364259690405, 23.06595206263087050, 10.00000000000000000 ) ) ;
#81911=VERTEX_POINT ( 'NONE', #9048 ) ;
#81912=CIRCLE ( 'NONE', #17138, 45.00000000000000000 ) ;
#81914=ADVANCED_FACE ( 'NONE', ( #84587 ), #61732, .F. ) ;
#81915=CARTESIAN_POINT ( 'NONE',  ( -16.99542894172669349, 24.36904009834038476, 10.00000000000000000 ) ) ;
#81920=PLANE ( 'NONE',  #6498 ) ;
#81945=VECTOR ( 'NONE', #25155, 1000.000000000000114 ) ;
#81952=AXIS2_PLACEMENT_3D ( 'NONE', #84987, #6469, #46432 ) ;
#81956=VECTOR ( 'NONE', #52435, 1000.000000000000000 ) ;
#81967=ORIENTED_EDGE ( 'NONE', *, *, #62181, .F. ) ;
#81970=EDGE_LOOP ( 'NONE', ( #66437, #89995, #824, #62615 ) ) ;
#81972=ORIENTED_EDGE ( 'NONE', *, *, #14634, .F. ) ;
#81975=DIRECTION ( 'NONE',  ( -0.000000000000000000, 0.000000000000000000, -1.000000000000000000 ) ) ;
#81980=VECTOR ( 'NONE', #27, 1000.000000000000114 ) ;
#81982=AXIS2_PLACEMENT_3D ( 'NONE', #77992, #95230, #981 ) ;
#81984=EDGE_CURVE ( 'NONE', #92543, #23591, #8058, .T. ) ;
#82008=ORIENTED_EDGE ( 'NONE', *, *, #25303, .T. ) ;
#82010=ADVANCED_FACE ( 'NONE', ( #77465 ), #93686, .T. ) ;
#82016=EDGE_CURVE ( 'NONE', #8241, #49563, #69837, .T. ) ;
#82028=CARTESIAN_POINT ( 'NONE',  ( 29.41244916810467203, 42.77587997571678358, -10.00000000000000000 ) ) ;
#82030=VECTOR ( 'NONE', #89721, 1000.000000000000114 ) ;
#82041=EDGE_CURVE ( 'NONE', #6796, #7444, #62224, .T. ) ;
#82048=ADVANCED_FACE ( 'NONE', ( #37759 ), #37272, .T. ) ;
#82049=VECTOR ( 'NONE', #59546, 1000.000000000000114 ) ;
#82059=LINE ( 'NONE', #27812, #84942 ) ;
#82060=PLANE ( 'NONE',  #65665 ) ;
#82062=DIRECTION ( 'NONE',  ( 0.9041295198386993803, -0.4272584830711297910, 0.000000000000000000 ) ) ;
#82068=DIRECTION ( 'NONE',  ( -0.6066398774942428629, 0.7949767663484071933, 0.000000000000000000 ) ) ;
#82079=CARTESIAN_POINT ( 'NONE',  ( 47.49582885874516336, 78.29235751436857527, -10.00000000000000000 ) ) ;
#82082=FACE_OUTER_BOUND ( 'NONE', #67635, .T. ) ;
#82083=DIRECTION ( 'NONE',  ( -0.1237105541964931971, 0.9923183454821323801, 0.000000000000000000 ) ) ;
#82085=CARTESIAN_POINT ( 'NONE',  ( 39.64431452495995245, 58.26521502737223557, -10.00000000000000000 ) ) ;
#82096=DIRECTION ( 'NONE',  ( -1.000000000000000000, 0.000000000000000000, 0.000000000000000000 ) ) ;
#82103=VECTOR ( 'NONE', #53636, 1000.000000000000114 ) ;
#82108=VERTEX_POINT ( 'NONE', #61055 ) ;
#82110=CARTESIAN_POINT ( 'NONE',  ( 39.64431452495995245, 58.26521502737223557, -10.00000000000000000 ) ) ;
#82113=VERTEX_POINT ( 'NONE', #28676 ) ;
#82114=AXIS2_PLACEMENT_3D ( 'NONE', #75013, #75507, #20311 ) ;
#82116=LINE ( 'NONE', #35461, #60447 ) ;
#82120=DIRECTION ( 'NONE',  ( -0.1963739994383708332, 0.9805290675673918876, 0.000000000000000000 ) ) ;
#82124=ADVANCED_FACE ( 'NONE', ( #38247 ), #44860, .F. ) ;
#82128=CIRCLE ( 'NONE', #85379, 70.00000000000001421 ) ;
#82132=FACE_BOUND ( 'NONE', #88581, .T. ) ;
#82136=EDGE_CURVE ( 'NONE', #14010, #52870, #91022, .T. ) ;
#82138=DIRECTION ( 'NONE',  ( -1.000000000000000000, 0.000000000000000000, 0.000000000000000000 ) ) ;
#82152=CARTESIAN_POINT ( 'NONE',  ( 50.30020549591840506, 90.50945844122863093, 177.5919119679930134 ) ) ;
#82155=DIRECTION ( 'NONE',  ( -0.000000000000000000, -0.000000000000000000, -1.000000000000000000 ) ) ;
#82161=LINE ( 'NONE', #12736, #15943 ) ;
#82166=DIRECTION ( 'NONE',  ( 1.000000000000000000, 0.000000000000000000, 0.000000000000000000 ) ) ;
#82172=EDGE_CURVE ( 'NONE', #41966, #30353, #9693, .T. ) ;
#82180=CARTESIAN_POINT ( 'NONE',  ( 7.864685750751951865, 30.05722773587472929, 10.00000000000000000 ) ) ;
#82206=FACE_OUTER_BOUND ( 'NONE', #83242, .T. ) ;
#82207=VECTOR ( 'NONE', #52475, 1000.000000000000000 ) ;
#82214=DIRECTION ( 'NONE',  ( -0.5696381972391070247, 0.8218955677251095215, 0.000000000000000000 ) ) ;
#82235=ORIENTED_EDGE ( 'NONE', *, *, #31520, .T. ) ;
#82241=CIRCLE ( 'NONE', #90336, 70.00000000000001421 ) ;
#82248=CIRCLE ( 'NONE', #100070, 70.00000000000001421 ) ;
#82253=ORIENTED_EDGE ( 'NONE', *, *, #91376, .F. ) ;
#82257=EDGE_CURVE ( 'NONE', #19564, #89238, #85415, .T. ) ;
#82259=ORIENTED_EDGE ( 'NONE', *, *, #24549, .F. ) ;
#82262=ORIENTED_EDGE ( 'NONE', *, *, #16346, .F. ) ;
#82263=AXIS2_PLACEMENT_3D ( 'NONE', #98020, #59478, #36190 ) ;
#82265=FACE_OUTER_BOUND ( 'NONE', #32060, .T. ) ;
#82267=CARTESIAN_POINT ( 'NONE',  ( 19.39689925177878749, 34.96947112835012916, 10.00000000000000000 ) ) ;
#82269=LINE ( 'NONE', #3252, #22451 ) ;
#82271=CIRCLE ( 'NONE', #27269, 0.1418229129681557177 ) ;
#82280=ORIENTED_EDGE ( 'NONE', *, *, #70651, .F. ) ;
#82283=DIRECTION ( 'NONE',  ( 1.000000000000000000, 0.000000000000000000, 0.000000000000000000 ) ) ;
#82289=CIRCLE ( 'NONE', #11101, 70.00000000000001421 ) ;
#82290=EDGE_CURVE ( 'NONE', #82431, #39405, #31151, .T. ) ;
#82303=ORIENTED_EDGE ( 'NONE', *, *, #90573, .T. ) ;
#82314=VECTOR ( 'NONE', #74686, 1000.000000000000000 ) ;
#82317=AXIS2_PLACEMENT_3D ( 'NONE', #73943, #43005, #65817 ) ;
#82329=PLANE ( 'NONE',  #18241 ) ;
#82330=LINE ( 'NONE', #50369, #2989 ) ;
#82331=DIRECTION ( 'NONE',  ( 0.000000000000000000, 0.000000000000000000, 1.000000000000000000 ) ) ;
#82333=VERTEX_POINT ( 'NONE', #96019 ) ;
#82336=DIRECTION ( 'NONE',  ( -0.6778389383370750920, -0.7352104281592222179, 0.000000000000000000 ) ) ;
#82341=FACE_OUTER_BOUND ( 'NONE', #18017, .T. ) ;
#82342=DIRECTION ( 'NONE',  ( 0.9991767892008865948, 0.04056776950002415755, 0.000000000000000000 ) ) ;
#82345=EDGE_LOOP ( 'NONE', ( #46048, #94314, #97902, #48044 ) ) ;
#82351=VECTOR ( 'NONE', #6628, 1000.000000000000114 ) ;
#82360=ORIENTED_EDGE ( 'NONE', *, *, #81062, .F. ) ;
#82361=PLANE ( 'NONE',  #128 ) ;
#82364=ORIENTED_EDGE ( 'NONE', *, *, #73774, .T. ) ;
#82372=EDGE_CURVE ( 'NONE', #89979, #27077, #26581, .T. ) ;
#82373=DIRECTION ( 'NONE',  ( -0.8321961394790272637, 0.5544813661758195567, 0.000000000000000000 ) ) ;
#82379=ORIENTED_EDGE ( 'NONE', *, *, #96899, .T. ) ;
#82380=VERTEX_POINT ( 'NONE', #88435 ) ;
#82389=ORIENTED_EDGE ( 'NONE', *, *, #72640, .F. ) ;
#82397=VECTOR ( 'NONE', #58934, 1000.000000000000000 ) ;
#82400=ORIENTED_EDGE ( 'NONE', *, *, #19660, .F. ) ;
#82403=AXIS2_PLACEMENT_3D ( 'NONE', #42385, #91034, #22587 ) ;
#82408=ORIENTED_EDGE ( 'NONE', *, *, #41367, .F. ) ;
#82410=CARTESIAN_POINT ( 'NONE',  ( 37.07881409725408162, 81.27343214090025469, 59.99999999999999289 ) ) ;
#82413=DIRECTION ( 'NONE',  ( -1.000000000000000000, 0.000000000000000000, 0.000000000000000000 ) ) ;
#82417=VECTOR ( 'NONE', #86357, 1000.000000000000000 ) ;
#82431=VERTEX_POINT ( 'NONE', #72062 ) ;
#82434=DIRECTION ( 'NONE',  ( 0.000000000000000000, -0.000000000000000000, -1.000000000000000000 ) ) ;
#82448=EDGE_CURVE ( 'NONE', #68842, #15749, #2661, .T. ) ;
#82450=CARTESIAN_POINT ( 'NONE',  ( 47.89168550319194395, 74.68847913791599069, -10.00000000000000000 ) ) ;
#82458=LINE ( 'NONE', #83931, #75621 ) ;
#82472=LINE ( 'NONE', #14986, #29673 ) ;
#82475=FACE_OUTER_BOUND ( 'NONE', #32268, .T. ) ;
#82477=DIRECTION ( 'NONE',  ( 0.000000000000000000, -0.000000000000000000, -1.000000000000000000 ) ) ;
#82482=AXIS2_PLACEMENT_3D ( 'NONE', #11678, #58732, #65357 ) ;
#82486=ORIENTED_EDGE ( 'NONE', *, *, #910, .F. ) ;
#82489=ORIENTED_EDGE ( 'NONE', *, *, #87771, .F. ) ;
#82490=DIRECTION ( 'NONE',  ( 0.000000000000000000, 0.000000000000000000, 1.000000000000000000 ) ) ;
#82498=CARTESIAN_POINT ( 'NONE',  ( -78.24550368024017644, 54.29179893118896416, -10.00000000000000000 ) ) ;
#82505=VERTEX_POINT ( 'NONE', #23315 ) ;
#82511=CYLINDRICAL_SURFACE ( 'NONE', #5302, 70.00000000000002842 ) ;
#82513=DIRECTION ( 'NONE',  ( -0.000000000000000000, -0.000000000000000000, -1.000000000000000000 ) ) ;
#82529=VERTEX_POINT ( 'NONE', #23815 ) ;
#82533=VECTOR ( 'NONE', #30502, 1000.000000000000000 ) ;
#82557=VECTOR ( 'NONE', #34697, 1000.000000000000114 ) ;
#82560=CARTESIAN_POINT ( 'NONE',  ( 50.27371054362190961, 89.86549102125590593, -10.00000000000000000 ) ) ;
#82570=EDGE_CURVE ( 'NONE', #50852, #16524, #14523, .T. ) ;
#82591=ORIENTED_EDGE ( 'NONE', *, *, #49742, .F. ) ;
#82593=VERTEX_POINT ( 'NONE', #24331 ) ;
#82596=AXIS2_PLACEMENT_3D ( 'NONE', #96164, #42888, #95686 ) ;
#82597=CARTESIAN_POINT ( 'NONE',  ( -48.71813016832984289, 30.75580926756359901, 10.00000000000000000 ) ) ;
#82599=DIRECTION ( 'NONE',  ( 0.8660254037844379305, 0.5000000000000011102, 0.000000000000000000 ) ) ;
#82606=ORIENTED_EDGE ( 'NONE', *, *, #68326, .F. ) ;
#82614=CARTESIAN_POINT ( 'NONE',  ( -2.073866539663252073, 26.60322154129610794, -10.00000000000000000 ) ) ;
#82621=CARTESIAN_POINT ( 'NONE',  ( -19.65312891409030271, 93.06504152958497400, 10.00000000000000888 ) ) ;
#82629=EDGE_CURVE ( 'NONE', #48601, #30838, #72955, .T. ) ;
#82633=CARTESIAN_POINT ( 'NONE',  ( 30.80155721116056355, 46.36891074996812989, -10.00000000000000000 ) ) ;
#82639=EDGE_CURVE ( 'NONE', #41570, #17465, #72455, .T. ) ;
#82641=CARTESIAN_POINT ( 'NONE',  ( 15.36455789491911794, 32.15369338429142942, 10.00000000000000000 ) ) ;
#82653=VERTEX_POINT ( 'NONE', #29321 ) ;
#82661=ORIENTED_EDGE ( 'NONE', *, *, #41742, .T. ) ;
#82662=DIRECTION ( 'NONE',  ( -0.8098206029991052990, 0.5866775868892262213, 0.000000000000000000 ) ) ;
#82668=DIRECTION ( 'NONE',  ( -0.000000000000000000, -0.000000000000000000, -1.000000000000000000 ) ) ;
#82670=DIRECTION ( 'NONE',  ( -0.5866775868892349921, -0.8098206029990988597, 0.000000000000000000 ) ) ;
#82681=DIRECTION ( 'NONE',  ( -0.000000000000000000, 0.000000000000000000, 1.000000000000000000 ) ) ;
#82689=EDGE_CURVE ( 'NONE', #1959, #35128, #69540, .T. ) ;
#82698=LINE ( 'NONE', #7631, #96038 ) ;
#82703=EDGE_CURVE ( 'NONE', #43568, #33103, #68278, .T. ) ;
#82711=LINE ( 'NONE', #36045, #90271 ) ;
#82714=DIRECTION ( 'NONE',  ( 0.000000000000000000, 0.000000000000000000, 1.000000000000000000 ) ) ;
#82731=ORIENTED_EDGE ( 'NONE', *, *, #65948, .F. ) ;
#82733=EDGE_CURVE ( 'NONE', #48909, #62608, #29301, .T. ) ;
#82734=FACE_OUTER_BOUND ( 'NONE', #65378, .T. ) ;
#82735=DIRECTION ( 'NONE',  ( -1.000000000000000000, 0.000000000000000000, 0.000000000000000000 ) ) ;
#82737=ORIENTED_EDGE ( 'NONE', *, *, #85698, .F. ) ;
#82742=CARTESIAN_POINT ( 'NONE',  ( 49.42830306794131445, 81.76213237698445369, 177.5919119679930134 ) ) ;
#82743=EDGE_CURVE ( 'NONE', #62710, #47438, #22692, .T. ) ;
#82744=ADVANCED_FACE ( 'NONE', ( #99697 ), #13599, .T. ) ;
#82748=ADVANCED_FACE ( 'NONE', ( #15069 ), #69776, .T. ) ;
#82749=CARTESIAN_POINT ( 'NONE',  ( -52.57320609282758994, 32.70376883311633520, 10.00000000000000000 ) ) ;
#82750=ORIENTED_EDGE ( 'NONE', *, *, #52881, .T. ) ;
#82753=ORIENTED_EDGE ( 'NONE', *, *, #96333, .T. ) ;
#82754=FACE_OUTER_BOUND ( 'NONE', #16048, .T. ) ;
#82756=ORIENTED_EDGE ( 'NONE', *, *, #21827, .F. ) ;
#82757=VECTOR ( 'NONE', #26522, 1000.000000000000000 ) ;
#82760=CARTESIAN_POINT ( 'NONE',  ( -19.65312891409030271, 93.06504152958497400, 59.99999999999999289 ) ) ;
#82774=ORIENTED_EDGE ( 'NONE', *, *, #78927, .F. ) ;
#82794=DIRECTION ( 'NONE',  ( -1.000000000000000000, 0.000000000000000000, 0.000000000000000000 ) ) ;
#82798=CARTESIAN_POINT ( 'NONE',  ( -61.64759997997268925, 36.73658404823907375, 10.00000000000000000 ) ) ;
#82818=CARTESIAN_POINT ( 'NONE',  ( -19.65312891409030271, 93.06504152958497400, 59.99999999999999289 ) ) ;
#82820=ORIENTED_EDGE ( 'NONE', *, *, #64377, .T. ) ;
#82822=VECTOR ( 'NONE', #71230, 1000.000000000000000 ) ;
#82824=CARTESIAN_POINT ( 'NONE',  ( 49.10122569834318540, 93.29622288527660601, -10.00000000000000000 ) ) ;
#82832=CARTESIAN_POINT ( 'NONE',  ( 17.60357497223980516, 35.28838536716092023, 10.00000000000000000 ) ) ;
#82846=CARTESIAN_POINT ( 'NONE',  ( 22.72264919896475988, 37.02287747747012503, 10.00000000000000000 ) ) ;
#82856=CARTESIAN_POINT ( 'NONE',  ( -76.23101443460923576, 54.01191295053621388, 10.00000000000000000 ) ) ;
#82861=CARTESIAN_POINT ( 'NONE',  ( 19.12011368430507829, 34.47266676343468106, 10.00000000000000000 ) ) ;
#82873=ORIENTED_EDGE ( 'NONE', *, *, #8469, .T. ) ;
#82878=CARTESIAN_POINT ( 'NONE',  ( 47.49582885874516336, 78.29235751436857527, 10.00000000000000000 ) ) ;
#82884=EDGE_CURVE ( 'NONE', #76991, #82653, #50166, .T. ) ;
#82893=FACE_OUTER_BOUND ( 'NONE', #74894, .T. ) ;
#82906=FACE_OUTER_BOUND ( 'NONE', #84709, .T. ) ;
#82911=ORIENTED_EDGE ( 'NONE', *, *, #62981, .F. ) ;
#82912=CARTESIAN_POINT ( 'NONE',  ( -23.29562891409031522, 78.77562236714182120, 59.99999999999999289 ) ) ;
#82914=CARTESIAN_POINT ( 'NONE',  ( -6.887318171848119341, 24.23892674679882475, 177.5919119679930134 ) ) ;
#82918=CARTESIAN_POINT ( 'NONE',  ( -19.65312891409030271, 93.06504152958497400, 10.00000000000000888 ) ) ;
#82922=CARTESIAN_POINT ( 'NONE',  ( 12.00096474099108690, 32.03863464977599307, -10.00000000000000000 ) ) ;
#82931=DIRECTION ( 'NONE',  ( 0.000000000000000000, 0.000000000000000000, 1.000000000000000000 ) ) ;
#82932=ADVANCED_FACE ( 'NONE', ( #11995 ), #81920, .F. ) ;
#82933=DIRECTION ( 'NONE',  ( -0.5372068985985170020, -0.8434505012732892437, 0.000000000000000000 ) ) ;
#82935=CARTESIAN_POINT ( 'NONE',  ( 48.81784752633560487, 86.82484054835779830, -10.00000000000000000 ) ) ;
#82936=EDGE_CURVE ( 'NONE', #38602, #90969, #43363, .T. ) ;
#82938=EDGE_CURVE ( 'NONE', #22359, #55654, #3406, .T. ) ;
#82942=CARTESIAN_POINT ( 'NONE',  ( 9.684647596568824568, 42.25052203202275081, 59.99999999999999289 ) ) ;
#82961=CARTESIAN_POINT ( 'NONE',  ( 1.813001633210440611, 27.74720351945397923, -10.00000000000000000 ) ) ;
#82968=DIRECTION ( 'NONE',  ( -1.000000000000000000, 0.000000000000000000, 0.000000000000000000 ) ) ;
#82969=VERTEX_POINT ( 'NONE', #80940 ) ;
#82972=CARTESIAN_POINT ( 'NONE',  ( -19.65312891409030271, 93.06504152958497400, 10.00000000000000888 ) ) ;
#82981=CARTESIAN_POINT ( 'NONE',  ( 46.80963145949300497, 71.09457308843315104, -10.00000000000000000 ) ) ;
#82995=ORIENTED_EDGE ( 'NONE', *, *, #19434, .F. ) ;
#82996=CARTESIAN_POINT ( 'NONE',  ( 0.9561933761060431580, 66.99251067065806353, -10.00000000000000000 ) ) ;
#83000=VECTOR ( 'NONE', #76203, 1000.000000000000227 ) ;
#83001=AXIS2_PLACEMENT_3D ( 'NONE', #26491, #32584, #25480 ) ;
#83010=ORIENTED_EDGE ( 'NONE', *, *, #50238, .F. ) ;
#83014=EDGE_CURVE ( 'NONE', #8310, #18075, #45355, .T. ) ;
#83016=CARTESIAN_POINT ( 'NONE',  ( -40.67952639183666008, 27.60432558407080350, -10.00000000000000000 ) ) ;
#83040=CYLINDRICAL_SURFACE ( 'NONE', #9321, 70.00000000000002842 ) ;
#83044=CARTESIAN_POINT ( 'NONE',  ( -69.61464189717713680, 45.83092310410449244, -10.00000000000000000 ) ) ;
#83057=LINE ( 'NONE', #59709, #84737 ) ;
#83060=CARTESIAN_POINT ( 'NONE',  ( -19.65312891409034179, 93.06504152958504505, 0.000000000000000000 ) ) ;
#83065=CIRCLE ( 'NONE', #94421, 0.1418229129681564116 ) ;
#83075=ORIENTED_EDGE ( 'NONE', *, *, #53591, .T. ) ;
#83078=CARTESIAN_POINT ( 'NONE',  ( 23.64814127513158937, 118.0650415295850451, 60.00000000000000000 ) ) ;
#83079=VERTEX_POINT ( 'NONE', #91013 ) ;
#83080=VECTOR ( 'NONE', #72978, 1000.000000000000114 ) ;
#83083=DIRECTION ( 'NONE',  ( -0.000000000000000000, -0.000000000000000000, -1.000000000000000000 ) ) ;
#83085=DIRECTION ( 'NONE',  ( -0.000000000000000000, -0.000000000000000000, 1.000000000000000000 ) ) ;
#83092=ORIENTED_EDGE ( 'NONE', *, *, #37215, .T. ) ;
#83097=CARTESIAN_POINT ( 'NONE',  ( -18.30488606758875392, 59.85806527642789376, -10.00000000000000000 ) ) ;
#83105=DIRECTION ( 'NONE',  ( -0.3958915996110536351, -0.9182972510888840478, 0.000000000000000000 ) ) ;
#83106=ORIENTED_EDGE ( 'NONE', *, *, #9716, .T. ) ;
#83109=EDGE_CURVE ( 'NONE', #60766, #97433, #92018, .T. ) ;
#83110=ORIENTED_EDGE ( 'NONE', *, *, #21544, .T. ) ;
#83111=PLANE ( 'NONE',  #13743 ) ;
#83112=EDGE_LOOP ( 'NONE', ( #46649, #10660, #41510, #81337 ) ) ;
#83121=ORIENTED_EDGE ( 'NONE', *, *, #42236, .T. ) ;
#83125=EDGE_LOOP ( 'NONE', ( #63146, #78082, #45909, #12969 ) ) ;
#83127=EDGE_CURVE ( 'NONE', #3988, #86151, #21099, .T. ) ;
#83141=DIRECTION ( 'NONE',  ( -0.9599109957006544125, -0.2803049773603353279, 0.000000000000000000 ) ) ;
#83145=AXIS2_PLACEMENT_3D ( 'NONE', #40755, #34183, #71705 ) ;
#83150=VECTOR ( 'NONE', #6648, 1000.000000000000114 ) ;
#83156=EDGE_CURVE ( 'NONE', #19346, #47682, #7353, .T. ) ;
#83168=CARTESIAN_POINT ( 'NONE',  ( -19.65312891409030271, 93.06504152958497400, 59.99999999999999289 ) ) ;
#83173=CARTESIAN_POINT ( 'NONE',  ( -52.24036053731629892, 86.53868222403792743, -10.00000000000000000 ) ) ;
#83189=DIRECTION ( 'NONE',  ( 0.000000000000000000, 0.000000000000000000, 1.000000000000000000 ) ) ;
#83202=DIRECTION ( 'NONE',  ( -0.8756465943326185997, -0.4829524219151267728, 0.000000000000000000 ) ) ;
#83206=DIRECTION ( 'NONE',  ( -0.000000000000000000, 0.000000000000000000, -1.000000000000000000 ) ) ;
#83210=ORIENTED_EDGE ( 'NONE', *, *, #61054, .T. ) ;
#83211=ORIENTED_EDGE ( 'NONE', *, *, #55878, .F. ) ;
#83220=DIRECTION ( 'NONE',  ( -0.000000000000000000, 0.000000000000000000, 1.000000000000000000 ) ) ;
#83229=ORIENTED_EDGE ( 'NONE', *, *, #35895, .F. ) ;
#83233=ORIENTED_EDGE ( 'NONE', *, *, #91858, .F. ) ;
#83239=ADVANCED_FACE ( 'NONE', ( #8615 ), #29914, .F. ) ;
#83242=EDGE_LOOP ( 'NONE', ( #90224, #84156, #53857, #13373 ) ) ;
#83246=CARTESIAN_POINT ( 'NONE',  ( 49.83874514172083536, 101.4840343560033915, 10.00000000000000000 ) ) ;
#83247=CARTESIAN_POINT ( 'NONE',  ( -46.96828164281857454, 74.13349478725223207, -10.00000000000000000 ) ) ;
#83250=ORIENTED_EDGE ( 'NONE', *, *, #24339, .T. ) ;
#83254=ADVANCED_FACE ( 'NONE', ( #45596 ), #23298, .F. ) ;
#83257=EDGE_CURVE ( 'NONE', #95321, #69469, #80958, .T. ) ;
#83262=CARTESIAN_POINT ( 'NONE',  ( -19.65312891409030271, 93.06504152958497400, 60.00000000000000000 ) ) ;
#83268=CARTESIAN_POINT ( 'NONE',  ( 20.67738335769525904, 35.85097175740956033, 177.5919119679930134 ) ) ;
#83272=CARTESIAN_POINT ( 'NONE',  ( 41.71240375114938814, 62.05720181600818108, -10.00000000000000000 ) ) ;
#83273=ORIENTED_EDGE ( 'NONE', *, *, #10268, .F. ) ;
#83278=LINE ( 'NONE', #44230, #31923 ) ;
#83281=VECTOR ( 'NONE', #97246, 1000.000000000000000 ) ;
#83282=CARTESIAN_POINT ( 'NONE',  ( -72.81784413424506397, 47.52919789448971244, 177.5919119679930134 ) ) ;
#83284=CARTESIAN_POINT ( 'NONE',  ( 6.117390533544194930, 29.33055864014943026, -10.00000000000000000 ) ) ;
#83291=EDGE_CURVE ( 'NONE', #31851, #21922, #39482, .T. ) ;
#83304=DIRECTION ( 'NONE',  ( -0.4831861483251571610, -0.8755176446347036068, 0.000000000000000000 ) ) ;
#83306=CARTESIAN_POINT ( 'NONE',  ( -36.52772323645827868, 26.41323893245353105, -10.00000000000000000 ) ) ;
#83308=ORIENTED_EDGE ( 'NONE', *, *, #1628, .F. ) ;
#83323=FACE_OUTER_BOUND ( 'NONE', #53314, .T. ) ;
#83330=LINE ( 'NONE', #53863, #34436 ) ;
#83335=DIRECTION ( 'NONE',  ( -0.000000000000000000, 0.000000000000000000, -1.000000000000000000 ) ) ;
#83338=EDGE_LOOP ( 'NONE', ( #80031, #80924, #95692, #36966 ) ) ;
#83340=CARTESIAN_POINT ( 'NONE',  ( 32.30839531297598910, 123.0650415295850593, 203.6502102582797420 ) ) ;
#83342=ORIENTED_EDGE ( 'NONE', *, *, #94957, .F. ) ;
#83347=DIRECTION ( 'NONE',  ( -0.03304531753666253152, -0.9994538543569188027, 0.000000000000000000 ) ) ;
#83349=ORIENTED_EDGE ( 'NONE', *, *, #37774, .T. ) ;
#83355=ORIENTED_EDGE ( 'NONE', *, *, #23835, .T. ) ;
#83358=CARTESIAN_POINT ( 'NONE',  ( -38.35373792487678202, 26.90998726756845727, -10.00000000000000000 ) ) ;
#83359=ORIENTED_EDGE ( 'NONE', *, *, #34570, .F. ) ;
#83365=CYLINDRICAL_SURFACE ( 'NONE', #89991, 70.00000000000002842 ) ;
#83367=VECTOR ( 'NONE', #26959, 1000.000000000000000 ) ;
#83374=ORIENTED_EDGE ( 'NONE', *, *, #18453, .T. ) ;
#83377=ORIENTED_EDGE ( 'NONE', *, *, #13487, .F. ) ;
#83383=FACE_OUTER_BOUND ( 'NONE', #40061, .T. ) ;
#83398=CIRCLE ( 'NONE', #34762, 70.00000000000001421 ) ;
#83401=ORIENTED_EDGE ( 'NONE', *, *, #69637, .T. ) ;
#83402=DIRECTION ( 'NONE',  ( 0.000000000000000000, 0.000000000000000000, 1.000000000000000000 ) ) ;
#83421=DIRECTION ( 'NONE',  ( -0.000000000000000000, -0.000000000000000000, -1.000000000000000000 ) ) ;
#83422=DIRECTION ( 'NONE',  ( -0.9834470158338919354, -0.1811959355157079787, 0.000000000000000000 ) ) ;
#83423=ADVANCED_FACE ( 'NONE', ( #11732 ), #74030, .F. ) ;
#83426=LINE ( 'NONE', #74325, #51323 ) ;
#83429=CARTESIAN_POINT ( 'NONE',  ( 48.38981961164312651, 109.5014996615669105, 177.5919119679930134 ) ) ;
#83453=EDGE_CURVE ( 'NONE', #88645, #46305, #5608, .T. ) ;
#83458=ORIENTED_EDGE ( 'NONE', *, *, #53579, .F. ) ;
#83461=EDGE_CURVE ( 'NONE', #81157, #93052, #74540, .T. ) ;
#83466=LINE ( 'NONE', #46917, #81558 ) ;
#83471=VECTOR ( 'NONE', #64041, 1000.000000000000000 ) ;
#83479=CARTESIAN_POINT ( 'NONE',  ( -0.4668637173180778532, 25.74574839753307387, 10.00000000000000000 ) ) ;
#83482=LINE ( 'NONE', #76831, #26092 ) ;
#83492=EDGE_LOOP ( 'NONE', ( #24951, #46509, #84722, #91110 ) ) ;
#83496=ORIENTED_EDGE ( 'NONE', *, *, #93701, .T. ) ;
#83497=AXIS2_PLACEMENT_3D ( 'NONE', #50960, #66174, #88042 ) ;
#83503=ADVANCED_FACE ( 'NONE', ( #97832 ), #75030, .T. ) ;
#83505=ORIENTED_EDGE ( 'NONE', *, *, #58915, .T. ) ;
#83509=ORIENTED_EDGE ( 'NONE', *, *, #51571, .F. ) ;
#83511=ORIENTED_EDGE ( 'NONE', *, *, #25003, .F. ) ;
#83539=VECTOR ( 'NONE', #36133, 1000.000000000000000 ) ;
#83545=LINE ( 'NONE', #14108, #73431 ) ;
#83547=DIRECTION ( 'NONE',  ( -0.9140770918436990078, -0.4055404667435369426, 0.000000000000000000 ) ) ;
#83552=LINE ( 'NONE', #67305, #99389 ) ;
#83556=ADVANCED_FACE ( 'NONE', ( #13710 ), #20831, .T. ) ;
#83561=DIRECTION ( 'NONE',  ( -0.7646402761590023189, -0.6444573283588950208, 0.000000000000000000 ) ) ;
#83564=AXIS2_PLACEMENT_3D ( 'NONE', #95848, #85761, #1101 ) ;
#83565=VERTEX_POINT ( 'NONE', #36500 ) ;
#83570=PLANE ( 'NONE',  #9605 ) ;
#83576=VERTEX_POINT ( 'NONE', #67403 ) ;
#83584=CARTESIAN_POINT ( 'NONE',  ( 19.31801425620940194, 115.5650415295850451, 60.00000000000000000 ) ) ;
#83595=ORIENTED_EDGE ( 'NONE', *, *, #45378, .T. ) ;
#83596=DIRECTION ( 'NONE',  ( 0.000000000000000000, 0.000000000000000000, 1.000000000000000000 ) ) ;
#83597=CARTESIAN_POINT ( 'NONE',  ( -19.65312891409030271, 93.06504152958497400, 177.5919119679930134 ) ) ;
#83607=VERTEX_POINT ( 'NONE', #50214 ) ;
#83610=VECTOR ( 'NONE', #31740, 1000.000000000000227 ) ;
#83612=LINE ( 'NONE', #14180, #44602 ) ;
#83613=AXIS2_PLACEMENT_3D ( 'NONE', #67767, #84498, #53546 ) ;
#83623=EDGE_CURVE ( 'NONE', #22484, #99081, #4111, .T. ) ;
#83628=EDGE_CURVE ( 'NONE', #66038, #62710, #97143, .T. ) ;
#83631=ADVANCED_FACE ( 'NONE', ( #26925 ), #88783, .T. ) ;
#83632=ORIENTED_EDGE ( 'NONE', *, *, #74008, .T. ) ;
#83634=EDGE_CURVE ( 'NONE', #22359, #34967, #96863, .T. ) ;
#83635=CARTESIAN_POINT ( 'NONE',  ( 15.11407551230992219, 32.30945333909093620, 10.00000000000000000 ) ) ;
#83640=LINE ( 'NONE', #75510, #41572 ) ;
#83643=AXIS2_PLACEMENT_3D ( 'NONE', #25929, #24904, #25406 ) ;
#83671=VERTEX_POINT ( 'NONE', #19830 ) ;
#83677=CIRCLE ( 'NONE', #31850, 70.00000000000001421 ) ;
#83683=VECTOR ( 'NONE', #19187, 999.9999999999998863 ) ;
#83687=EDGE_CURVE ( 'NONE', #78482, #50533, #89759, .T. ) ;
#83692=DIRECTION ( 'NONE',  ( -0.6201213960746242426, 0.7845058662180030007, 0.000000000000000000 ) ) ;
#83693=EDGE_CURVE ( 'NONE', #98005, #7924, #91737, .T. ) ;
#83697=CARTESIAN_POINT ( 'NONE',  ( -38.02969130575858969, 25.52022711230254615, 177.5919119679930134 ) ) ;
#83708=DIRECTION ( 'NONE',  ( 0.000000000000000000, 0.000000000000000000, 1.000000000000000000 ) ) ;
#83716=ORIENTED_EDGE ( 'NONE', *, *, #29214, .F. ) ;
#83720=DIRECTION ( 'NONE',  ( 0.000000000000000000, 0.000000000000000000, 1.000000000000000000 ) ) ;
#83731=VERTEX_POINT ( 'NONE', #60773 ) ;
#83734=DIRECTION ( 'NONE',  ( 1.000000000000000000, 0.000000000000000000, 0.000000000000000000 ) ) ;
#83736=LINE ( 'NONE', #76124, #51414 ) ;
#83738=CARTESIAN_POINT ( 'NONE',  ( 23.64814127513158937, 118.0650415295850451, 60.00000000000000000 ) ) ;
#83740=VERTEX_POINT ( 'NONE', #99321 ) ;
#83747=EDGE_CURVE ( 'NONE', #98547, #26987, #22300, .T. ) ;
#83749=EDGE_CURVE ( 'NONE', #11268, #28252, #29203, .T. ) ;
#83750=CARTESIAN_POINT ( 'NONE',  ( -19.65312891409030271, 93.06504152958497400, 10.00000000000000888 ) ) ;
#83751=LINE ( 'NONE', #35617, #2764 ) ;
#83752=VECTOR ( 'NONE', #45579, 999.9999999999998863 ) ;
#83756=CARTESIAN_POINT ( 'NONE',  ( 25.98835327777827686, 41.64452202306098627, -10.00000000000000000 ) ) ;
#83760=CARTESIAN_POINT ( 'NONE',  ( 48.48788556946983874, 102.1758113618167982, -10.00000000000000000 ) ) ;
#83774=LINE ( 'NONE', #98953, #98012 ) ;
#83775=CARTESIAN_POINT ( 'NONE',  ( 24.19030146973739193, 38.49624447322263876, -10.00000000000000000 ) ) ;
#83779=LINE ( 'NONE', #37620, #33345 ) ;
#83781=VERTEX_POINT ( 'NONE', #23286 ) ;
#83785=LINE ( 'NONE', #45235, #85602 ) ;
#83789=CIRCLE ( 'NONE', #46563, 70.00000000000001421 ) ;
#83791=ORIENTED_EDGE ( 'NONE', *, *, #63015, .F. ) ;
#83807=CARTESIAN_POINT ( 'NONE',  ( -54.21831688459418785, 33.63902229265146104, -10.00000000000000000 ) ) ;
#83809=ORIENTED_EDGE ( 'NONE', *, *, #79482, .T. ) ;
#83815=EDGE_CURVE ( 'NONE', #91193, #67048, #81034, .T. ) ;
#83816=CARTESIAN_POINT ( 'NONE',  ( 38.04107491472452551, 53.42442038713602415, -10.00000000000000000 ) ) ;
#83823=AXIS2_PLACEMENT_3D ( 'NONE', #38837, #353, #62126 ) ;
#83840=FACE_OUTER_BOUND ( 'NONE', #6055, .T. ) ;
#83845=PLANE ( 'NONE',  #88850 ) ;
#83848=CARTESIAN_POINT ( 'NONE',  ( -30.18034446749236821, 25.12100238203590763, -10.00000000000000000 ) ) ;
#83860=ORIENTED_EDGE ( 'NONE', *, *, #13294, .T. ) ;
#83861=EDGE_CURVE ( 'NONE', #85923, #63494, #3031, .T. ) ;
#83863=VERTEX_POINT ( 'NONE', #1005 ) ;
#83867=DIRECTION ( 'NONE',  ( -0.000000000000000000, -0.000000000000000000, -1.000000000000000000 ) ) ;
#83868=EDGE_LOOP ( 'NONE', ( #25266, #97299, #97188, #88777 ) ) ;
#83881=DIRECTION ( 'NONE',  ( 0.000000000000000000, 0.000000000000000000, 1.000000000000000000 ) ) ;
#83883=EDGE_CURVE ( 'NONE', #87907, #38349, #48609, .T. ) ;
#83891=ORIENTED_EDGE ( 'NONE', *, *, #33756, .T. ) ;
#83893=VECTOR ( 'NONE', #95403, 1000.000000000000114 ) ;
#83900=VECTOR ( 'NONE', #14934, 1000.000000000000000 ) ;
#83905=EDGE_LOOP ( 'NONE', ( #49079, #31738, #18978, #64564 ) ) ;
#83906=AXIS2_PLACEMENT_3D ( 'NONE', #43693, #13321, #28492 ) ;
#83913=VECTOR ( 'NONE', #31979, 1000.000000000000227 ) ;
#83919=CARTESIAN_POINT ( 'NONE',  ( -29.91485116994501325, 25.08783183303773967, 10.00000000000000000 ) ) ;
#83921=AXIS2_PLACEMENT_3D ( 'NONE', #55908, #36116, #3266 ) ;
#83926=DIRECTION ( 'NONE',  ( 1.000000000000000000, 1.962715704248044129E-13, 0.000000000000000000 ) ) ;
#83931=CARTESIAN_POINT ( 'NONE',  ( -47.78078991586325230, 28.96484896693081978, 177.5919119679930134 ) ) ;
#83944=AXIS2_PLACEMENT_3D ( 'NONE', #51982, #13497, #29188 ) ;
#83948=ORIENTED_EDGE ( 'NONE', *, *, #70921, .T. ) ;
#83952=EDGE_CURVE ( 'NONE', #44815, #6582, #39975, .T. ) ;
#83962=ORIENTED_EDGE ( 'NONE', *, *, #86968, .F. ) ;
#83965=ORIENTED_EDGE ( 'NONE', *, *, #47322, .T. ) ;
#83969=VECTOR ( 'NONE', #29948, 1000.000000000000114 ) ;
#83979=CARTESIAN_POINT ( 'NONE',  ( -19.65312891409030271, 93.06504152958497400, 10.00000000000000888 ) ) ;
#83984=CARTESIAN_POINT ( 'NONE',  ( 47.05668214639808156, 76.45164061169337799, -10.00000000000000000 ) ) ;
#83986=AXIS2_PLACEMENT_3D ( 'NONE', #55042, #78880, #47445 ) ;
#83987=EDGE_CURVE ( 'NONE', #61495, #72257, #45377, .T. ) ;
#83989=CARTESIAN_POINT ( 'NONE',  ( 40.48539884740148409, 126.3902902409112556, -10.00000000000000000 ) ) ;
#84002=CARTESIAN_POINT ( 'NONE',  ( 23.64814127513158226, 118.0650415295850451, -20.00000000000000355 ) ) ;
#84006=CIRCLE ( 'NONE', #61302, 70.00000000000001421 ) ;
#84007=ORIENTED_EDGE ( 'NONE', *, *, #62394, .F. ) ;
#84010=ADVANCED_FACE ( 'NONE', ( #19227 ), #89171, .F. ) ;
#84012=CARTESIAN_POINT ( 'NONE',  ( 42.33744422746375591, 122.7866300363639169, 10.00000000000000000 ) ) ;
#84018=CARTESIAN_POINT ( 'NONE',  ( -41.40204166758637427, 67.93526189084366251, -10.00000000000000000 ) ) ;
#84035=CYLINDRICAL_SURFACE ( 'NONE', #89980, 70.00000000000002842 ) ;
#84039=AXIS2_PLACEMENT_3D ( 'NONE', #84371, #6342, #76731 ) ;
#84043=LINE ( 'NONE', #45480, #13970 ) ;
#84045=VECTOR ( 'NONE', #60064, 1000.000000000000114 ) ;
#84063=ADVANCED_FACE ( 'NONE', ( #36378 ), #18710, .T. ) ;
#84079=EDGE_CURVE ( 'NONE', #8947, #76337, #50097, .T. ) ;
#84080=DIRECTION ( 'NONE',  ( -0.000000000000000000, -0.000000000000000000, 1.000000000000000000 ) ) ;
#84091=ORIENTED_EDGE ( 'NONE', *, *, #48834, .F. ) ;
#84092=CARTESIAN_POINT ( 'NONE',  ( -71.61465314115659453, 63.06504152958490295, -60.00000000000000000 ) ) ;
#84106=ORIENTED_EDGE ( 'NONE', *, *, #25046, .T. ) ;
#84117=CIRCLE ( 'NONE', #79194, 70.00000000000001421 ) ;
#84121=ORIENTED_EDGE ( 'NONE', *, *, #96190, .F. ) ;
#84122=CARTESIAN_POINT ( 'NONE',  ( 41.50249547274756878, 124.4848494355456836, 10.00000000000000000 ) ) ;
#84123=DIRECTION ( 'NONE',  ( 1.000000000000000000, 0.000000000000000000, 0.000000000000000000 ) ) ;
#84124=ORIENTED_EDGE ( 'NONE', *, *, #28639, .F. ) ;
#84126=CARTESIAN_POINT ( 'NONE',  ( -19.65312891409030271, 93.06504152958497400, 59.99999999999999289 ) ) ;
#84129=FACE_BOUND ( 'NONE', #21049, .T. ) ;
#84137=ORIENTED_EDGE ( 'NONE', *, *, #70293, .F. ) ;
#84140=CARTESIAN_POINT ( 'NONE',  ( -34.16292631813981728, 25.86630820016799248, -10.00000000000000000 ) ) ;
#84147=LINE ( 'NONE', #15170, #33490 ) ;
#84156=ORIENTED_EDGE ( 'NONE', *, *, #23307, .T. ) ;
#84164=CARTESIAN_POINT ( 'NONE',  ( -19.65312891409030271, 93.06504152958497400, 177.5919119679930134 ) ) ;
#84170=CARTESIAN_POINT ( 'NONE',  ( -13.42108286626701030, 23.34301056334150104, 177.5919119679930134 ) ) ;
#84175=DIRECTION ( 'NONE',  ( 0.9819794923402651587, -0.1889875038809575580, 0.000000000000000000 ) ) ;
#84191=EDGE_CURVE ( 'NONE', #32399, #36317, #63179, .T. ) ;
#84192=AXIS2_PLACEMENT_3D ( 'NONE', #22803, #53682, #92732 ) ;
#84202=DIRECTION ( 'NONE',  ( -0.000000000000000000, -0.000000000000000000, -1.000000000000000000 ) ) ;
#84211=ORIENTED_EDGE ( 'NONE', *, *, #50727, .F. ) ;
#84216=VERTEX_POINT ( 'NONE', #65543 ) ;
#84224=DIRECTION ( 'NONE',  ( 0.000000000000000000, 0.000000000000000000, 1.000000000000000000 ) ) ;
#84231=ORIENTED_EDGE ( 'NONE', *, *, #9958, .F. ) ;
#84233=VERTEX_POINT ( 'NONE', #2267 ) ;
#84240=CARTESIAN_POINT ( 'NONE',  ( -18.15312891409030627, 78.77562236714182120, 13.81405534229504894 ) ) ;
#84241=CARTESIAN_POINT ( 'NONE',  ( -19.65312891409030271, 93.06504152958497400, 60.00000000000000000 ) ) ;
#84251=DIRECTION ( 'NONE',  ( -0.2639761180675095353, 0.9645292162967424865, 0.000000000000000000 ) ) ;
#84268=VECTOR ( 'NONE', #67094, 1000.000000000000000 ) ;
#84274=EDGE_CURVE ( 'NONE', #1103, #95115, #79304, .T. ) ;
#84283=B_SPLINE_CURVE_WITH_KNOTS ( 'NONE', 3,
 ( #40530, #40023, #1052, #32449, #23331, #71465, #57726, #10657, #10157, #95310, #42038, #2565, #4538, #87225, #11171, #25865, #33449, #79593, #41023, #64345, #96791, #41533, #26851, #19761, #97274, #81096, #80090, #34930, #56741, #17759, #27351, #49636, #57231, #71961, #88706, #3564, #87723, #64855, #19276, #18259, #50629, #72973, #88207 ),
 .UNSPECIFIED., .F., .F.,
 ( 4, 2, 2, 2, 2, 2, 1, 2, 2, 2, 2, 2, 2, 2, 2, 2, 2, 2, 2, 2, 2, 4 ),
 ( 0.000000000000000000, 0.001338277739954425337, 0.002007416609931637896, 0.002676555479908850673, 0.004014833219863313957, 0.004683972089840546249, 0.005353110959817779409, 0.006022249829795012568, 0.006691388699772244861, 0.008029666439726690363, 0.008698805309703908778, 0.009367944179681128927, 0.01070622191963556749, 0.01204449965959000259, 0.01271363852956721753, 0.01338277739954443248, 0.01472105513949887971, 0.01605933287945332175, 0.01739761061940776551, 0.01873588835936220928, 0.02007416609931665652, 0.02141244383927110029 ),
 .UNSPECIFIED. ) ;
#84284=ORIENTED_EDGE ( 'NONE', *, *, #36694, .T. ) ;
#84287=CARTESIAN_POINT ( 'NONE',  ( 23.64814127513154673, 118.0650415295851019, -45.00000000000000711 ) ) ;
#84293=DIRECTION ( 'NONE',  ( 1.000000000000000000, -1.687142489207157240E-13, 0.000000000000000000 ) ) ;
#84294=EDGE_LOOP ( 'NONE', ( #88230, #57207, #61116, #12461 ) ) ;
#84302=LINE ( 'NONE', #92397, #18418 ) ;
#84309=EDGE_LOOP ( 'NONE', ( #35586, #97910, #6322, #57115 ) ) ;
#84316=EDGE_CURVE ( 'NONE', #87203, #8463, #73172, .T. ) ;
#84318=CARTESIAN_POINT ( 'NONE',  ( -78.57153713424665398, 57.64153020465174393, -10.00000000000000000 ) ) ;
#84322=ORIENTED_EDGE ( 'NONE', *, *, #23322, .T. ) ;
#84323=CARTESIAN_POINT ( 'NONE',  ( -19.65312891409030271, 93.06504152958497400, -10.00000000000000888 ) ) ;
#84324=( NAMED_UNIT ( * ) PLANE_ANGLE_UNIT ( ) SI_UNIT ( $, .RADIAN. ) );
#84325=CARTESIAN_POINT ( 'NONE',  ( -19.73679784724330588, 93.17955462170891678, 59.99999999999999289 ) ) ;
#84333=DIRECTION ( 'NONE',  ( -0.9972444261165168689, 0.07418594597050684469, 0.000000000000000000 ) ) ;
#84338=DIRECTION ( 'NONE',  ( -1.000000000000000000, 0.000000000000000000, 0.000000000000000000 ) ) ;
#84344=EDGE_LOOP ( 'NONE', ( #64271, #22245, #96841, #23384 ) ) ;
#84349=ORIENTED_EDGE ( 'NONE', *, *, #85808, .T. ) ;
#84355=ORIENTED_EDGE ( 'NONE', *, *, #33767, .F. ) ;
#84356=ORIENTED_EDGE ( 'NONE', *, *, #11993, .F. ) ;
#84365=DIRECTION ( 'NONE',  ( -0.8325133752583718794, 0.5540049458406605121, 0.000000000000000000 ) ) ;
#84371=CARTESIAN_POINT ( 'NONE',  ( 48.48788556946983874, 102.1758113618167982, -10.00000000000000000 ) ) ;
#84376=DIRECTION ( 'NONE',  ( -1.000000000000000000, 0.000000000000000000, 0.000000000000000000 ) ) ;
#84380=ORIENTED_EDGE ( 'NONE', *, *, #3423, .T. ) ;
#84399=LINE ( 'NONE', #24550, #25946 ) ;
#84401=VECTOR ( 'NONE', #62448, 1000.000000000000000 ) ;
#84425=ORIENTED_EDGE ( 'NONE', *, *, #76416, .F. ) ;
#84428=CARTESIAN_POINT ( 'NONE',  ( 42.45923888023187232, 122.5484010731363043, 10.00000000000000000 ) ) ;
#84433=CARTESIAN_POINT ( 'NONE',  ( 10.06845959268932411, 31.07446838803123157, 10.00000000000000000 ) ) ;
#84438=CARTESIAN_POINT ( 'NONE',  ( -73.66720466879952767, 50.53642055324488069, -10.00000000000000000 ) ) ;
#84457=VERTEX_POINT ( 'NONE', #17567 ) ;
#84464=VERTEX_POINT ( 'NONE', #93601 ) ;
#84465=DIRECTION ( 'NONE',  ( 0.000000000000000000, 0.000000000000000000, 1.000000000000000000 ) ) ;
#84466=DIRECTION ( 'NONE',  ( 0.000000000000000000, -0.000000000000000000, -1.000000000000000000 ) ) ;
#84475=ORIENTED_EDGE ( 'NONE', *, *, #52413, .F. ) ;
#84476=EDGE_LOOP ( 'NONE', ( #81133, #27741, #55843, #71638 ) ) ;
#84480=CARTESIAN_POINT ( 'NONE',  ( -25.62627769214124740, 24.57763045674671432, -10.00000000000000000 ) ) ;
#84497=EDGE_CURVE ( 'NONE', #48849, #58283, #27695, .T. ) ;
#84498=DIRECTION ( 'NONE',  ( -0.000000000000000000, -0.000000000000000000, 1.000000000000000000 ) ) ;
#84504=ORIENTED_EDGE ( 'NONE', *, *, #41478, .T. ) ;
#84505=FACE_OUTER_BOUND ( 'NONE', #70617, .T. ) ;
#84507=ORIENTED_EDGE ( 'NONE', *, *, #47205, .F. ) ;
#84509=EDGE_CURVE ( 'NONE', #3476, #33732, #89521, .T. ) ;
#84515=VECTOR ( 'NONE', #54356, 1000.000000000000000 ) ;
#84517=EDGE_LOOP ( 'NONE', ( #5101, #18045, #32722, #59592 ) ) ;
#84520=CARTESIAN_POINT ( 'NONE',  ( -77.74869931532472833, 54.01501336371526918, 177.5919119679930134 ) ) ;
#84524=EDGE_CURVE ( 'NONE', #68842, #78966, #36746, .T. ) ;
#84525=DIRECTION ( 'NONE',  ( 0.3653410243663972601, 0.9308737486442033582, 0.000000000000000000 ) ) ;
#84532=FACE_OUTER_BOUND ( 'NONE', #90087, .T. ) ;
#84540=EDGE_CURVE ( 'NONE', #24915, #30767, #6363, .T. ) ;
#84551=DIRECTION ( 'NONE',  ( -0.4245406647209920559, -0.9054088711727195093, 0.000000000000000000 ) ) ;
#84564=EDGE_CURVE ( 'NONE', #73603, #49393, #95642, .T. ) ;
#84572=ORIENTED_EDGE ( 'NONE', *, *, #24408, .F. ) ;
#84573=LINE ( 'NONE', #54107, #89455 ) ;
#84583=LINE ( 'NONE', #6552, #50552 ) ;
#84584=VECTOR ( 'NONE', #9403, 1000.000000000000114 ) ;
#84585=EDGE_LOOP ( 'NONE', ( #79761, #44818, #46707, #80851 ) ) ;
#84587=FACE_OUTER_BOUND ( 'NONE', #54659, .T. ) ;
#84588=LINE ( 'NONE', #91682, #45613 ) ;
#84592=ORIENTED_EDGE ( 'NONE', *, *, #8556, .T. ) ;
#84596=CARTESIAN_POINT ( 'NONE',  ( -19.65312891409030271, 93.06504152958497400, 45.00000000000000711 ) ) ;
#84602=VECTOR ( 'NONE', #24226, 1000.000000000000114 ) ;
#84605=ORIENTED_EDGE ( 'NONE', *, *, #69177, .F. ) ;
#84608=CARTESIAN_POINT ( 'NONE',  ( -16.25778278694858514, 23.14743555886465032, -10.00000000000000000 ) ) ;
#84613=FACE_BOUND ( 'NONE', #15512, .T. ) ;
#84622=ORIENTED_EDGE ( 'NONE', *, *, #11273, .T. ) ;
#84630=ORIENTED_EDGE ( 'NONE', *, *, #14349, .F. ) ;
#84635=ADVANCED_FACE ( 'NONE', ( #71170 ), #54939, .F. ) ;
#84642=DIRECTION ( 'NONE',  ( -0.4554470513245731378, -0.8902628732232696906, 0.000000000000000000 ) ) ;
#84646=ORIENTED_EDGE ( 'NONE', *, *, #99469, .F. ) ;
#84649=VECTOR ( 'NONE', #93650, 1000.000000000000000 ) ;
#84656=DIRECTION ( 'NONE',  ( 1.000000000000000000, 0.000000000000000000, 0.000000000000000000 ) ) ;
#84657=DIRECTION ( 'NONE',  ( 0.000000000000000000, 0.000000000000000000, 1.000000000000000000 ) ) ;
#84658=EDGE_CURVE ( 'NONE', #91719, #100031, #7339, .T. ) ;
#84661=ORIENTED_EDGE ( 'NONE', *, *, #71141, .T. ) ;
#84662=VECTOR ( 'NONE', #29107, 1000.000000000000227 ) ;
#84664=ADVANCED_FACE ( 'NONE', ( #86407, #84885 ), #78763, .F. ) ;
#84676=EDGE_CURVE ( 'NONE', #42808, #39213, #32646, .T. ) ;
#84697=VERTEX_POINT ( 'NONE', #63045 ) ;
#84700=DIRECTION ( 'NONE',  ( 0.000000000000000000, 0.000000000000000000, 1.000000000000000000 ) ) ;
#84702=ORIENTED_EDGE ( 'NONE', *, *, #90559, .F. ) ;
#84707=CARTESIAN_POINT ( 'NONE',  ( -36.52772323645827868, 26.41323893245353105, 10.00000000000000000 ) ) ;
#84709=EDGE_LOOP ( 'NONE', ( #71613, #14794, #54347, #28614 ) ) ;
#84711=( LENGTH_UNIT ( ) NAMED_UNIT ( * ) SI_UNIT ( .MILLI., .METRE. ) );
#84722=ORIENTED_EDGE ( 'NONE', *, *, #11582, .F. ) ;
#84725=ORIENTED_EDGE ( 'NONE', *, *, #52233, .F. ) ;
#84727=PLANE ( 'NONE',  #59537 ) ;
#84728=VERTEX_POINT ( 'NONE', #249 ) ;
#84730=CARTESIAN_POINT ( 'NONE',  ( -5.530696300892750550, 75.41849186590253851, 14.61344814751857868 ) ) ;
#84734=EDGE_LOOP ( 'NONE', ( #21382, #31970, #36467, #47466 ) ) ;
#84735=ORIENTED_EDGE ( 'NONE', *, *, #38578, .F. ) ;
#84737=VECTOR ( 'NONE', #36408, 1000.000000000000000 ) ;
#84746=CARTESIAN_POINT ( 'NONE',  ( 49.93482446054090218, 85.48106202472366988, 177.5919119679930134 ) ) ;
#84747=FACE_OUTER_BOUND ( 'NONE', #10854, .T. ) ;
#84756=ADVANCED_FACE ( 'NONE', ( #7855 ), #47338, .F. ) ;
#84761=ORIENTED_EDGE ( 'NONE', *, *, #94717, .T. ) ;
#84765=EDGE_CURVE ( 'NONE', #23591, #41972, #98018, .T. ) ;
#84769=DIRECTION ( 'NONE',  ( 1.000000000000000000, 0.000000000000000000, 0.000000000000000000 ) ) ;
#84778=CARTESIAN_POINT ( 'NONE',  ( -19.65312891409030271, 93.06504152958497400, 10.00000000000000888 ) ) ;
#84783=ADVANCED_FACE ( 'NONE', ( #96553 ), #82361, .F. ) ;
#84785=DIRECTION ( 'NONE',  ( -0.5000000000000012212, 0.8660254037844379305, -0.000000000000000000 ) ) ;
#84786=ORIENTED_EDGE ( 'NONE', *, *, #74081, .T. ) ;
#84792=LINE ( 'NONE', #70546, #99885 ) ;
#84800=ORIENTED_EDGE ( 'NONE', *, *, #17566, .T. ) ;
#84801=AXIS2_PLACEMENT_3D ( 'NONE', #61623, #6934, #54013 ) ;
#84809=VECTOR ( 'NONE', #86119, 1000.000000000000114 ) ;
#84813=ORIENTED_EDGE ( 'NONE', *, *, #16877, .F. ) ;
#84820=ORIENTED_EDGE ( 'NONE', *, *, #83952, .T. ) ;
#84826=CYLINDRICAL_SURFACE ( 'NONE', #36405, 70.00000000000002842 ) ;
#84833=VERTEX_POINT ( 'NONE', #97530 ) ;
#84837=VERTEX_POINT ( 'NONE', #80867 ) ;
#84841=DIRECTION ( 'NONE',  ( -1.000000000000000000, 0.000000000000000000, 0.000000000000000000 ) ) ;
#84845=DIRECTION ( 'NONE',  ( 1.000000000000000000, 0.000000000000000000, 0.000000000000000000 ) ) ;
#84849=VERTEX_POINT ( 'NONE', #27625 ) ;
#84866=DIRECTION ( 'NONE',  ( 0.000000000000000000, -0.000000000000000000, -1.000000000000000000 ) ) ;
#84876=EDGE_CURVE ( 'NONE', #15552, #43154, #90457, .T. ) ;
#84885=FACE_OUTER_BOUND ( 'NONE', #1958, .T. ) ;
#84892=ORIENTED_EDGE ( 'NONE', *, *, #45017, .T. ) ;
#84895=DIRECTION ( 'NONE',  ( -0.000000000000000000, -0.000000000000000000, -1.000000000000000000 ) ) ;
#84907=DIRECTION ( 'NONE',  ( 1.000000000000000000, 0.000000000000000000, 0.000000000000000000 ) ) ;
#84918=VERTEX_POINT ( 'NONE', #43790 ) ;
#84924=CARTESIAN_POINT ( 'NONE',  ( 40.37736971981244238, 56.55791953817036699, -10.00000000000000000 ) ) ;
#84931=CARTESIAN_POINT ( 'NONE',  ( 29.12701137275935181, 44.61184105132205957, -10.00000000000000000 ) ) ;
#84932=FACE_OUTER_BOUND ( 'NONE', #66656, .T. ) ;
#84939=ORIENTED_EDGE ( 'NONE', *, *, #21239, .F. ) ;
#84942=VECTOR ( 'NONE', #58687, 1000.000000000000227 ) ;
#84944=ADVANCED_FACE ( 'NONE', ( #53386 ), #60978, .T. ) ;
#84945=LINE ( 'NONE', #53500, #45246 ) ;
#84947=ORIENTED_EDGE ( 'NONE', *, *, #77158, .T. ) ;
#84952=EDGE_CURVE ( 'NONE', #38602, #17814, #195, .T. ) ;
#84953=LINE ( 'NONE', #25106, #58048 ) ;
#84954=AXIS2_PLACEMENT_3D ( 'NONE', #61877, #46693, #31984 ) ;
#84955=ORIENTED_EDGE ( 'NONE', *, *, #68907, .T. ) ;
#84961=LINE ( 'NONE', #85475, #29190 ) ;
#84967=VERTEX_POINT ( 'NONE', #15882 ) ;
#84969=ORIENTED_EDGE ( 'NONE', *, *, #44193, .T. ) ;
#84982=ORIENTED_EDGE ( 'NONE', *, *, #76953, .F. ) ;
#84983=VECTOR ( 'NONE', #70702, 1000.000000000000114 ) ;
#84987=CARTESIAN_POINT ( 'NONE',  ( 17.26055046206296950, 33.28368158147418399, -10.00000000000000000 ) ) ;
#84994=ORIENTED_EDGE ( 'NONE', *, *, #55658, .T. ) ;
#84996=DIRECTION ( 'NONE',  ( -0.000000000000000000, -0.000000000000000000, 1.000000000000000000 ) ) ;
#84997=ORIENTED_EDGE ( 'NONE', *, *, #43100, .T. ) ;
#84999=EDGE_CURVE ( 'NONE', #92184, #1733, #76694, .T. ) ;
#85000=ADVANCED_FACE ( 'NONE', ( #83840 ), #13899, .F. ) ;
#85005=LINE ( 'NONE', #98704, #25821 ) ;
#85012=DIRECTION ( 'NONE',  ( 0.05364311403569549386, 0.9985601716053735810, 0.000000000000000000 ) ) ;
#85013=CARTESIAN_POINT ( 'NONE',  ( -41.73592930317598615, 44.85821161687699998, 59.99999999999999289 ) ) ;
#85016=AXIS2_PLACEMENT_3D ( 'NONE', #36083, #18929, #11336 ) ;
#85018=LINE ( 'NONE', #85537, #20385 ) ;
#85023=CARTESIAN_POINT ( 'NONE',  ( 41.25821923120311396, 128.0827283385945918, -10.00000000000000000 ) ) ;
#85043=CARTESIAN_POINT ( 'NONE',  ( -42.47074677134371257, 28.21475011077167139, -10.00000000000000000 ) ) ;
#85046=EDGE_CURVE ( 'NONE', #68592, #17528, #14405, .T. ) ;
#85049=CARTESIAN_POINT ( 'NONE',  ( -78.10577900106846982, 54.55156729251706338, 10.00000000000000000 ) ) ;
#85052=LINE ( 'NONE', #76909, #28679 ) ;
#85058=VECTOR ( 'NONE', #64914, 1000.000000000000114 ) ;
#85061=LINE ( 'NONE', #69819, #50697 ) ;
#85063=ORIENTED_EDGE ( 'NONE', *, *, #57842, .F. ) ;
#85069=EDGE_CURVE ( 'NONE', #10423, #74959, #16319, .T. ) ;
#85071=ORIENTED_EDGE ( 'NONE', *, *, #30850, .F. ) ;
#85076=DIRECTION ( 'NONE',  ( 0.000000000000000000, 0.000000000000000000, -1.000000000000000000 ) ) ;
#85082=EDGE_CURVE ( 'NONE', #49707, #44730, #62466, .T. ) ;
#85084=CARTESIAN_POINT ( 'NONE',  ( 0.5143710859096835009, 78.77562236714182120, 59.99999999999999289 ) ) ;
#85089=VERTEX_POINT ( 'NONE', #47772 ) ;
#85090=LINE ( 'NONE', #8064, #45921 ) ;
#85104=EDGE_LOOP ( 'NONE', ( #44204, #46829, #88929, #90210 ) ) ;
#85106=VERTEX_POINT ( 'NONE', #93432 ) ;
#85108=ADVANCED_FACE ( 'NONE', ( #1199 ), #9296, .F. ) ;
#85117=EDGE_CURVE ( 'NONE', #60349, #39911, #40522, .T. ) ;
#85120=ORIENTED_EDGE ( 'NONE', *, *, #90559, .T. ) ;
#85123=EDGE_CURVE ( 'NONE', #79865, #8628, #18409, .T. ) ;
#85126=AXIS2_PLACEMENT_3D ( 'NONE', #5008, #35887, #51593 ) ;
#85142=EDGE_LOOP ( 'NONE', ( #12192, #57062, #35269, #85401 ) ) ;
#85151=AXIS2_PLACEMENT_3D ( 'NONE', #60666, #75923, #76883 ) ;
#85159=DIRECTION ( 'NONE',  ( -0.000000000000000000, -0.000000000000000000, -1.000000000000000000 ) ) ;
#85164=CARTESIAN_POINT ( 'NONE',  ( 10.06845959268932411, 31.07446838803123157, -10.00000000000000000 ) ) ;
#85181=PLANE ( 'NONE',  #18332 ) ;
#85184=PLANE ( 'NONE',  #30989 ) ;
#85187=EDGE_CURVE ( 'NONE', #70849, #27171, #24421, .T. ) ;
#85199=VECTOR ( 'NONE', #64798, 1000.000000000000000 ) ;
#85204=ORIENTED_EDGE ( 'NONE', *, *, #1583, .T. ) ;
#85208=DIRECTION ( 'NONE',  ( -0.000000000000000000, -0.000000000000000000, -1.000000000000000000 ) ) ;
#85215=ORIENTED_EDGE ( 'NONE', *, *, #14071, .T. ) ;
#85217=DIRECTION ( 'NONE',  ( 0.9708212084269294273, -0.2398044646550112069, 0.000000000000000000 ) ) ;
#85222=DIRECTION ( 'NONE',  ( 0.000000000000000000, 0.000000000000000000, 1.000000000000000000 ) ) ;
#85223=VERTEX_POINT ( 'NONE', #74616 ) ;
#85224=DIRECTION ( 'NONE',  ( -0.000000000000000000, 0.000000000000000000, 1.000000000000000000 ) ) ;
#85225=VECTOR ( 'NONE', #59905, 1000.000000000000000 ) ;
#85231=ORIENTED_EDGE ( 'NONE', *, *, #393, .F. ) ;
#85232=CARTESIAN_POINT ( 'NONE',  ( -4.696717224021703885, 77.89375390941042099, 14.01032106654459142 ) ) ;
#85236=AXIS2_PLACEMENT_3D ( 'NONE', #83060, #14627, #23206 ) ;
#85238=ORIENTED_EDGE ( 'NONE', *, *, #97792, .T. ) ;
#85241=CARTESIAN_POINT ( 'NONE',  ( -11.70629829599211646, 23.25616956148705938, 10.00000000000000000 ) ) ;
#85244=DIRECTION ( 'NONE',  ( 0.000000000000000000, -0.000000000000000000, -1.000000000000000000 ) ) ;
#85248=ADVANCED_FACE ( 'NONE', ( #82734 ), #13305, .T. ) ;
#85249=CARTESIAN_POINT ( 'NONE',  ( 47.39496755818311158, 108.2889530649357681, -10.00000000000000000 ) ) ;
#85259=EDGE_CURVE ( 'NONE', #66385, #1218, #43162, .T. ) ;
#85271=CARTESIAN_POINT ( 'NONE',  ( 20.94669640352213236, 37.57748520232516398, 10.00000000000000000 ) ) ;
#85275=CIRCLE ( 'NONE', #93366, 70.00000000000001421 ) ;
#85276=AXIS2_PLACEMENT_3D ( 'NONE', #54244, #85217, #15762 ) ;
#85283=FACE_OUTER_BOUND ( 'NONE', #60540, .T. ) ;
#85288=CIRCLE ( 'NONE', #23770, 70.00000000000001421 ) ;
#85289=LINE ( 'NONE', #77140, #77424 ) ;
#85291=EDGE_CURVE ( 'NONE', #7311, #60486, #77806, .T. ) ;
#85297=AXIS2_PLACEMENT_3D ( 'NONE', #13703, #82155, #89273 ) ;
#85298=CARTESIAN_POINT ( 'NONE',  ( -29.62033169268383404, 35.98430678844710684, 59.99999999999999289 ) ) ;
#85299=CARTESIAN_POINT ( 'NONE',  ( -19.65312891409030271, 93.06504152958497400, 203.6502102582797420 ) ) ;
#85300=DIRECTION ( 'NONE',  ( -0.3766285016932073293, 0.9263643838751195458, 0.000000000000000000 ) ) ;
#85307=ORIENTED_EDGE ( 'NONE', *, *, #36985, .T. ) ;
#85319=VERTEX_POINT ( 'NONE', #46663 ) ;
#85328=EDGE_CURVE ( 'NONE', #95622, #36742, #22866, .T. ) ;
#85330=LINE ( 'NONE', #22975, #1298 ) ;
#85332=EDGE_CURVE ( 'NONE', #17413, #77961, #82, .T. ) ;
#85339=EDGE_LOOP ( 'NONE', ( #41789, #78738, #4474, #30956 ) ) ;
#85343=CARTESIAN_POINT ( 'NONE',  ( -27.77457187288641904, 24.79904599702367562, -10.00000000000000000 ) ) ;
#85348=ORIENTED_EDGE ( 'NONE', *, *, #3505, .T. ) ;
#85353=ORIENTED_EDGE ( 'NONE', *, *, #58813, .F. ) ;
#85360=ORIENTED_EDGE ( 'NONE', *, *, #97792, .F. ) ;
#85378=ORIENTED_EDGE ( 'NONE', *, *, #93329, .T. ) ;
#85379=AXIS2_PLACEMENT_3D ( 'NONE', #54052, #93610, #24178 ) ;
#85388=AXIS2_PLACEMENT_3D ( 'NONE', #89694, #21248, #44013 ) ;
#85401=ORIENTED_EDGE ( 'NONE', *, *, #29935, .F. ) ;
#85411=CIRCLE ( 'NONE', #41681, 0.1418229129680828593 ) ;
#85415=LINE ( 'NONE', #32667, #43641 ) ;
#85416=VECTOR ( 'NONE', #94587, 1000.000000000000000 ) ;
#85426=LINE ( 'NONE', #8875, #92830 ) ;
#85429=LINE ( 'NONE', #8878, #31805 ) ;
#85432=VECTOR ( 'NONE', #91139, 1000.000000000000000 ) ;
#85434=PLANE ( 'NONE',  #19090 ) ;
#85438=CYLINDRICAL_SURFACE ( 'NONE', #7962, 70.00000000000002842 ) ;
#85439=AXIS2_PLACEMENT_3D ( 'NONE', #100267, #1466, #3472 ) ;
#85440=CARTESIAN_POINT ( 'NONE',  ( 39.25774830830064843, 55.25619937740605536, 10.00000000000000000 ) ) ;
#85445=FACE_OUTER_BOUND ( 'NONE', #82345, .T. ) ;
#85451=DIRECTION ( 'NONE',  ( 1.000000000000000000, 0.000000000000000000, 0.000000000000000000 ) ) ;
#85454=ORIENTED_EDGE ( 'NONE', *, *, #2735, .F. ) ;
#85461=VECTOR ( 'NONE', #76889, 1000.000000000000114 ) ;
#85470=ORIENTED_EDGE ( 'NONE', *, *, #45017, .F. ) ;
#85474=DIRECTION ( 'NONE',  ( 0.000000000000000000, -0.000000000000000000, -1.000000000000000000 ) ) ;
#85475=CARTESIAN_POINT ( 'NONE',  ( -52.58585057098314053, 88.59772970696691630, -10.00000000000000000 ) ) ;
#85478=ORIENTED_EDGE ( 'NONE', *, *, #98104, .F. ) ;
#85486=CARTESIAN_POINT ( 'NONE',  ( 46.43574122514301195, 74.10519008736565638, 10.00000000000000000 ) ) ;
#85488=FACE_OUTER_BOUND ( 'NONE', #64495, .T. ) ;
#85490=VECTOR ( 'NONE', #95429, 1000.000000000000114 ) ;
#85498=VECTOR ( 'NONE', #66168, 1000.000000000000227 ) ;
#85501=ORIENTED_EDGE ( 'NONE', *, *, #93047, .T. ) ;
#85503=AXIS2_PLACEMENT_3D ( 'NONE', #80710, #14125, #83561 ) ;
#85517=VERTEX_POINT ( 'NONE', #25367 ) ;
#85519=VECTOR ( 'NONE', #72161, 1000.000000000000000 ) ;
#85524=DIRECTION ( 'NONE',  ( -0.9999990636452668058, -0.001368469433204066998, 0.000000000000000000 ) ) ;
#85528=EDGE_LOOP ( 'NONE', ( #100106, #22013, #75203, #84356 ) ) ;
#85531=CARTESIAN_POINT ( 'NONE',  ( 47.83996289752659692, 111.6306699247848968, 10.00000000000000000 ) ) ;
#85537=CARTESIAN_POINT ( 'NONE',  ( 44.44844410339183582, 68.22168590943847732, 10.00000000000000000 ) ) ;
#85540=VECTOR ( 'NONE', #44905, 1000.000000000000227 ) ;
#85545=CARTESIAN_POINT ( 'NONE',  ( -50.41871976035449165, 31.58591985673634639, -10.00000000000000000 ) ) ;
#85548=AXIS2_PLACEMENT_3D ( 'NONE', #88790, #19359, #50219 ) ;
#85549=CARTESIAN_POINT ( 'NONE',  ( 33.47037235539275457, 49.41749479597460493, 10.00000000000000000 ) ) ;
#85554=CARTESIAN_POINT ( 'NONE',  ( -17.81126293257622706, 23.08927765589692527, 10.00000000000000000 ) ) ;
#85558=DIRECTION ( 'NONE',  ( 0.000000000000000000, 0.000000000000000000, 1.000000000000000000 ) ) ;
#85569=CIRCLE ( 'NONE', #48357, 49.99999999999999289 ) ;
#85578=VECTOR ( 'NONE', #12548, 1000.000000000000114 ) ;
#85582=EDGE_CURVE ( 'NONE', #21527, #9589, #33476, .T. ) ;
#85583=VECTOR ( 'NONE', #61956, 1000.000000000000000 ) ;
#85589=DIRECTION ( 'NONE',  ( 0.2398044646550112069, 0.9708212084269294273, 0.000000000000000000 ) ) ;
#85591=ORIENTED_EDGE ( 'NONE', *, *, #51700, .T. ) ;
#85599=CARTESIAN_POINT ( 'NONE',  ( -27.12601731895737700, 23.20384585402105770, 10.00000000000000000 ) ) ;
#85602=VECTOR ( 'NONE', #99959, 1000.000000000000000 ) ;
#85603=ORIENTED_EDGE ( 'NONE', *, *, #56178, .F. ) ;
#85610=ORIENTED_EDGE ( 'NONE', *, *, #76368, .F. ) ;
#85638=VECTOR ( 'NONE', #57553, 1000.000000000000000 ) ;
#85639=ORIENTED_EDGE ( 'NONE', *, *, #46259, .F. ) ;
#85642=VECTOR ( 'NONE', #81810, 1000.000000000000000 ) ;
#85644=AXIS2_PLACEMENT_3D ( 'NONE', #88095, #57113, #72861 ) ;
#85646=EDGE_CURVE ( 'NONE', #14328, #37072, #78590, .T. ) ;
#85648=DIRECTION ( 'NONE',  ( 0.000000000000000000, -0.000000000000000000, 1.000000000000000000 ) ) ;
#85650=VECTOR ( 'NONE', #96727, 1000.000000000000000 ) ;
#85654=LINE ( 'NONE', #37973, #35143 ) ;
#85661=LINE ( 'NONE', #93746, #47761 ) ;
#85662=VECTOR ( 'NONE', #65271, 1000.000000000000341 ) ;
#85678=EDGE_CURVE ( 'NONE', #35956, #27521, #21271, .T. ) ;
#85681=CARTESIAN_POINT ( 'NONE',  ( -45.75347490765856406, 28.11296735934751823, 177.5919119679930134 ) ) ;
#85698=EDGE_CURVE ( 'NONE', #65030, #70217, #40604, .T. ) ;
#85710=AXIS2_PLACEMENT_3D ( 'NONE', #913, #28951, #97862 ) ;
#85720=EDGE_LOOP ( 'NONE', ( #40717, #65149, #34467, #40736 ) ) ;
#85729=ADVANCED_FACE ( 'NONE', ( #75873 ), #90601, .F. ) ;
#85750=LINE ( 'NONE', #23369, #880 ) ;
#85751=EDGE_LOOP ( 'NONE', ( #4987, #15760, #9963, #24774 ) ) ;
#85754=DIRECTION ( 'NONE',  ( -0.8393827800519415572, -0.5435407515102007592, 0.000000000000000000 ) ) ;
#85757=DIRECTION ( 'NONE',  ( 0.6833540297821637521, -0.7300871660154543141, 0.000000000000000000 ) ) ;
#85759=CARTESIAN_POINT ( 'NONE',  ( 43.16562282991920085, 123.9487658730721904, 177.5919119679930134 ) ) ;
#85761=DIRECTION ( 'NONE',  ( -0.000000000000000000, -0.000000000000000000, -1.000000000000000000 ) ) ;
#85766=DIRECTION ( 'NONE',  ( -0.1239754375649670948, -0.9922852870422774751, 0.000000000000000000 ) ) ;
#85777=DIRECTION ( 'NONE',  ( 0.2803049773603250028, -0.9599109957006575211, 0.000000000000000000 ) ) ;
#85789=ORIENTED_EDGE ( 'NONE', *, *, #47834, .F. ) ;
#85807=DIRECTION ( 'NONE',  ( 0.3956464567955564338, -0.9184028970038813355, 0.000000000000000000 ) ) ;
#85808=EDGE_CURVE ( 'NONE', #8735, #70726, #83482, .T. ) ;
#85810=DIRECTION ( 'NONE',  ( -0.000000000000000000, 0.000000000000000000, -1.000000000000000000 ) ) ;
#85817=ORIENTED_EDGE ( 'NONE', *, *, #93715, .F. ) ;
#85822=DIRECTION ( 'NONE',  ( -0.4270171210482543445, 0.9042435392811277728, 0.000000000000000000 ) ) ;
#85823=CARTESIAN_POINT ( 'NONE',  ( 19.31801425620939483, 115.5650415295850451, -20.00000000000000355 ) ) ;
#85847=ORIENTED_EDGE ( 'NONE', *, *, #85046, .T. ) ;
#85850=FACE_OUTER_BOUND ( 'NONE', #18513, .T. ) ;
#85853=EDGE_CURVE ( 'NONE', #12944, #38056, #95960, .T. ) ;
#85857=LINE ( 'NONE', #61961, #70872 ) ;
#85868=ORIENTED_EDGE ( 'NONE', *, *, #23855, .T. ) ;
#85869=AXIS2_PLACEMENT_3D ( 'NONE', #94065, #77330, #100148 ) ;
#85871=PLANE ( 'NONE',  #94507 ) ;
#85874=VERTEX_POINT ( 'NONE', #92577 ) ;
#85881=ORIENTED_EDGE ( 'NONE', *, *, #33054, .F. ) ;
#85883=ORIENTED_EDGE ( 'NONE', *, *, #49379, .T. ) ;
#85897=DIRECTION ( 'NONE',  ( -0.3374500364938435304, -0.9413434404457831084, 0.000000000000000000 ) ) ;
#85902=LINE ( 'NONE', #39205, #18902 ) ;
#85904=LINE ( 'NONE', #24529, #21440 ) ;
#85910=PLANE ( 'NONE',  #51164 ) ;
#85911=DIRECTION ( 'NONE',  ( -0.7957378174433814566, 0.6056412518070772855, 0.000000000000000000 ) ) ;
#85914=EDGE_CURVE ( 'NONE', #84849, #28495, #56896, .T. ) ;
#85916=CARTESIAN_POINT ( 'NONE',  ( -4.653128914090325807, 78.77562236714182120, 52.49999999999999289 ) ) ;
#85923=VERTEX_POINT ( 'NONE', #63507 ) ;
#85924=LINE ( 'NONE', #70649, #59760 ) ;
#85926=EDGE_CURVE ( 'NONE', #67254, #47702, #98921, .T. ) ;
#85950=ORIENTED_EDGE ( 'NONE', *, *, #13247, .F. ) ;
#85962=CARTESIAN_POINT ( 'NONE',  ( 48.98007068238332096, 88.97864505566217019, -10.00000000000000000 ) ) ;
#85968=ORIENTED_EDGE ( 'NONE', *, *, #48834, .T. ) ;
#85972=EDGE_CURVE ( 'NONE', #75236, #37985, #38064, .T. ) ;
#85984=CARTESIAN_POINT ( 'NONE',  ( 49.07419501245632887, 91.40403951869188859, -10.00000000000000000 ) ) ;
#85987=DIRECTION ( 'NONE',  ( -0.2805612043866616001, -0.9598361373656993933, 0.000000000000000000 ) ) ;
#85995=ORIENTED_EDGE ( 'NONE', *, *, #17553, .F. ) ;
#85997=VERTEX_POINT ( 'NONE', #92818 ) ;
#86003=VERTEX_POINT ( 'NONE', #87270 ) ;
#86011=DIRECTION ( 'NONE',  ( 0.6116140086401538056, -0.7911563084720502070, 0.000000000000000000 ) ) ;
#86028=LINE ( 'NONE', #32255, #33549 ) ;
#86031=DIRECTION ( 'NONE',  ( -0.1654779384134575371, 0.9862134920484671996, 0.000000000000000000 ) ) ;
#86041=DIRECTION ( 'NONE',  ( -0.2270762630343691746, 0.9738769792773346312, 0.000000000000000000 ) ) ;
#86045=CARTESIAN_POINT ( 'NONE',  ( 20.94669640352213236, 37.57748520232516398, 10.00000000000000000 ) ) ;
#86050=EDGE_CURVE ( 'NONE', #23431, #72257, #71509, .T. ) ;
#86060=CARTESIAN_POINT ( 'NONE',  ( -19.65312891409030271, 93.06504152958497400, 10.00000000000000888 ) ) ;
#86061=ADVANCED_FACE ( 'NONE', ( #58276, #97312, #27879, #13199, #19802, #58761, #57274, #42563, #50183, #4584, #88250, #20292, #73012, #18798, #49680, #80636, #82132, #50669, #81621, #11213, #96325, #12194, #26895, #57773, #43053, #12704, #43574, #73999, #29385, #98298, #84613, #91709, #14184, #15152, #61258, #99785, #67372, #45559, #22271, #45069, #37951, #22778, #37457, #53175, #14678, #53655, #76008, #84129, #28887, #21772, #52662 ), #68860, .F. ) ;
#86063=CARTESIAN_POINT ( 'NONE',  ( -50.07135831343601495, 43.74682248199032841, 59.99999999999999289 ) ) ;
#86065=DIRECTION ( 'NONE',  ( -1.000000000000000000, 0.000000000000000000, -0.000000000000000000 ) ) ;
#86077=DIRECTION ( 'NONE',  ( -0.7135562106085605594, 0.7005979833698863235, 0.000000000000000000 ) ) ;
#86098=ORIENTED_EDGE ( 'NONE', *, *, #78821, .F. ) ;
#86113=CARTESIAN_POINT ( 'NONE',  ( -19.65312891409030271, 93.06504152958497400, 177.5919119679930134 ) ) ;
#86115=ORIENTED_EDGE ( 'NONE', *, *, #22591, .F. ) ;
#86119=DIRECTION ( 'NONE',  ( -0.8560416229147732592, -0.5169068966820244970, 0.000000000000000000 ) ) ;
#86140=FACE_OUTER_BOUND ( 'NONE', #75588, .T. ) ;
#86147=ORIENTED_EDGE ( 'NONE', *, *, #63926, .F. ) ;
#86151=VERTEX_POINT ( 'NONE', #52165 ) ;
#86185=ORIENTED_EDGE ( 'NONE', *, *, #80627, .F. ) ;
#86191=VECTOR ( 'NONE', #67851, 1000.000000000000114 ) ;
#86208=AXIS2_PLACEMENT_3D ( 'NONE', #95501, #728, #48342 ) ;
#86222=LINE ( 'NONE', #76, #11828 ) ;
#86225=LINE ( 'NONE', #23856, #37152 ) ;
#86226=EDGE_CURVE ( 'NONE', #84464, #48146, #21610, .T. ) ;
#86232=DIRECTION ( 'NONE',  ( -0.000000000000000000, -0.000000000000000000, -1.000000000000000000 ) ) ;
#86242=ORIENTED_EDGE ( 'NONE', *, *, #4120, .F. ) ;
#86254=FACE_OUTER_BOUND ( 'NONE', #75985, .T. ) ;
#86274=EDGE_CURVE ( 'NONE', #95220, #1951, #61650, .T. ) ;
#86279=ORIENTED_EDGE ( 'NONE', *, *, #52940, .F. ) ;
#86290=DIRECTION ( 'NONE',  ( 0.7059494278973770243, -0.7082622432767159415, 0.000000000000000000 ) ) ;
#86295=CARTESIAN_POINT ( 'NONE',  ( -32.04500338604974985, 25.44370296803430520, 10.00000000000000000 ) ) ;
#86306=CARTESIAN_POINT ( 'NONE',  ( -51.35363524361505227, 103.0449678370604687, -10.00000000000000000 ) ) ;
#86331=ORIENTED_EDGE ( 'NONE', *, *, #29049, .T. ) ;
#86346=LINE ( 'NONE', #61478, #19118 ) ;
#86351=ORIENTED_EDGE ( 'NONE', *, *, #54968, .T. ) ;
#86353=CIRCLE ( 'NONE', #65253, 0.1418229129680897982 ) ;
#86355=EDGE_LOOP ( 'NONE', ( #19333, #99536, #86509, #48338 ) ) ;
#86357=DIRECTION ( 'NONE',  ( 0.000000000000000000, 0.000000000000000000, 1.000000000000000000 ) ) ;
#86382=LINE ( 'NONE', #78736, #9531 ) ;
#86384=LINE ( 'NONE', #226, #93298 ) ;
#86389=ORIENTED_EDGE ( 'NONE', *, *, #37389, .F. ) ;
#86394=CARTESIAN_POINT ( 'NONE',  ( 27.88397166348279654, 69.57562948509108480, 59.99999999999999289 ) ) ;
#86407=FACE_BOUND ( 'NONE', #34470, .T. ) ;
#86411=VECTOR ( 'NONE', #59729, 1000.000000000000114 ) ;
#86414=ORIENTED_EDGE ( 'NONE', *, *, #23905, .T. ) ;
#86417=LINE ( 'NONE', #68914, #12874 ) ;
#86420=CARTESIAN_POINT ( 'NONE',  ( -3.216670782107629911, 25.02209300385174373, -10.00000000000000000 ) ) ;
#86421=VECTOR ( 'NONE', #87635, 1000.000000000000000 ) ;
#86422=DIRECTION ( 'NONE',  ( -0.2126238682951524517, 0.9771341211068240717, 0.000000000000000000 ) ) ;
#86423=CARTESIAN_POINT ( 'NONE',  ( 48.48788556946983874, 102.1758113618167982, -10.00000000000000000 ) ) ;
#86443=ORIENTED_EDGE ( 'NONE', *, *, #9515, .T. ) ;
#86451=DIRECTION ( 'NONE',  ( -0.9985601716053730259, 0.05364311403570636710, 0.000000000000000000 ) ) ;
#86461=ORIENTED_EDGE ( 'NONE', *, *, #78353, .T. ) ;
#86463=CARTESIAN_POINT ( 'NONE',  ( 30.79296800917359889, 109.3972131079642338, 59.99999999999999289 ) ) ;
#86465=ORIENTED_EDGE ( 'NONE', *, *, #60812, .T. ) ;
#86471=EDGE_LOOP ( 'NONE', ( #81586, #37964, #52654, #53883 ) ) ;
#86479=ORIENTED_EDGE ( 'NONE', *, *, #100231, .T. ) ;
#86480=EDGE_CURVE ( 'NONE', #70676, #23520, #22965, .T. ) ;
#86488=EDGE_CURVE ( 'NONE', #11929, #62608, #45511, .T. ) ;
#86494=ORIENTED_EDGE ( 'NONE', *, *, #34864, .F. ) ;
#86496=CARTESIAN_POINT ( 'NONE',  ( 40.34888600819125060, 126.6204015641749834, -10.00000000000000000 ) ) ;
#86505=VECTOR ( 'NONE', #59505, 1000.000000000000114 ) ;
#86509=ORIENTED_EDGE ( 'NONE', *, *, #94019, .T. ) ;
#86520=CARTESIAN_POINT ( 'NONE',  ( 43.63646518856938172, 66.22046553916848666, -10.00000000000000000 ) ) ;
#86523=ADVANCED_FACE ( 'NONE', ( #99498 ), #30078, .F. ) ;
#86566=CARTESIAN_POINT ( 'NONE',  ( -29.48056340892364346, 35.96025339996432280, 59.99999999999999289 ) ) ;
#86577=CARTESIAN_POINT ( 'NONE',  ( 48.29091023345864642, 82.53782597618220507, -10.00000000000000000 ) ) ;
#86580=PLANE ( 'NONE',  #23151 ) ;
#86586=DIRECTION ( 'NONE',  ( -1.000000000000000000, 0.000000000000000000, 0.000000000000000000 ) ) ;
#86603=AXIS2_PLACEMENT_3D ( 'NONE', #99629, #8903, #53984 ) ;
#86608=CARTESIAN_POINT ( 'NONE',  ( -62.95439910331221256, 68.06504152958493137, 60.00000000000000000 ) ) ;
#86609=EDGE_CURVE ( 'NONE', #30332, #39213, #94413, .T. ) ;
#86622=CARTESIAN_POINT ( 'NONE',  ( 39.77289032284285497, 58.49985355908045648, -10.00000000000000000 ) ) ;
#86627=ORIENTED_EDGE ( 'NONE', *, *, #89267, .T. ) ;
#86638=AXIS2_PLACEMENT_3D ( 'NONE', #72873, #81975, #58132 ) ;
#86639=ORIENTED_EDGE ( 'NONE', *, *, #25039, .T. ) ;
#86645=AXIS2_PLACEMENT_3D ( 'NONE', #69188, #61081, #68685 ) ;
#86648=CARTESIAN_POINT ( 'NONE',  ( 47.92671612011950799, 80.40884667711614497, -10.00000000000000000 ) ) ;
#86655=DIRECTION ( 'NONE',  ( 1.000000000000000000, 0.000000000000000000, 0.000000000000000000 ) ) ;
#86667=EDGE_CURVE ( 'NONE', #82593, #27025, #23967, .T. ) ;
#86674=CARTESIAN_POINT ( 'NONE',  ( -34.42581292930597670, 25.91608375674935161, -10.00000000000000000 ) ) ;
#86677=DIRECTION ( 'NONE',  ( 0.000000000000000000, 0.000000000000000000, 1.000000000000000000 ) ) ;
#86684=DIRECTION ( 'NONE',  ( -0.4055404667435467125, 0.9140770918436946779, 0.000000000000000000 ) ) ;
#86689=DIRECTION ( 'NONE',  ( -0.7715546603183375263, -0.6361630342459821952, 0.000000000000000000 ) ) ;
#86707=CARTESIAN_POINT ( 'NONE',  ( -19.65312891409030271, 93.06504152958497400, 177.5919119679930134 ) ) ;
#86708=LINE ( 'NONE', #17243, #46064 ) ;
#86721=CARTESIAN_POINT ( 'NONE',  ( -33.75225536883274913, 24.49963747467413810, -10.00000000000000000 ) ) ;
#86722=DIRECTION ( 'NONE',  ( -0.9708212084269268738, 0.2398044646550215042, 0.000000000000000000 ) ) ;
#86739=EDGE_CURVE ( 'NONE', #38705, #57548, #74637, .T. ) ;
#86754=VECTOR ( 'NONE', #34521, 1000.000000000000114 ) ;
#86769=CARTESIAN_POINT ( 'NONE',  ( 46.80869107419874098, 110.6443039040113092, -10.00000000000000000 ) ) ;
#86771=DIRECTION ( 'NONE',  ( 0.000000000000000000, 0.000000000000000000, 1.000000000000000000 ) ) ;
#86789=EDGE_CURVE ( 'NONE', #26239, #99548, #16375, .T. ) ;
#86793=EDGE_CURVE ( 'NONE', #2857, #56966, #56366, .T. ) ;
#86800=ADVANCED_FACE ( 'NONE', ( #41157 ), #33585, .F. ) ;
#86844=AXIS2_PLACEMENT_3D ( 'NONE', #78917, #18097, #41375 ) ;
#86847=EDGE_CURVE ( 'NONE', #7311, #28252, #72605, .T. ) ;
#86856=CARTESIAN_POINT ( 'NONE',  ( 13.67211979723576931, 32.92651376809308772, -10.00000000000000000 ) ) ;
#86862=VERTEX_POINT ( 'NONE', #96412 ) ;
#86864=EDGE_CURVE ( 'NONE', #98279, #78709, #90856, .T. ) ;
#86872=ORIENTED_EDGE ( 'NONE', *, *, #9504, .F. ) ;
#86875=ORIENTED_EDGE ( 'NONE', *, *, #87671, .F. ) ;
#86882=CARTESIAN_POINT ( 'NONE',  ( 44.98086946945896614, 119.9434018396067785, 10.00000000000000000 ) ) ;
#86887=ORIENTED_EDGE ( 'NONE', *, *, #52020, .T. ) ;
#86888=DIRECTION ( 'NONE',  ( -0.4535245244745221282, 0.8912437970051507730, 0.000000000000000000 ) ) ;
#86895=VECTOR ( 'NONE', #80505, 1000.000000000000000 ) ;
#86899=CARTESIAN_POINT ( 'NONE',  ( -19.65312891409030271, 93.06504152958497400, 60.00000000000000000 ) ) ;
#86903=ORIENTED_EDGE ( 'NONE', *, *, #26582, .T. ) ;
#86907=LINE ( 'NONE', #11379, #66136 ) ;
#86915=EDGE_CURVE ( 'NONE', #44311, #74402, #16386, .T. ) ;
#86917=AXIS2_PLACEMENT_3D ( 'NONE', #67666, #60542, #92491 ) ;
#86920=PRODUCT_DEFINITION_CONTEXT ( 'detailed design', #5503, 'design' ) ;
#86924=ADVANCED_FACE ( 'NONE', ( #49283 ), #57363, .F. ) ;
#86947=ADVANCED_FACE ( 'NONE', ( #21366 ), #5659, .F. ) ;
#86953=PLANE ( 'NONE',  #32243 ) ;
#86959=VECTOR ( 'NONE', #45376, 1000.000000000000114 ) ;
#86966=AXIS2_PLACEMENT_3D ( 'NONE', #90435, #29578, #12909 ) ;
#86967=LINE ( 'NONE', #41283, #527 ) ;
#86968=EDGE_CURVE ( 'NONE', #16667, #15864, #29459, .T. ) ;
#86976=AXIS2_PLACEMENT_3D ( 'NONE', #34258, #12470, #82413 ) ;
#86977=ORIENTED_EDGE ( 'NONE', *, *, #77355, .T. ) ;
#86985=ORIENTED_EDGE ( 'NONE', *, *, #30962, .F. ) ;
#86989=CARTESIAN_POINT ( 'NONE',  ( 17.00529913897481293, 33.43149683636510616, 177.5919119679930134 ) ) ;
#86991=VECTOR ( 'NONE', #18826, 1000.000000000000000 ) ;
#86993=ADVANCED_FACE ( 'NONE', ( #31437 ), #8652, .F. ) ;
#86998=ORIENTED_EDGE ( 'NONE', *, *, #89456, .F. ) ;
#87005=AXIS2_PLACEMENT_3D ( 'NONE', #39487, #41504, #80059 ) ;
#87008=CARTESIAN_POINT ( 'NONE',  ( 42.33744422746376301, 122.7866300363639169, -10.00000000000000000 ) ) ;
#87019=ORIENTED_EDGE ( 'NONE', *, *, #52947, .T. ) ;
#87023=DIRECTION ( 'NONE',  ( -0.9303772761487891785, -0.3666034970181814012, 0.000000000000000000 ) ) ;
#87032=ORIENTED_EDGE ( 'NONE', *, *, #92565, .T. ) ;
#87033=FACE_OUTER_BOUND ( 'NONE', #58874, .T. ) ;
#87036=DIRECTION ( 'NONE',  ( 0.000000000000000000, 0.000000000000000000, 1.000000000000000000 ) ) ;
#87042=AXIS2_PLACEMENT_3D ( 'NONE', #14025, #21149, #82968 ) ;
#87045=DIRECTION ( 'NONE',  ( -0.000000000000000000, -0.000000000000000000, -1.000000000000000000 ) ) ;
#87059=VECTOR ( 'NONE', #92569, 1000.000000000000000 ) ;
#87060=DIRECTION ( 'NONE',  ( 0.4242989612870596283, -0.9055221650797523614, 0.000000000000000000 ) ) ;
#87064=CARTESIAN_POINT ( 'NONE',  ( -58.62427208439002158, 70.56504152958493137, 20.00000000000000355 ) ) ;
#87073=DIRECTION ( 'NONE',  ( 1.000000000000000000, 0.000000000000000000, 0.000000000000000000 ) ) ;
#87087=ORIENTED_EDGE ( 'NONE', *, *, #17117, .T. ) ;
#87099=EDGE_CURVE ( 'NONE', #96593, #79260, #47637, .T. ) ;
#87101=VERTEX_POINT ( 'NONE', #41031 ) ;
#87110=EDGE_CURVE ( 'NONE', #41680, #18235, #8366, .T. ) ;
#87116=VECTOR ( 'NONE', #65426, 1000.000000000000000 ) ;
#87119=EDGE_CURVE ( 'NONE', #6688, #97892, #25347, .T. ) ;
#87123=EDGE_CURVE ( 'NONE', #76464, #72231, #16749, .T. ) ;
#87133=CARTESIAN_POINT ( 'NONE',  ( 34.81516168915606357, 51.10768172523390973, 10.00000000000000000 ) ) ;
#87139=AXIS2_PLACEMENT_3D ( 'NONE', #99646, #53521, #61112 ) ;
#87142=ORIENTED_EDGE ( 'NONE', *, *, #44572, .F. ) ;
#87155=EDGE_LOOP ( 'NONE', ( #96826, #59219, #98939, #66340 ) ) ;
#87166=ORIENTED_EDGE ( 'NONE', *, *, #1377, .F. ) ;
#87171=DIRECTION ( 'NONE',  ( 0.9598361373656965068, -0.2805612043866717031, 0.000000000000000000 ) ) ;
#87173=DIRECTION ( 'NONE',  ( -1.000000000000000000, 0.000000000000000000, 0.000000000000000000 ) ) ;
#87175=CARTESIAN_POINT ( 'NONE',  ( -19.65312891409030271, 93.06504152958497400, 177.5919119679930134 ) ) ;
#87178=AXIS2_PLACEMENT_3D ( 'NONE', #79280, #65033, #48335 ) ;
#87183=ORIENTED_EDGE ( 'NONE', *, *, #70159, .F. ) ;
#87185=CIRCLE ( 'NONE', #64477, 70.00000000000001421 ) ;
#87191=EDGE_CURVE ( 'NONE', #79669, #56390, #28727, .T. ) ;
#87200=VECTOR ( 'NONE', #63715, 1000.000000000000114 ) ;
#87203=VERTEX_POINT ( 'NONE', #43911 ) ;
#87205=FACE_OUTER_BOUND ( 'NONE', #14562, .T. ) ;
#87208=LINE ( 'NONE', #41004, #60380 ) ;
#87217=CARTESIAN_POINT ( 'NONE',  ( -58.62427208439001447, 70.56504152958493137, -20.00000000000000355 ) ) ;
#87221=CARTESIAN_POINT ( 'NONE',  ( -19.65312891409030271, 93.06504152958497400, -10.00000000000000888 ) ) ;
#87223=CARTESIAN_POINT ( 'NONE',  ( 50.51697681462041345, 96.61285555410614734, -10.00000000000000000 ) ) ;
#87225=CARTESIAN_POINT ( 'NONE',  ( -6.979067178619878575, 83.87849322502869143, 13.57452325917756220 ) ) ;
#87228=CARTESIAN_POINT ( 'NONE',  ( 24.17817230090144065, 55.16553699959921175, 59.99999999999999289 ) ) ;
#87231=FACE_OUTER_BOUND ( 'NONE', #50315, .T. ) ;
#87233=DIRECTION ( 'NONE',  ( 0.000000000000000000, 0.000000000000000000, 1.000000000000000000 ) ) ;
#87249=ORIENTED_EDGE ( 'NONE', *, *, #85972, .F. ) ;
#87255=AXIS2_PLACEMENT_3D ( 'NONE', #18079, #95116, #17057 ) ;
#87256=FACE_OUTER_BOUND ( 'NONE', #62135, .T. ) ;
#87261=VECTOR ( 'NONE', #192, 999.9999999999998863 ) ;
#87262=VECTOR ( 'NONE', #81503, 1000.000000000000000 ) ;
#87265=ORIENTED_EDGE ( 'NONE', *, *, #5644, .F. ) ;
#87266=VECTOR ( 'NONE', #98529, 1000.000000000000000 ) ;
#87268=ORIENTED_EDGE ( 'NONE', *, *, #5342, .F. ) ;
#87270=CARTESIAN_POINT ( 'NONE',  ( 11.23059542939759936, 30.24628978557580794, 10.00000000000000000 ) ) ;
#87276=CARTESIAN_POINT ( 'NONE',  ( 35.43817338645655468, 49.87999306568065805, 10.00000000000000000 ) ) ;
#87278=ORIENTED_EDGE ( 'NONE', *, *, #66147, .F. ) ;
#87279=VECTOR ( 'NONE', #12289, 1000.000000000000114 ) ;
#87283=ORIENTED_EDGE ( 'NONE', *, *, #287, .F. ) ;
#87290=AXIS2_PLACEMENT_3D ( 'NONE', #21328, #13723, #37015 ) ;
#87299=DIRECTION ( 'NONE',  ( 0.000000000000000000, 0.000000000000000000, 1.000000000000000000 ) ) ;
#87312=LINE ( 'NONE', #55308, #4605 ) ;
#87321=LINE ( 'NONE', #17853, #48333 ) ;
#87322=LINE ( 'NONE', #17854, #10729 ) ;
#87330=VECTOR ( 'NONE', #49503, 1000.000000000000114 ) ;
#87345=CARTESIAN_POINT ( 'NONE',  ( -62.95439910331221256, 68.06504152958493137, -40.00000000000000000 ) ) ;
#87348=AXIS2_PLACEMENT_3D ( 'NONE', #80422, #65660, #43354 ) ;
#87356=CARTESIAN_POINT ( 'NONE',  ( -19.65312891409030271, 93.06504152958497400, 177.5919119679930134 ) ) ;
#87362=ORIENTED_EDGE ( 'NONE', *, *, #43183, .T. ) ;
#87370=DIRECTION ( 'NONE',  ( -0.000000000000000000, -0.000000000000000000, -1.000000000000000000 ) ) ;
#87379=EDGE_LOOP ( 'NONE', ( #12596, #73771, #6800, #87249 ) ) ;
#87385=CARTESIAN_POINT ( 'NONE',  ( -66.34925969370661392, 42.61035540433362456, -10.00000000000000000 ) ) ;
#87412=VECTOR ( 'NONE', #81388, 1000.000000000000000 ) ;
#87413=DIRECTION ( 'NONE',  ( -0.9879428538673719062, -0.1548189829846212673, 0.000000000000000000 ) ) ;
#87426=PLANE ( 'NONE',  #47314 ) ;
#87428=VERTEX_POINT ( 'NONE', #56504 ) ;
#87431=CARTESIAN_POINT ( 'NONE',  ( 50.20806676147353187, 85.59215312471712878, 10.00000000000000000 ) ) ;
#87440=VECTOR ( 'NONE', #44777, 1000.000000000000114 ) ;
#87442=ORIENTED_EDGE ( 'NONE', *, *, #53591, .F. ) ;
#87455=EDGE_CURVE ( 'NONE', #40778, #37845, #1822, .T. ) ;
#87458=DIRECTION ( 'NONE',  ( -0.000000000000000000, -0.000000000000000000, -1.000000000000000000 ) ) ;
#87471=VECTOR ( 'NONE', #11042, 1000.000000000000000 ) ;
#87483=DIRECTION ( 'NONE',  ( 0.3103181967972123423, -0.9506327454577433445, 0.000000000000000000 ) ) ;
#87496=ORIENTED_EDGE ( 'NONE', *, *, #34639, .F. ) ;
#87499=CARTESIAN_POINT ( 'NONE',  ( -54.45295541630240166, 33.76759809053437777, -10.00000000000000000 ) ) ;
#87500=ORIENTED_EDGE ( 'NONE', *, *, #69873, .F. ) ;
#87505=PLANE ( 'NONE',  #46820 ) ;
#87523=DIRECTION ( 'NONE',  ( -0.9607486656258008573, -0.2774202615135435979, 0.000000000000000000 ) ) ;
#87525=EDGE_CURVE ( 'NONE', #1235, #62719, #48920, .T. ) ;
#87526=DIRECTION ( 'NONE',  ( -0.8903844177683373218, -0.4552093898365224267, 0.000000000000000000 ) ) ;
#87530=FACE_OUTER_BOUND ( 'NONE', #53444, .T. ) ;
#87535=DIRECTION ( 'NONE',  ( 0.5803476755362092510, 0.8143688203140632131, 0.000000000000000000 ) ) ;
#87539=DIRECTION ( 'NONE',  ( 0.000000000000000000, -0.000000000000000000, -1.000000000000000000 ) ) ;
#87541=DIRECTION ( 'NONE',  ( -0.7696402260561131525, -0.6384778167143280170, 0.000000000000000000 ) ) ;
#87543=EDGE_LOOP ( 'NONE', ( #24423, #9783, #25156, #83511 ) ) ;
#87547=CARTESIAN_POINT ( 'NONE',  ( 30.91722093456329645, 63.30801963086432949, 59.99999999999999289 ) ) ;
#87558=FACE_OUTER_BOUND ( 'NONE', #24608, .T. ) ;
#87562=AXIS2_PLACEMENT_3D ( 'NONE', #58550, #19092, #27681 ) ;
#87565=PLANE ( 'NONE',  #49863 ) ;
#87571=DIRECTION ( 'NONE',  ( -0.9909246428798921258, -0.1344185706417024839, 0.000000000000000000 ) ) ;
#87573=LINE ( 'NONE', #85549, #50556 ) ;
#87574=CARTESIAN_POINT ( 'NONE',  ( 19.39999966495784989, 36.48715600906564305, -10.00000000000000000 ) ) ;
#87577=FACE_OUTER_BOUND ( 'NONE', #71022, .T. ) ;
#87578=ADVANCED_FACE ( 'NONE', ( #46635 ), #85184, .F. ) ;
#87589=FACE_OUTER_BOUND ( 'NONE', #28136, .T. ) ;
#87592=CARTESIAN_POINT ( 'NONE',  ( -3.019589773780833930, 24.80263534580897300, -10.00000000000000000 ) ) ;
#87597=ORIENTED_EDGE ( 'NONE', *, *, #68711, .F. ) ;
#87602=LINE ( 'NONE', #42885, #44196 ) ;
#87604=EDGE_LOOP ( 'NONE', ( #55131, #41840, #41437, #42447 ) ) ;
#87610=EDGE_LOOP ( 'NONE', ( #88379, #84800, #38951, #13051 ) ) ;
#87612=EDGE_LOOP ( 'NONE', ( #105, #49574, #96803, #98913 ) ) ;
#87615=CARTESIAN_POINT ( 'NONE',  ( -11.40312891409031693, 78.77562236714182120, 52.49999999999999289 ) ) ;
#87617=DIRECTION ( 'NONE',  ( -0.000000000000000000, -0.000000000000000000, -1.000000000000000000 ) ) ;
#87618=VERTEX_POINT ( 'NONE', #39515 ) ;
#87621=DIRECTION ( 'NONE',  ( 0.1237105541964824001, -0.9923183454821336014, 0.000000000000000000 ) ) ;
#87628=DIRECTION ( 'NONE',  ( -0.000000000000000000, 0.000000000000000000, -1.000000000000000000 ) ) ;
#87629=CARTESIAN_POINT ( 'NONE',  ( -78.24550368024017644, 54.29179893118896416, 10.00000000000000000 ) ) ;
#87631=VECTOR ( 'NONE', #10285, 1000.000000000000000 ) ;
#87632=ORIENTED_EDGE ( 'NONE', *, *, #85117, .F. ) ;
#87635=DIRECTION ( 'NONE',  ( -0.6625377181876236365, -0.7490285521785781109, 0.000000000000000000 ) ) ;
#87641=EDGE_CURVE ( 'NONE', #50852, #81157, #6656, .T. ) ;
#87643=DIRECTION ( 'NONE',  ( -0.8660254037844379305, -0.5000000000000011102, -0.000000000000000000 ) ) ;
#87646=DIRECTION ( 'NONE',  ( -0.6139877827364832452, 0.7893155279419866721, 0.000000000000000000 ) ) ;
#87650=VERTEX_POINT ( 'NONE', #70440 ) ;
#87652=EDGE_CURVE ( 'NONE', #70323, #82431, #76080, .T. ) ;
#87660=ORIENTED_EDGE ( 'NONE', *, *, #97129, .T. ) ;
#87671=EDGE_CURVE ( 'NONE', #81514, #97599, #16742, .T. ) ;
#87673=DIRECTION ( 'NONE',  ( 0.000000000000000000, 0.000000000000000000, 1.000000000000000000 ) ) ;
#87675=LINE ( 'NONE', #18210, #44932 ) ;
#87676=ORIENTED_EDGE ( 'NONE', *, *, #49300, .T. ) ;
#87683=CARTESIAN_POINT ( 'NONE',  ( -33.66737166714137430, 24.21715323669988607, -10.00000000000000000 ) ) ;
#87688=ADVANCED_FACE ( 'NONE', ( #9668 ), #9148, .F. ) ;
#87700=DIRECTION ( 'NONE',  ( -0.000000000000000000, -0.000000000000000000, -1.000000000000000000 ) ) ;
#87701=ORIENTED_EDGE ( 'NONE', *, *, #72707, .T. ) ;
#87708=CARTESIAN_POINT ( 'NONE',  ( 48.87252615048947035, 107.3561085985703016, 10.00000000000000000 ) ) ;
#87721=DIRECTION ( 'NONE',  ( -0.5169068966820244970, 0.8560416229147732592, 0.000000000000000000 ) ) ;
#87722=EDGE_LOOP ( 'NONE', ( #73402, #30599, #48330, #65275 ) ) ;
#87723=CARTESIAN_POINT ( 'NONE',  ( -17.28329050831346692, 82.11986129481219621, 14.61049846789633300 ) ) ;
#87725=DIRECTION ( 'NONE',  ( -0.9414334852479518956, -0.3371987438498165734, 0.000000000000000000 ) ) ;
#87734=CARTESIAN_POINT ( 'NONE',  ( 44.08135397534552169, 118.8355609772188188, 10.00000000000000000 ) ) ;
#87739=ORIENTED_EDGE ( 'NONE', *, *, #3345, .T. ) ;
#87744=ORIENTED_EDGE ( 'NONE', *, *, #10851, .T. ) ;
#87750=CARTESIAN_POINT ( 'NONE',  ( -71.61465314115659453, 63.06504152958490295, 203.6502102582797420 ) ) ;
#87771=EDGE_CURVE ( 'NONE', #58503, #58533, #30210, .T. ) ;
#87777=ORIENTED_EDGE ( 'NONE', *, *, #91424, .T. ) ;
#87792=DIRECTION ( 'NONE',  ( -0.000000000000000000, -0.000000000000000000, -1.000000000000000000 ) ) ;
#87793=CARTESIAN_POINT ( 'NONE',  ( 40.34888600819125770, 126.6204015641749834, -10.00000000000000000 ) ) ;
#87796=ORIENTED_EDGE ( 'NONE', *, *, #80492, .T. ) ;
#87798=EDGE_CURVE ( 'NONE', #94453, #73260, #28212, .T. ) ;
#87807=AXIS2_PLACEMENT_3D ( 'NONE', #17255, #79102, #9686 ) ;
#87819=VERTEX_POINT ( 'NONE', #77311 ) ;
#87838=DIRECTION ( 'NONE',  ( 0.000000000000000000, 0.000000000000000000, 1.000000000000000000 ) ) ;
#87854=LINE ( 'NONE', #45880, #43702 ) ;
#87878=VERTEX_POINT ( 'NONE', #7920 ) ;
#87880=VECTOR ( 'NONE', #44523, 1000.000000000000227 ) ;
#87885=ORIENTED_EDGE ( 'NONE', *, *, #77903, .T. ) ;
#87890=EDGE_CURVE ( 'NONE', #53400, #18010, #96053, .T. ) ;
#87895=CARTESIAN_POINT ( 'NONE',  ( 48.92549481379852949, 97.87922363803308201, -10.00000000000000000 ) ) ;
#87897=VECTOR ( 'NONE', #40210, 1000.000000000000000 ) ;
#87899=DIRECTION ( 'NONE',  ( -1.000000000000000000, 0.000000000000000000, 0.000000000000000000 ) ) ;
#87904=CARTESIAN_POINT ( 'NONE',  ( -19.65312891409030271, 93.06504152958497400, 10.00000000000000888 ) ) ;
#87905=CARTESIAN_POINT ( 'NONE',  ( 16.73070718246250621, 56.29032694264133596, 59.99999999999999289 ) ) ;
#87907=VERTEX_POINT ( 'NONE', #11435 ) ;
#87928=ORIENTED_EDGE ( 'NONE', *, *, #34307, .T. ) ;
#87929=ORIENTED_EDGE ( 'NONE', *, *, #74715, .T. ) ;
#87958=CARTESIAN_POINT ( 'NONE',  ( -3.019589773780833930, 24.80263534580897300, 10.00000000000000000 ) ) ;
#87959=VECTOR ( 'NONE', #90944, 1000.000000000000114 ) ;
#87962=CARTESIAN_POINT ( 'NONE',  ( -52.31886624268647523, 30.86069821571189919, 10.00000000000000000 ) ) ;
#87966=FACE_OUTER_BOUND ( 'NONE', #5049, .T. ) ;
#87978=DIRECTION ( 'NONE',  ( 0.000000000000000000, 0.000000000000000000, 1.000000000000000000 ) ) ;
#87994=ORIENTED_EDGE ( 'NONE', *, *, #8879, .F. ) ;
#87997=ORIENTED_EDGE ( 'NONE', *, *, #12012, .T. ) ;
#88001=LINE ( 'NONE', #17022, #2362 ) ;
#88009=CARTESIAN_POINT ( 'NONE',  ( -11.40312891409031693, 78.77562236714182120, 59.97499999999998721 ) ) ;
#88010=EDGE_CURVE ( 'NONE', #28615, #94399, #67589, .T. ) ;
#88024=CARTESIAN_POINT ( 'NONE',  ( -19.65312891409030271, 93.06504152958497400, 10.00000000000000888 ) ) ;
#88032=VECTOR ( 'NONE', #93534, 1000.000000000000000 ) ;
#88035=VECTOR ( 'NONE', #13738, 1000.000000000000114 ) ;
#88038=CARTESIAN_POINT ( 'NONE',  ( -11.87431992379006296, 23.49859753039504895, 10.00000000000000000 ) ) ;
#88042=DIRECTION ( 'NONE',  ( 1.000000000000000000, 0.000000000000000000, 0.000000000000000000 ) ) ;
#88047=DIRECTION ( 'NONE',  ( 0.000000000000000000, 0.000000000000000000, 1.000000000000000000 ) ) ;
#88048=DIRECTION ( 'NONE',  ( -0.07193265315672570104, 0.9974094913373514615, 0.000000000000000000 ) ) ;
#88050=DIRECTION ( 'NONE',  ( -0.000000000000000000, -0.000000000000000000, -1.000000000000000000 ) ) ;
#88060=DIRECTION ( 'NONE',  ( 0.6833540297821638632, -0.7300871660154544251, 0.000000000000000000 ) ) ;
#88061=FACE_OUTER_BOUND ( 'NONE', #76146, .T. ) ;
#88072=EDGE_CURVE ( 'NONE', #90334, #38467, #97526, .T. ) ;
#88077=CARTESIAN_POINT ( 'NONE',  ( 41.19957572438558913, 58.46810036157969392, 10.00000000000000000 ) ) ;
#88078=DIRECTION ( 'NONE',  ( -0.6681572590663601430, 0.7440200784635646603, 0.000000000000000000 ) ) ;
#88079=LINE ( 'NONE', #32808, #41228 ) ;
#88089=CARTESIAN_POINT ( 'NONE',  ( -28.04097607764120781, 24.82386083235215679, -10.00000000000000000 ) ) ;
#88090=AXIS2_PLACEMENT_3D ( 'NONE', #2815, #49388, #71715 ) ;
#88095=CARTESIAN_POINT ( 'NONE',  ( -19.65312891409030271, 93.06504152958497400, 10.00000000000000888 ) ) ;
#88101=CARTESIAN_POINT ( 'NONE',  ( -14.95575157760114671, 40.24948350530962671, 59.99999999999999289 ) ) ;
#88102=ORIENTED_EDGE ( 'NONE', *, *, #38452, .F. ) ;
#88103=CARTESIAN_POINT ( 'NONE',  ( -34.42581292930597670, 25.91608375674935161, 10.00000000000000000 ) ) ;
#88105=DIRECTION ( 'NONE',  ( 0.6361630342459738685, -0.7715546603183444097, 0.000000000000000000 ) ) ;
#88107=LINE ( 'NONE', #26742, #70374 ) ;
#88109=ORIENTED_EDGE ( 'NONE', *, *, #40794, .F. ) ;
#88115=ORIENTED_EDGE ( 'NONE', *, *, #83453, .F. ) ;
#88116=ORIENTED_EDGE ( 'NONE', *, *, #92565, .F. ) ;
#88123=CARTESIAN_POINT ( 'NONE',  ( 48.32408078245681793, 82.80331927372955647, -10.00000000000000000 ) ) ;
#88128=CARTESIAN_POINT ( 'NONE',  ( -48.71813016832984289, 30.75580926756359901, -10.00000000000000000 ) ) ;
#88129=CARTESIAN_POINT ( 'NONE',  ( 31.12960416526798824, 44.88710030135629836, 10.00000000000000000 ) ) ;
#88132=CARTESIAN_POINT ( 'NONE',  ( -40.14225747417106760, 26.13077817479420872, 10.00000000000000000 ) ) ;
#88135=ORIENTED_EDGE ( 'NONE', *, *, #33579, .T. ) ;
#88137=DIRECTION ( 'NONE',  ( 0.4458072818673325943, 0.8951289669282637140, 0.000000000000000000 ) ) ;
#88144=CARTESIAN_POINT ( 'NONE',  ( 20.94141239725287917, 35.71947554534623492, 10.00000000000000000 ) ) ;
#88145=DIRECTION ( 'NONE',  ( -0.9756173257765569096, -0.2194785493951510180, 0.000000000000000000 ) ) ;
#88151=LINE ( 'NONE', #38604, #85199 ) ;
#88154=ORIENTED_EDGE ( 'NONE', *, *, #23401, .T. ) ;
#88161=VECTOR ( 'NONE', #48897, 1000.000000000000000 ) ;
#88163=DIRECTION ( 'NONE',  ( -1.000000000000000000, 0.000000000000000000, 0.000000000000000000 ) ) ;
#88171=AXIS2_PLACEMENT_3D ( 'NONE', #66738, #75870, #6449 ) ;
#88198=EDGE_CURVE ( 'NONE', #41047, #95263, #86346, .T. ) ;
#88199=LINE ( 'NONE', #80586, #67731 ) ;
#88203=DIRECTION ( 'NONE',  ( -0.7911563084720435457, -0.6116140086401625764, 0.000000000000000000 ) ) ;
#88206=VERTEX_POINT ( 'NONE', #14878 ) ;
#88207=CARTESIAN_POINT ( 'NONE',  ( -18.15312891409030627, 78.77562236714182120, 13.81405534229504894 ) ) ;
#88216=PLANE ( 'NONE',  #24666 ) ;
#88220=LINE ( 'NONE', #56755, #38728 ) ;
#88222=EDGE_CURVE ( 'NONE', #93711, #17411, #85330, .T. ) ;
#88223=ORIENTED_EDGE ( 'NONE', *, *, #90442, .F. ) ;
#88227=CARTESIAN_POINT ( 'NONE',  ( 48.83428215874786815, 87.09189275153327969, -10.00000000000000000 ) ) ;
#88229=VERTEX_POINT ( 'NONE', #8785 ) ;
#88230=ORIENTED_EDGE ( 'NONE', *, *, #540, .F. ) ;
#88231=EDGE_CURVE ( 'NONE', #60917, #33333, #14235, .T. ) ;
#88235=VERTEX_POINT ( 'NONE', #55363 ) ;
#88241=VECTOR ( 'NONE', #64221, 1000.000000000000000 ) ;
#88244=DIRECTION ( 'NONE',  ( 1.000000000000000000, 0.000000000000000000, 0.000000000000000000 ) ) ;
#88250=FACE_BOUND ( 'NONE', #7986, .T. ) ;
#88252=EDGE_CURVE ( 'NONE', #9589, #78857, #85857, .T. ) ;
#88270=DIRECTION ( 'NONE',  ( -0.7646402761590023189, -0.6444573283588951318, 0.000000000000000000 ) ) ;
#88274=ORIENTED_EDGE ( 'NONE', *, *, #59808, .F. ) ;
#88289=DIRECTION ( 'NONE',  ( -0.7715546603183375263, -0.6361630342459821952, 0.000000000000000000 ) ) ;
#88343=VECTOR ( 'NONE', #5610, 1000.000000000000000 ) ;
#88351=CARTESIAN_POINT ( 'NONE',  ( 45.34926676561319425, 66.39822172987334170, 10.00000000000000000 ) ) ;
#88355=EDGE_CURVE ( 'NONE', #99043, #28862, #28468, .T. ) ;
#88357=DIRECTION ( 'NONE',  ( 1.000000000000000000, 0.000000000000000000, 0.000000000000000000 ) ) ;
#88362=ORIENTED_EDGE ( 'NONE', *, *, #73932, .T. ) ;
#88366=ADVANCED_FACE ( 'NONE', ( #52752 ), #21379, .F. ) ;
#88368=ORIENTED_EDGE ( 'NONE', *, *, #86915, .F. ) ;
#88379=ORIENTED_EDGE ( 'NONE', *, *, #16964, .F. ) ;
#88381=AXIS2_PLACEMENT_3D ( 'NONE', #70213, #47415, #72250 ) ;
#88384=ORIENTED_EDGE ( 'NONE', *, *, #63337, .T. ) ;
#88396=CARTESIAN_POINT ( 'NONE',  ( 48.74043828842092552, 100.0309547576005258, -10.00000000000000000 ) ) ;
#88403=EDGE_CURVE ( 'NONE', #26239, #60221, #58850, .T. ) ;
#88408=DIRECTION ( 'NONE',  ( -0.000000000000000000, 0.000000000000000000, -1.000000000000000000 ) ) ;
#88409=DIRECTION ( 'NONE',  ( -0.9008877160804935613, -0.4340522123146846045, 0.000000000000000000 ) ) ;
#88414=CARTESIAN_POINT ( 'NONE',  ( -16.10531488956837975, 22.89493580087430402, 10.00000000000000000 ) ) ;
#88417=VECTOR ( 'NONE', #75915, 999.9999999999998863 ) ;
#88419=ORIENTED_EDGE ( 'NONE', *, *, #16284, .F. ) ;
#88424=AXIS2_PLACEMENT_3D ( 'NONE', #75616, #36098, #75130 ) ;
#88426=DIRECTION ( 'NONE',  ( 1.000000000000000000, 0.000000000000000000, 0.000000000000000000 ) ) ;
#88435=CARTESIAN_POINT ( 'NONE',  ( -70.92467617367975663, 45.40763453331954480, 10.00000000000000000 ) ) ;
#88446=ORIENTED_EDGE ( 'NONE', *, *, #96175, .F. ) ;
#88447=AXIS2_PLACEMENT_3D ( 'NONE', #17208, #55197, #9123 ) ;
#88458=LINE ( 'NONE', #87962, #51348 ) ;
#88468=CARTESIAN_POINT ( 'NONE',  ( 39.00902500372484383, 91.81115952553612658, 59.99999999999999289 ) ) ;
#88474=ORIENTED_EDGE ( 'NONE', *, *, #73488, .F. ) ;
#88482=PLANE ( 'NONE',  #46760 ) ;
#88483=ORIENTED_EDGE ( 'NONE', *, *, #73774, .F. ) ;
#88486=AXIS2_PLACEMENT_3D ( 'NONE', #99778, #61253, #30370 ) ;
#88489=AXIS2_PLACEMENT_3D ( 'NONE', #8953, #87535, #78372 ) ;
#88495=CARTESIAN_POINT ( 'NONE',  ( -19.65312891409030271, 93.06504152958497400, 177.5919119679930134 ) ) ;
#88497=CARTESIAN_POINT ( 'NONE',  ( 28.29029450517493061, 115.7140298976778325, 59.99999999999999289 ) ) ;
#88506=CARTESIAN_POINT ( 'NONE',  ( 38.65784837781280459, 56.65029301956751340, -10.00000000000000000 ) ) ;
#88511=EDGE_CURVE ( 'NONE', #28623, #27644, #46542, .T. ) ;
#88517=CARTESIAN_POINT ( 'NONE',  ( 46.88368875251780565, 110.3874725885333135, -10.00000000000000000 ) ) ;
#88522=CIRCLE ( 'NONE', #85236, 14.99999999999967848 ) ;
#88523=CARTESIAN_POINT ( 'NONE',  ( 43.53831125515428369, 65.97156238185917232, 10.00000000000000000 ) ) ;
#88538=VERTEX_POINT ( 'NONE', #3098 ) ;
#88544=LINE ( 'NONE', #43367, #98405 ) ;
#88551=DIRECTION ( 'NONE',  ( 0.000000000000000000, 0.000000000000000000, 1.000000000000000000 ) ) ;
#88562=EDGE_CURVE ( 'NONE', #77615, #55413, #71978, .T. ) ;
#88566=VECTOR ( 'NONE', #58670, 1000.000000000000114 ) ;
#88567=CYLINDRICAL_SURFACE ( 'NONE', #82403, 70.00000000000002842 ) ;
#88569=EDGE_CURVE ( 'NONE', #90851, #84918, #59741, .T. ) ;
#88579=CARTESIAN_POINT ( 'NONE',  ( 44.85937643310610667, 116.8208962945185050, -10.00000000000000000 ) ) ;
#88581=EDGE_LOOP ( 'NONE', ( #45326, #49966, #14546, #88931 ) ) ;
#88586=DIRECTION ( 'NONE',  ( 1.000000000000000000, 0.000000000000000000, 0.000000000000000000 ) ) ;
#88594=EDGE_LOOP ( 'NONE', ( #79236, #99938, #6562, #7451 ) ) ;
#88598=CARTESIAN_POINT ( 'NONE',  ( 32.30839531297598910, 123.0650415295850593, 60.00000000000000000 ) ) ;
#88599=LINE ( 'NONE', #21505, #80807 ) ;
#88619=CARTESIAN_POINT ( 'NONE',  ( 45.11483101423404918, 69.99284853207299761, -10.00000000000000000 ) ) ;
#88625=VERTEX_POINT ( 'NONE', #52636 ) ;
#88626=DIRECTION ( 'NONE',  ( -1.000000000000000000, 0.000000000000000000, 0.000000000000000000 ) ) ;
#88633=ORIENTED_EDGE ( 'NONE', *, *, #76944, .F. ) ;
#88642=AXIS2_PLACEMENT_3D ( 'NONE', #35896, #52586, #75929 ) ;
#88644=LINE ( 'NONE', #19209, #7418 ) ;
#88645=VERTEX_POINT ( 'NONE', #82614 ) ;
#88658=CYLINDRICAL_SURFACE ( 'NONE', #77220, 70.00000000000002842 ) ;
#88660=DIRECTION ( 'NONE',  ( -1.000000000000000000, 0.000000000000000000, 0.000000000000000000 ) ) ;
#88662=LINE ( 'NONE', #9104, #93142 ) ;
#88664=VECTOR ( 'NONE', #59692, 1000.000000000000000 ) ;
#88675=CARTESIAN_POINT ( 'NONE',  ( -65.03992292888628413, 39.77302590755693501, -10.00000000000000000 ) ) ;
#88681=VERTEX_POINT ( 'NONE', #6052 ) ;
#88697=CARTESIAN_POINT ( 'NONE',  ( -0.7215821717578424499, 65.74988880085649612, -10.00000000000000000 ) ) ;
#88698=CIRCLE ( 'NONE', #35277, 70.00000000000001421 ) ;
#88699=FACE_OUTER_BOUND ( 'NONE', #91167, .T. ) ;
#88706=CARTESIAN_POINT ( 'NONE',  ( -16.51533461259688806, 83.20563776615510676, 14.84223041658741060 ) ) ;
#88710=VECTOR ( 'NONE', #46529, 1000.000000000000000 ) ;
#88723=ORIENTED_EDGE ( 'NONE', *, *, #21506, .F. ) ;
#88728=ORIENTED_EDGE ( 'NONE', *, *, #49180, .T. ) ;
#88734=VERTEX_POINT ( 'NONE', #99761 ) ;
#88745=ORIENTED_EDGE ( 'NONE', *, *, #44500, .F. ) ;
#88749=EDGE_CURVE ( 'NONE', #46305, #68766, #70343, .T. ) ;
#88751=EDGE_LOOP ( 'NONE', ( #88135, #93565, #78296, #24002 ) ) ;
#88752=CARTESIAN_POINT ( 'NONE',  ( -73.83803415018344651, 50.74234351129840093, 10.00000000000000000 ) ) ;
#88759=VECTOR ( 'NONE', #88203, 1000.000000000000000 ) ;
#88765=DIRECTION ( 'NONE',  ( 0.9522021074858112444, 0.3054687324417666994, 0.000000000000000000 ) ) ;
#88773=ORIENTED_EDGE ( 'NONE', *, *, #85678, .T. ) ;
#88775=AXIS2_PLACEMENT_3D ( 'NONE', #14790, #91330, #52290 ) ;
#88777=ORIENTED_EDGE ( 'NONE', *, *, #73695, .F. ) ;
#88783=CYLINDRICAL_SURFACE ( 'NONE', #55067, 70.00000000000002842 ) ;
#88790=CARTESIAN_POINT ( 'NONE',  ( 48.60927726968589013, 109.6985806698937012, -10.00000000000000000 ) ) ;
#88791=CIRCLE ( 'NONE', #17488, 70.00000000000001421 ) ;
#88798=EDGE_CURVE ( 'NONE', #10180, #2192, #53635, .T. ) ;
#88801=DIRECTION ( 'NONE',  ( 0.9995565931350004485, 0.02977611660964677234, 0.000000000000000000 ) ) ;
#88808=ORIENTED_EDGE ( 'NONE', *, *, #70203, .F. ) ;
#88835=CARTESIAN_POINT ( 'NONE',  ( 6.089871667348707440, 48.19321075732142390, 59.99999999999999289 ) ) ;
#88850=AXIS2_PLACEMENT_3D ( 'NONE', #89947, #45292, #76226 ) ;
#88859=VERTEX_POINT ( 'NONE', #30351 ) ;
#88860=VECTOR ( 'NONE', #67480, 1000.000000000000227 ) ;
#88863=CARTESIAN_POINT ( 'NONE',  ( -19.65312891409030271, 93.06504152958497400, -10.00000000000000888 ) ) ;
#88865=ORIENTED_EDGE ( 'NONE', *, *, #1085, .T. ) ;
#88868=EDGE_LOOP ( 'NONE', ( #9940, #54114, #92599, #59622 ) ) ;
#88869=DIRECTION ( 'NONE',  ( 0.3693965786901519111, -0.9292718480896805522, 0.000000000000000000 ) ) ;
#88873=VECTOR ( 'NONE', #94758, 1000.000000000000000 ) ;
#88881=VERTEX_POINT ( 'NONE', #91684 ) ;
#88883=EDGE_CURVE ( 'NONE', #50922, #19773, #39423, .T. ) ;
#88884=ORIENTED_EDGE ( 'NONE', *, *, #19225, .F. ) ;
#88891=CARTESIAN_POINT ( 'NONE',  ( 19.18375657693640335, 36.32959363016014720, 10.00000000000000000 ) ) ;
#88897=ORIENTED_EDGE ( 'NONE', *, *, #57683, .F. ) ;
#88898=LINE ( 'NONE', #71653, #51237 ) ;
#88901=CARTESIAN_POINT ( 'NONE',  ( 30.54350413710242051, 75.98152451519752049, 59.99999999999999289 ) ) ;
#88909=FACE_OUTER_BOUND ( 'NONE', #24612, .T. ) ;
#88910=ADVANCED_FACE ( 'NONE', ( #38433 ), #53147, .F. ) ;
#88918=VECTOR ( 'NONE', #88409, 1000.000000000000000 ) ;
#88928=CARTESIAN_POINT ( 'NONE',  ( 47.49582885874516336, 78.29235751436857527, 10.00000000000000000 ) ) ;
#88929=ORIENTED_EDGE ( 'NONE', *, *, #29714, .F. ) ;
#88931=ORIENTED_EDGE ( 'NONE', *, *, #84658, .F. ) ;
#88935=CARTESIAN_POINT ( 'NONE',  ( 45.29894525614687950, 66.96469553601605185, 177.5919119679930134 ) ) ;
#88938=AXIS2_PLACEMENT_3D ( 'NONE', #81844, #74233, #15239 ) ;
#88946=ADVANCED_FACE ( 'NONE', ( #71367 ), #32348, .F. ) ;
#88959=ORIENTED_EDGE ( 'NONE', *, *, #21901, .F. ) ;
#88962=CARTESIAN_POINT ( 'NONE',  ( 1.233819684896646951, 25.98176417558038764, -10.00000000000000000 ) ) ;
#88966=DIRECTION ( 'NONE',  ( -0.000000000000000000, 0.000000000000000000, -1.000000000000000000 ) ) ;
#88970=ORIENTED_EDGE ( 'NONE', *, *, #72707, .F. ) ;
#88973=LINE ( 'NONE', #84325, #57205 ) ;
#88995=VECTOR ( 'NONE', #2944, 1000.000000000000000 ) ;
#88996=CARTESIAN_POINT ( 'NONE',  ( 46.74097198175142154, 116.0488203434314727, -10.00000000000000000 ) ) ;
#88999=LINE ( 'NONE', #28605, #59350 ) ;
#89003=AXIS2_PLACEMENT_3D ( 'NONE', #53470, #74932, #42497 ) ;
#89008=VERTEX_POINT ( 'NONE', #94190 ) ;
#89011=FACE_OUTER_BOUND ( 'NONE', #52024, .T. ) ;
#89013=CARTESIAN_POINT ( 'NONE',  ( 33.63407072503001416, 49.62913085183823370, -10.00000000000000000 ) ) ;
#89014=VECTOR ( 'NONE', #90005, 1000.000000000000114 ) ;
#89016=ORIENTED_EDGE ( 'NONE', *, *, #91671, .F. ) ;
#89020=CARTESIAN_POINT ( 'NONE',  ( 24.69086998626516305, 38.90223361192549589, -10.00000000000000000 ) ) ;
#89035=FACE_OUTER_BOUND ( 'NONE', #95738, .T. ) ;
#89040=EDGE_CURVE ( 'NONE', #69469, #98279, #24744, .T. ) ;
#89043=ORIENTED_EDGE ( 'NONE', *, *, #72853, .F. ) ;
#89050=CARTESIAN_POINT ( 'NONE',  ( -19.65312891409030271, 93.06504152958497400, 10.00000000000000888 ) ) ;
#89058=LINE ( 'NONE', #19105, #25728 ) ;
#89059=CARTESIAN_POINT ( 'NONE',  ( 26.15794687706369004, 39.79426100978996317, 10.00000000000000000 ) ) ;
#89068=AXIS2_PLACEMENT_3D ( 'NONE', #81638, #97818, #90242 ) ;
#89069=DIRECTION ( 'NONE',  ( 0.9972444261165168689, -0.07418594597050690020, 0.000000000000000000 ) ) ;
#89074=ADVANCED_FACE ( 'NONE', ( #56644 ), #78468, .T. ) ;
#89096=LINE ( 'NONE', #49032, #87471 ) ;
#89098=ADVANCED_FACE ( 'NONE', ( #63751 ), #56127, .F. ) ;
#89099=DIRECTION ( 'NONE',  ( 0.1783728972749306640, 0.9839629614562466209, 0.000000000000000000 ) ) ;
#89105=ORIENTED_EDGE ( 'NONE', *, *, #67817, .F. ) ;
#89109=VERTEX_POINT ( 'NONE', #5447 ) ;
#89122=ORIENTED_EDGE ( 'NONE', *, *, #78956, .F. ) ;
#89128=CARTESIAN_POINT ( 'NONE',  ( -40.67952639183666008, 27.60432558407080350, 10.00000000000000000 ) ) ;
#89131=VECTOR ( 'NONE', #54232, 1000.000000000000000 ) ;
#89133=DIRECTION ( 'NONE',  ( 0.000000000000000000, 0.000000000000000000, 1.000000000000000000 ) ) ;
#89135=ORIENTED_EDGE ( 'NONE', *, *, #20917, .T. ) ;
#89136=FACE_OUTER_BOUND ( 'NONE', #87610, .T. ) ;
#89145=ADVANCED_FACE ( 'NONE', ( #36330 ), #73852, .T. ) ;
#89146=DIRECTION ( 'NONE',  ( -0.9985437513708431689, -0.05394790633790857298, 0.000000000000000000 ) ) ;
#89149=EDGE_CURVE ( 'NONE', #35732, #43419, #4441, .T. ) ;
#89150=AXIS2_PLACEMENT_3D ( 'NONE', #35511, #65416, #96359 ) ;
#89152=PLANE ( 'NONE',  #65734 ) ;
#89153=DIRECTION ( 'NONE',  ( -0.1580495287025880657, -0.9874311856918890351, 0.000000000000000000 ) ) ;
#89154=ADVANCED_FACE ( 'NONE', ( #5939 ), #90596, .F. ) ;
#89158=FACE_OUTER_BOUND ( 'NONE', #34593, .T. ) ;
#89163=CARTESIAN_POINT ( 'NONE',  ( 30.96785900501025424, 44.34188169337050311, -10.00000000000000000 ) ) ;
#89171=PLANE ( 'NONE',  #21118 ) ;
#89172=CARTESIAN_POINT ( 'NONE',  ( -19.65312891409030271, 93.06504152958497400, 25.00000000000000000 ) ) ;
#89176=LINE ( 'NONE', #19723, #54735 ) ;
#89178=LINE ( 'NONE', #5875, #36589 ) ;
#89183=DIRECTION ( 'NONE',  ( -0.000000000000000000, -0.000000000000000000, 1.000000000000000000 ) ) ;
#89185=DIRECTION ( 'NONE',  ( -0.9140770918436990078, -0.4055404667435369426, 0.000000000000000000 ) ) ;
#89205=VECTOR ( 'NONE', #75716, 1000.000000000000114 ) ;
#89206=DIRECTION ( 'NONE',  ( -0.9689885751534065284, -0.2471055264905481497, 0.000000000000000000 ) ) ;
#89208=DIRECTION ( 'NONE',  ( -0.8279987035736700030, -0.5607300124661794838, 0.000000000000000000 ) ) ;
#89209=LINE ( 'NONE', #72472, #9366 ) ;
#89213=DIRECTION ( 'NONE',  ( 0.3666034970181715757, -0.9303772761487930643, 0.000000000000000000 ) ) ;
#89216=EDGE_LOOP ( 'NONE', ( #87442, #5870, #19254, #69649 ) ) ;
#89219=DIRECTION ( 'NONE',  ( 1.000000000000000000, -2.158987274672848517E-13, 0.000000000000000000 ) ) ;
#89226=CYLINDRICAL_SURFACE ( 'NONE', #46189, 70.00000000000002842 ) ;
#89236=FACE_OUTER_BOUND ( 'NONE', #90249, .T. ) ;
#89238=VERTEX_POINT ( 'NONE', #50531 ) ;
#89239=CARTESIAN_POINT ( 'NONE',  ( -19.65312891409030271, 93.06504152958497400, 177.5919119679930134 ) ) ;
#89241=DIRECTION ( 'NONE',  ( 1.000000000000000000, 0.000000000000000000, 0.000000000000000000 ) ) ;
#89259=ORIENTED_EDGE ( 'NONE', *, *, #55712, .F. ) ;
#89267=EDGE_CURVE ( 'NONE', #79622, #72764, #40689, .T. ) ;
#89273=DIRECTION ( 'NONE',  ( -1.000000000000000000, 0.000000000000000000, 0.000000000000000000 ) ) ;
#89282=DIRECTION ( 'NONE',  ( 0.000000000000000000, -0.000000000000000000, -1.000000000000000000 ) ) ;
#89283=ORIENTED_EDGE ( 'NONE', *, *, #63640, .F. ) ;
#89286=PLANE ( 'NONE',  #64562 ) ;
#89287=CARTESIAN_POINT ( 'NONE',  ( -42.47074677134370546, 28.21475011077167849, 10.00000000000000000 ) ) ;
#89306=EDGE_CURVE ( 'NONE', #57725, #28914, #45904, .T. ) ;
#89313=FACE_OUTER_BOUND ( 'NONE', #12996, .T. ) ;
#89317=CARTESIAN_POINT ( 'NONE',  ( 49.09245556086620610, 93.56363653685789927, -10.00000000000000000 ) ) ;
#89333=CARTESIAN_POINT ( 'NONE',  ( 4.394486334025504704, 45.80786630299208895, 59.99999999999999289 ) ) ;
#89340=ORIENTED_EDGE ( 'NONE', *, *, #82372, .F. ) ;
#89344=ORIENTED_EDGE ( 'NONE', *, *, #34155, .F. ) ;
#89351=DIRECTION ( 'NONE',  ( -0.000000000000000000, -0.000000000000000000, -1.000000000000000000 ) ) ;
#89358=DIRECTION ( 'NONE',  ( -0.000000000000000000, 0.000000000000000000, 1.000000000000000000 ) ) ;
#89360=ORIENTED_EDGE ( 'NONE', *, *, #66201, .T. ) ;
#89365=ADVANCED_FACE ( 'NONE', ( #37323 ), #55871, .F. ) ;
#89366=EDGE_CURVE ( 'NONE', #2381, #30665, #54004, .T. ) ;
#89372=DIRECTION ( 'NONE',  ( 0.3887219701524006754, 0.9213551052231903071, 0.000000000000000000 ) ) ;
#89373=EDGE_LOOP ( 'NONE', ( #44565, #45100, #55865, #57661 ) ) ;
#89374=LINE ( 'NONE', #50801, #93389 ) ;
#89385=LINE ( 'NONE', #54797, #70487 ) ;
#89386=AXIS2_PLACEMENT_3D ( 'NONE', #69346, #53632, #7042 ) ;
#89390=VERTEX_POINT ( 'NONE', #9828 ) ;
#89394=CARTESIAN_POINT ( 'NONE',  ( 28.65130504220245555, 111.5816539614736485, 59.99999999999999289 ) ) ;
#89412=ORIENTED_EDGE ( 'NONE', *, *, #74668, .T. ) ;
#89416=DIRECTION ( 'NONE',  ( 0.01068548594337171906, -0.9999429085653609439, 0.000000000000000000 ) ) ;
#89418=CARTESIAN_POINT ( 'NONE',  ( -19.65312891409030271, 93.06504152958497400, 60.00000000000000000 ) ) ;
#89425=ADVANCED_FACE ( 'NONE', ( #6925 ), #37814, .F. ) ;
#89432=CARTESIAN_POINT ( 'NONE',  ( 43.25185672232382217, 62.35734246106904521, 10.00000000000000000 ) ) ;
#89440=LINE ( 'NONE', #67069, #75029 ) ;
#89452=ORIENTED_EDGE ( 'NONE', *, *, #49300, .F. ) ;
#89455=VECTOR ( 'NONE', #85589, 1000.000000000000000 ) ;
#89456=EDGE_CURVE ( 'NONE', #83671, #7444, #78721, .T. ) ;
#89458=EDGE_CURVE ( 'NONE', #84833, #98290, #72558, .T. ) ;
#89466=CARTESIAN_POINT ( 'NONE',  ( 46.08672700828314817, 69.01776843458344501, -10.00000000000000000 ) ) ;
#89467=ORIENTED_EDGE ( 'NONE', *, *, #84497, .F. ) ;
#89474=CIRCLE ( 'NONE', #44115, 0.1418229129681522482 ) ;
#89479=LINE ( 'NONE', #20038, #50479 ) ;
#89483=EDGE_LOOP ( 'NONE', ( #4829, #91950, #43065, #65417 ) ) ;
#89487=ORIENTED_EDGE ( 'NONE', *, *, #36677, .T. ) ;
#89496=LINE ( 'NONE', #49438, #80948 ) ;
#89501=VERTEX_POINT ( 'NONE', #59879 ) ;
#89502=CARTESIAN_POINT ( 'NONE',  ( -2.073866539663252073, 26.60322154129611505, 10.00000000000000000 ) ) ;
#89503=ORIENTED_EDGE ( 'NONE', *, *, #34139, .F. ) ;
#89508=EDGE_CURVE ( 'NONE', #32335, #23143, #93, .T. ) ;
#89509=LINE ( 'NONE', #88517, #10993 ) ;
#89511=DIRECTION ( 'NONE',  ( -1.000000000000000000, 0.000000000000000000, 0.000000000000000000 ) ) ;
#89521=LINE ( 'NONE', #33794, #71301 ) ;
#89522=FACE_OUTER_BOUND ( 'NONE', #50068, .T. ) ;
#89525=VECTOR ( 'NONE', #3064, 1000.000000000000000 ) ;
#89526=CARTESIAN_POINT ( 'NONE',  ( 8.004356468201564212, 74.63722199011714054, -10.00000000000000000 ) ) ;
#89529=ORIENTED_EDGE ( 'NONE', *, *, #45133, .F. ) ;
#89547=DIRECTION ( 'NONE',  ( -0.000000000000000000, -0.000000000000000000, 1.000000000000000000 ) ) ;
#89550=LINE ( 'NONE', #5400, #9250 ) ;
#89551=DIRECTION ( 'NONE',  ( 1.000000000000000000, 0.000000000000000000, 0.000000000000000000 ) ) ;
#89561=DIRECTION ( 'NONE',  ( 0.000000000000000000, -0.000000000000000000, 1.000000000000000000 ) ) ;
#89564=VERTEX_POINT ( 'NONE', #22876 ) ;
#89566=DIRECTION ( 'NONE',  ( 0.001368469433193686413, -0.9999990636452668058, 0.000000000000000000 ) ) ;
#89569=EDGE_CURVE ( 'NONE', #166, #8200, #88791, .T. ) ;
#89571=EDGE_CURVE ( 'NONE', #22609, #31605, #23993, .T. ) ;
#89579=ORIENTED_EDGE ( 'NONE', *, *, #69593, .F. ) ;
#89580=CARTESIAN_POINT ( 'NONE',  ( -19.68164973832074338, 92.92611600555152052, 59.99999999999999289 ) ) ;
#89582=ORIENTED_EDGE ( 'NONE', *, *, #37923, .T. ) ;
#89596=DIRECTION ( 'NONE',  ( -0.03304531753666254540, -0.9994538543569189137, 0.000000000000000000 ) ) ;
#89604=DIRECTION ( 'NONE',  ( -1.000000000000000000, 0.000000000000000000, 0.000000000000000000 ) ) ;
#89608=LINE ( 'NONE', #57643, #30202 ) ;
#89610=CARTESIAN_POINT ( 'NONE',  ( 49.17298586869600996, 105.8308522718264584, -10.00000000000000000 ) ) ;
#89614=EDGE_CURVE ( 'NONE', #27521, #36145, #99724, .T. ) ;
#89616=ORIENTED_EDGE ( 'NONE', *, *, #39192, .T. ) ;
#89617=CARTESIAN_POINT ( 'NONE',  ( 15.48905510666703478, 53.35892832886757020, 59.99999999999999289 ) ) ;
#89622=EDGE_CURVE ( 'NONE', #14275, #1030, #45980, .T. ) ;
#89627=ORIENTED_EDGE ( 'NONE', *, *, #27080, .F. ) ;
#89629=CARTESIAN_POINT ( 'NONE',  ( -54.25007008209492199, 32.21233689110872689, -10.00000000000000000 ) ) ;
#89648=LINE ( 'NONE', #97234, #28469 ) ;
#89652=EDGE_CURVE ( 'NONE', #1959, #38287, #30310, .T. ) ;
#89658=CARTESIAN_POINT ( 'NONE',  ( -35.39007723419273788, 42.43010318828366678, 59.99999999999999289 ) ) ;
#89662=DIRECTION ( 'NONE',  ( -0.6139877827364750296, 0.7893155279419930004, 0.000000000000000000 ) ) ;
#89667=ORIENTED_EDGE ( 'NONE', *, *, #41483, .F. ) ;
#89671=PLANE ( 'NONE',  #6289 ) ;
#89686=EDGE_CURVE ( 'NONE', #68396, #19346, #100021, .T. ) ;
#89687=FACE_OUTER_BOUND ( 'NONE', #51520, .T. ) ;
#89690=CARTESIAN_POINT ( 'NONE',  ( -69.50121871515369776, 62.11365277976253907, 59.99999999999999289 ) ) ;
#89694=CARTESIAN_POINT ( 'NONE',  ( -19.65312891409030271, 93.06504152958497400, 10.00000000000000888 ) ) ;
#89695=CARTESIAN_POINT ( 'NONE',  ( 47.39496755818312579, 108.2889530649357681, -10.00000000000000000 ) ) ;
#89697=ORIENTED_EDGE ( 'NONE', *, *, #8510, .F. ) ;
#89698=DIRECTION ( 'NONE',  ( -0.6386832404231509441, -0.7694697644498993405, 0.000000000000000000 ) ) ;
#89700=DIRECTION ( 'NONE',  ( -1.000000000000000000, 0.000000000000000000, 0.000000000000000000 ) ) ;
#89703=CARTESIAN_POINT ( 'NONE',  ( 34.81516168915606357, 51.10768172523390973, -10.00000000000000000 ) ) ;
#89708=CARTESIAN_POINT ( 'NONE',  ( -57.46197106626858186, 34.15416430719361074, 10.00000000000000000 ) ) ;
#89709=PLANE ( 'NONE',  #13335 ) ;
#89717=DIRECTION ( 'NONE',  ( 1.000000000000000000, 0.000000000000000000, 0.000000000000000000 ) ) ;
#89721=DIRECTION ( 'NONE',  ( -0.9042435392811277728, -0.4270171210482544000, 0.000000000000000000 ) ) ;
#89727=EDGE_LOOP ( 'NONE', ( #80094, #94467 ) ) ;
#89729=ORIENTED_EDGE ( 'NONE', *, *, #8174, .T. ) ;
#89739=VERTEX_POINT ( 'NONE', #78424 ) ;
#89744=CARTESIAN_POINT ( 'NONE',  ( -19.65312891409030271, 93.06504152958497400, 177.5919119679930134 ) ) ;
#89748=LINE ( 'NONE', #65892, #916 ) ;
#89749=ADVANCED_FACE ( 'NONE', ( #39380 ), #70814, .F. ) ;
#89750=PLANE ( 'NONE',  #36498 ) ;
#89757=CARTESIAN_POINT ( 'NONE',  ( 43.53831125515428369, 65.97156238185917232, -10.00000000000000000 ) ) ;
#89759=LINE ( 'NONE', #20328, #50230 ) ;
#89775=VERTEX_POINT ( 'NONE', #55091 ) ;
#89790=AXIS2_PLACEMENT_3D ( 'NONE', #81395, #11963, #50441 ) ;
#89798=ADVANCED_FACE ( 'NONE', ( #62184 ), #48518, .T. ) ;
#89802=VECTOR ( 'NONE', #64733, 1000.000000000000000 ) ;
#89811=CARTESIAN_POINT ( 'NONE',  ( 24.19030146973739193, 38.49624447322263876, 10.00000000000000000 ) ) ;
#89812=CARTESIAN_POINT ( 'NONE',  ( -59.65739779450132829, 37.15562860896453401, -10.00000000000000000 ) ) ;
#89832=ORIENTED_EDGE ( 'NONE', *, *, #70539, .F. ) ;
#89839=ORIENTED_EDGE ( 'NONE', *, *, #5915, .T. ) ;
#89842=DIRECTION ( 'NONE',  ( -1.000000000000000000, 0.000000000000000000, 0.000000000000000000 ) ) ;
#89847=DIRECTION ( 'NONE',  ( -0.000000000000000000, -0.000000000000000000, -1.000000000000000000 ) ) ;
#89852=DIRECTION ( 'NONE',  ( -0.000000000000000000, 0.000000000000000000, -1.000000000000000000 ) ) ;
#89858=VERTEX_POINT ( 'NONE', #15588 ) ;
#89863=DIRECTION ( 'NONE',  ( 0.000000000000000000, 0.000000000000000000, 1.000000000000000000 ) ) ;
#89865=CARTESIAN_POINT ( 'NONE',  ( 32.35804664341760883, 67.52305595790635095, 59.99999999999999289 ) ) ;
#89870=AXIS2_PLACEMENT_3D ( 'NONE', #36704, #67611, #78222 ) ;
#89887=ORIENTED_EDGE ( 'NONE', *, *, #7264, .T. ) ;
#89888=ORIENTED_EDGE ( 'NONE', *, *, #69795, .F. ) ;
#89901=DIRECTION ( 'NONE',  ( 0.000000000000000000, -0.000000000000000000, 1.000000000000000000 ) ) ;
#89907=EDGE_CURVE ( 'NONE', #72231, #58877, #82271, .T. ) ;
#89913=ORIENTED_EDGE ( 'NONE', *, *, #21394, .F. ) ;
#89914=AXIS2_PLACEMENT_3D ( 'NONE', #20063, #12971, #35745 ) ;
#89929=LINE ( 'NONE', #20507, #70145 ) ;
#89935=VECTOR ( 'NONE', #92793, 1000.000000000000000 ) ;
#89945=ORIENTED_EDGE ( 'NONE', *, *, #21827, .T. ) ;
#89947=CARTESIAN_POINT ( 'NONE',  ( -18.31116180715439512, 22.81812098060338911, -10.00000000000000000 ) ) ;
#89950=PLANE ( 'NONE',  #68500 ) ;
#89953=LINE ( 'NONE', #12943, #25392 ) ;
#89961=EDGE_LOOP ( 'NONE', ( #41729, #60402, #29604, #83496 ) ) ;
#89967=FACE_OUTER_BOUND ( 'NONE', #15932, .T. ) ;
#89971=LINE ( 'NONE', #67623, #56002 ) ;
#89972=DIRECTION ( 'NONE',  ( -0.000000000000000000, -0.000000000000000000, -1.000000000000000000 ) ) ;
#89976=ORIENTED_EDGE ( 'NONE', *, *, #86789, .F. ) ;
#89979=VERTEX_POINT ( 'NONE', #12015 ) ;
#89980=AXIS2_PLACEMENT_3D ( 'NONE', #54061, #61671, #37865 ) ;
#89984=ORIENTED_EDGE ( 'NONE', *, *, #79857, .F. ) ;
#89991=AXIS2_PLACEMENT_3D ( 'NONE', #13931, #44810, #32107 ) ;
#89995=ORIENTED_EDGE ( 'NONE', *, *, #84876, .F. ) ;
#90005=DIRECTION ( 'NONE',  ( -0.6313854049612632746, -0.7754691937155863135, 0.000000000000000000 ) ) ;
#90008=ORIENTED_EDGE ( 'NONE', *, *, #66791, .F. ) ;
#90011=DIRECTION ( 'NONE',  ( -0.6602847420308683990, -0.7510153523339117010, 0.000000000000000000 ) ) ;
#90012=CARTESIAN_POINT ( 'NONE',  ( -73.66720466879951346, 50.53642055324488780, -10.00000000000000000 ) ) ;
#90013=LINE ( 'NONE', #82914, #59684 ) ;
#90016=VECTOR ( 'NONE', #56327, 1000.000000000000000 ) ;
#90019=LINE ( 'NONE', #43864, #80718 ) ;
#90040=EDGE_CURVE ( 'NONE', #72111, #65613, #71667, .T. ) ;
#90046=AXIS2_PLACEMENT_3D ( 'NONE', #18793, #34478, #88244 ) ;
#90050=ORIENTED_EDGE ( 'NONE', *, *, #39996, .F. ) ;
#90053=VECTOR ( 'NONE', #96478, 1000.000000000000000 ) ;
#90059=AXIS2_PLACEMENT_3D ( 'NONE', #58639, #57150, #88626 ) ;
#90063=DIRECTION ( 'NONE',  ( -0.3374500364938434194, -0.9413434404457831084, 0.000000000000000000 ) ) ;
#90068=ORIENTED_EDGE ( 'NONE', *, *, #97350, .T. ) ;
#90069=CARTESIAN_POINT ( 'NONE',  ( -19.65312891409030271, 93.06504152958497400, -10.00000000000000888 ) ) ;
#90072=DIRECTION ( 'NONE',  ( 0.000000000000000000, 0.000000000000000000, 1.000000000000000000 ) ) ;
#90073=ORIENTED_EDGE ( 'NONE', *, *, #84079, .T. ) ;
#90084=CARTESIAN_POINT ( 'NONE',  ( 46.22371820283660782, 112.7232458147606451, 10.00000000000000000 ) ) ;
#90085=AXIS2_PLACEMENT_3D ( 'NONE', #34070, #69674, #77283 ) ;
#90086=ORIENTED_EDGE ( 'NONE', *, *, #12481, .T. ) ;
#90087=EDGE_LOOP ( 'NONE', ( #52158, #73622, #76594, #68607 ) ) ;
#90092=DIRECTION ( 'NONE',  ( -1.000000000000000000, 0.000000000000000000, 0.000000000000000000 ) ) ;
#90093=DIRECTION ( 'NONE',  ( -0.3986482622784278673, -0.9171038997749326738, 0.000000000000000000 ) ) ;
#90099=ORIENTED_EDGE ( 'NONE', *, *, #48115, .T. ) ;
#90100=CARTESIAN_POINT ( 'NONE',  ( 22.96769398916923777, 37.53608102203546792, 10.00000000000000000 ) ) ;
#90103=VERTEX_POINT ( 'NONE', #55412 ) ;
#90119=LINE ( 'NONE', #51582, #38317 ) ;
#90120=EDGE_LOOP ( 'NONE', ( #38852, #65172, #5676, #62594 ) ) ;
#90127=ADVANCED_FACE ( 'NONE', ( #63533 ), #25029, .F. ) ;
#90128=CIRCLE ( 'NONE', #20541, 0.1418229129681522482 ) ;
#90142=PLANE ( 'NONE',  #88642 ) ;
#90149=VECTOR ( 'NONE', #10313, 1000.000000000000114 ) ;
#90161=CARTESIAN_POINT ( 'NONE',  ( -47.77400264604317925, 41.56691441172057466, 59.99999999999999289 ) ) ;
#90170=EDGE_CURVE ( 'NONE', #68063, #47151, #90883, .T. ) ;
#90173=DIRECTION ( 'NONE',  ( -0.7082622432767082810, -0.7059494278973847958, 0.000000000000000000 ) ) ;
#90177=CARTESIAN_POINT ( 'NONE',  ( -2.073866539663252073, 26.60322154129611505, -10.00000000000000000 ) ) ;
#90184=FACE_OUTER_BOUND ( 'NONE', #67881, .T. ) ;
#90185=ORIENTED_EDGE ( 'NONE', *, *, #6479, .F. ) ;
#90186=CARTESIAN_POINT ( 'NONE',  ( -43.70040200909111405, 27.32518560721127798, 177.5919119679930134 ) ) ;
#90188=LINE ( 'NONE', #21254, #3872 ) ;
#90194=ORIENTED_EDGE ( 'NONE', *, *, #74528, .T. ) ;
#90205=ORIENTED_EDGE ( 'NONE', *, *, #26893, .T. ) ;
#90206=VECTOR ( 'NONE', #1371, 1000.000000000000000 ) ;
#90210=ORIENTED_EDGE ( 'NONE', *, *, #89622, .T. ) ;
#90213=LINE ( 'NONE', #51157, #74281 ) ;
#90224=ORIENTED_EDGE ( 'NONE', *, *, #6151, .F. ) ;
#90225=AXIS2_PLACEMENT_3D ( 'NONE', #234, #2253, #15925 ) ;
#90228=ORIENTED_EDGE ( 'NONE', *, *, #9839, .F. ) ;
#90230=DIRECTION ( 'NONE',  ( -0.000000000000000000, -0.000000000000000000, -1.000000000000000000 ) ) ;
#90232=PLANE ( 'NONE',  #9335 ) ;
#90233=CARTESIAN_POINT ( 'NONE',  ( -75.69529296620470404, 50.68926341652933587, -10.00000000000000000 ) ) ;
#90234=CARTESIAN_POINT ( 'NONE',  ( -68.29659580619643577, 42.72804590294295224, 177.5919119679930134 ) ) ;
#90236=ORIENTED_EDGE ( 'NONE', *, *, #20961, .F. ) ;
#90237=DIRECTION ( 'NONE',  ( -0.7884491381006394350, 0.6150999566154746745, 0.000000000000000000 ) ) ;
#90238=AXIS2_PLACEMENT_3D ( 'NONE', #64183, #95132, #46465 ) ;
#90240=PLANE ( 'NONE',  #77125 ) ;
#90241=VERTEX_POINT ( 'NONE', #7717 ) ;
#90242=DIRECTION ( 'NONE',  ( 0.3984034379158949979, -0.9172102815913020235, 0.000000000000000000 ) ) ;
#90246=CARTESIAN_POINT ( 'NONE',  ( -4.429217378738782962, 26.01694505731172313, 10.00000000000000000 ) ) ;
#90249=EDGE_LOOP ( 'NONE', ( #4749, #73504, #37094, #83860 ) ) ;
#90252=ORIENTED_EDGE ( 'NONE', *, *, #83628, .F. ) ;
#90256=EDGE_CURVE ( 'NONE', #68464, #85874, #76625, .T. ) ;
#90260=DIRECTION ( 'NONE',  ( 0.000000000000000000, 0.000000000000000000, 1.000000000000000000 ) ) ;
#90270=AXIS2_PLACEMENT_3D ( 'NONE', #28410, #27439, #72559 ) ;
#90271=VECTOR ( 'NONE', #68440, 1000.000000000000227 ) ;
#90281=VECTOR ( 'NONE', #85807, 1000.000000000000227 ) ;
#90303=VECTOR ( 'NONE', #29312, 1000.000000000000227 ) ;
#90309=FACE_OUTER_BOUND ( 'NONE', #43436, .T. ) ;
#90323=FACE_OUTER_BOUND ( 'NONE', #70095, .T. ) ;
#90330=VERTEX_POINT ( 'NONE', #25936 ) ;
#90331=DIRECTION ( 'NONE',  ( 1.000000000000000000, -1.003165804393444873E-13, 0.000000000000000000 ) ) ;
#90334=VERTEX_POINT ( 'NONE', #51198 ) ;
#90336=AXIS2_PLACEMENT_3D ( 'NONE', #96401, #87838, #18883 ) ;
#90339=EDGE_LOOP ( 'NONE', ( #17409, #91823, #24728, #18433 ) ) ;
#90344=AXIS2_PLACEMENT_3D ( 'NONE', #54655, #47072, #8583 ) ;
#90347=DIRECTION ( 'NONE',  ( 1.000000000000000000, 0.000000000000000000, 0.000000000000000000 ) ) ;
#90352=ORIENTED_EDGE ( 'NONE', *, *, #36752, .T. ) ;
#90356=LINE ( 'NONE', #58883, #13752 ) ;
#90358=CARTESIAN_POINT ( 'NONE',  ( 27.80861752939100029, 41.25950758903265836, 10.00000000000000000 ) ) ;
#90369=EDGE_LOOP ( 'NONE', ( #92707, #64673, #70342, #10870 ) ) ;
#90385=AXIS2_PLACEMENT_3D ( 'NONE', #32717, #1835, #46919 ) ;
#90386=EDGE_CURVE ( 'NONE', #26065, #51970, #11245, .T. ) ;
#90394=LINE ( 'NONE', #59923, #38496 ) ;
#90397=CARTESIAN_POINT ( 'NONE',  ( 37.67364948790085322, 52.89489741671173562, 177.5919119679930134 ) ) ;
#90398=ORIENTED_EDGE ( 'NONE', *, *, #48708, .F. ) ;
#90413=CARTESIAN_POINT ( 'NONE',  ( -19.65312891409030271, 93.06504152958497400, 60.00000000000000000 ) ) ;
#90415=AXIS2_PLACEMENT_3D ( 'NONE', #72895, #39934, #71382 ) ;
#90417=CIRCLE ( 'NONE', #3043, 45.00000000000000000 ) ;
#90420=DIRECTION ( 'NONE',  ( 0.000000000000000000, 0.000000000000000000, 1.000000000000000000 ) ) ;
#90428=AXIS2_PLACEMENT_3D ( 'NONE', #52291, #44676, #15780 ) ;
#90430=CARTESIAN_POINT ( 'NONE',  ( -54.21831688459418785, 33.63902229265146104, 10.00000000000000000 ) ) ;
#90435=CARTESIAN_POINT ( 'NONE',  ( 47.78135487164287554, 106.4364430393875267, -10.00000000000000000 ) ) ;
#90442=EDGE_CURVE ( 'NONE', #63506, #72984, #64432, .T. ) ;
#90446=VECTOR ( 'NONE', #28306, 1000.000000000000114 ) ;
#90451=DIRECTION ( 'NONE',  ( 0.000000000000000000, -0.000000000000000000, 1.000000000000000000 ) ) ;
#90457=LINE ( 'NONE', #3818, #51907 ) ;
#90460=ORIENTED_EDGE ( 'NONE', *, *, #78472, .F. ) ;
#90463=LINE ( 'NONE', #83340, #38573 ) ;
#90469=CARTESIAN_POINT ( 'NONE',  ( 13.43400709863221820, 31.08381733381234469, 10.00000000000000000 ) ) ;
#90470=ORIENTED_EDGE ( 'NONE', *, *, #50966, .T. ) ;
#90476=EDGE_LOOP ( 'NONE', ( #74396, #99379, #82753, #55612 ) ) ;
#90477=ORIENTED_EDGE ( 'NONE', *, *, #52628, .F. ) ;
#90479=ORIENTED_EDGE ( 'NONE', *, *, #99668, .F. ) ;
#90480=CARTESIAN_POINT ( 'NONE',  ( -45.06544009570465903, 71.64693071047494755, -10.00000000000000000 ) ) ;
#90482=CARTESIAN_POINT ( 'NONE',  ( -78.57153713424663977, 57.64153020465174393, 10.00000000000000000 ) ) ;
#90484=CARTESIAN_POINT ( 'NONE',  ( -27.77457187288641904, 24.79904599702367562, -10.00000000000000000 ) ) ;
#90486=CIRCLE ( 'NONE', #7926, 70.00000000000001421 ) ;
#90489=VECTOR ( 'NONE', #95455, 1000.000000000000114 ) ;
#90497=CARTESIAN_POINT ( 'NONE',  ( 40.37736971981244238, 56.55791953817036699, 10.00000000000000000 ) ) ;
#90507=AXIS2_PLACEMENT_3D ( 'NONE', #32209, #56510, #9933 ) ;
#90513=EDGE_CURVE ( 'NONE', #93866, #12312, #49889, .T. ) ;
#90523=VERTEX_POINT ( 'NONE', #92949 ) ;
#90524=DIRECTION ( 'NONE',  ( -1.000000000000000000, 0.000000000000000000, 0.000000000000000000 ) ) ;
#90525=DIRECTION ( 'NONE',  ( -0.000000000000000000, 0.000000000000000000, -1.000000000000000000 ) ) ;
#90533=FACE_OUTER_BOUND ( 'NONE', #20420, .T. ) ;
#90547=DIRECTION ( 'NONE',  ( 0.3074612162317589825, -0.9515606131578205895, 0.000000000000000000 ) ) ;
#90552=CIRCLE ( 'NONE', #85710, 0.1418229129680828593 ) ;
#90553=DIRECTION ( 'NONE',  ( -0.8903844177683322147, -0.4552093898365321412, 0.000000000000000000 ) ) ;
#90559=EDGE_CURVE ( 'NONE', #77091, #47670, #24519, .T. ) ;
#90573=EDGE_CURVE ( 'NONE', #8415, #31684, #9393, .T. ) ;
#90593=VECTOR ( 'NONE', #20017, 1000.000000000000114 ) ;
#90596=PLANE ( 'NONE',  #30365 ) ;
#90601=PLANE ( 'NONE',  #58463 ) ;
#90602=FACE_OUTER_BOUND ( 'NONE', #84344, .T. ) ;
#90616=EDGE_CURVE ( 'NONE', #54113, #32823, #32623, .T. ) ;
#90625=DIRECTION ( 'NONE',  ( -0.000000000000000000, 0.000000000000000000, -1.000000000000000000 ) ) ;
#90656=AXIS2_PLACEMENT_3D ( 'NONE', #68665, #36278, #22078 ) ;
#90683=EDGE_CURVE ( 'NONE', #9269, #30721, #2244, .T. ) ;
#90690=ORIENTED_EDGE ( 'NONE', *, *, #37699, .T. ) ;
#90699=DIRECTION ( 'NONE',  ( -0.000000000000000000, -0.000000000000000000, -1.000000000000000000 ) ) ;
#90709=ORIENTED_EDGE ( 'NONE', *, *, #68900, .T. ) ;
#90715=ORIENTED_EDGE ( 'NONE', *, *, #8854, .F. ) ;
#90718=CARTESIAN_POINT ( 'NONE',  ( 4.102725850843912170, 28.55253618238879909, -10.00000000000000000 ) ) ;
#90725=ORIENTED_EDGE ( 'NONE', *, *, #77029, .T. ) ;
#90728=ORIENTED_EDGE ( 'NONE', *, *, #92013, .F. ) ;
#90732=EDGE_CURVE ( 'NONE', #58893, #49038, #14312, .T. ) ;
#90739=CARTESIAN_POINT ( 'NONE',  ( -19.65312891409030271, 93.06504152958497400, 60.00000000000000000 ) ) ;
#90740=ORIENTED_EDGE ( 'NONE', *, *, #86739, .F. ) ;
#90745=ORIENTED_EDGE ( 'NONE', *, *, #77073, .F. ) ;
#90746=PLANE ( 'NONE',  #89068 ) ;
#90749=EDGE_CURVE ( 'NONE', #43182, #89564, #58291, .T. ) ;
#90759=LINE ( 'NONE', #21310, #96706 ) ;
#90760=EDGE_CURVE ( 'NONE', #22789, #48279, #18964, .T. ) ;
#90765=VERTEX_POINT ( 'NONE', #56795 ) ;
#90779=DIRECTION ( 'NONE',  ( 0.1548189829846108034, -0.9879428538673736826, 0.000000000000000000 ) ) ;
#90781=VECTOR ( 'NONE', #100012, 1000.000000000000114 ) ;
#90796=DIRECTION ( 'NONE',  ( 0.9738769792773321887, 0.2270762630343793331, 0.000000000000000000 ) ) ;
#90802=CARTESIAN_POINT ( 'NONE',  ( -19.65312891409030271, 93.06504152958497400, -10.00000000000000888 ) ) ;
#90811=CARTESIAN_POINT ( 'NONE',  ( -46.74660806181546491, 29.87360136034012825, -10.00000000000000000 ) ) ;
#90828=CARTESIAN_POINT ( 'NONE',  ( 38.13144443662678640, 88.76639304957403453, 59.99999999999999289 ) ) ;
#90829=EDGE_CURVE ( 'NONE', #22676, #24509, #98315, .T. ) ;
#90832=ORIENTED_EDGE ( 'NONE', *, *, #27080, .T. ) ;
#90836=ORIENTED_EDGE ( 'NONE', *, *, #6838, .T. ) ;
#90840=CARTESIAN_POINT ( 'NONE',  ( 13.43400709863221820, 31.08381733381234469, -10.00000000000000000 ) ) ;
#90851=VERTEX_POINT ( 'NONE', #83635 ) ;
#90853=DIRECTION ( 'NONE',  ( -0.7763215174174871169, 0.6303371332823493045, 0.000000000000000000 ) ) ;
#90854=LINE ( 'NONE', #6700, #48298 ) ;
#90855=ORIENTED_EDGE ( 'NONE', *, *, #68950, .T. ) ;
#90856=CIRCLE ( 'NONE', #60049, 49.99999999999999289 ) ;
#90858=EDGE_CURVE ( 'NONE', #41051, #31813, #61003, .T. ) ;
#90872=CARTESIAN_POINT ( 'NONE',  ( 47.83996289752659692, 111.6306699247848968, -10.00000000000000000 ) ) ;
#90879=EDGE_CURVE ( 'NONE', #74953, #65613, #62137, .T. ) ;
#90883=LINE ( 'NONE', #51840, #36933 ) ;
#90884=EDGE_LOOP ( 'NONE', ( #97826, #49923, #94740, #71710 ) ) ;
#90893=DIRECTION ( 'NONE',  ( -0.7071067811865474617, 8.659560562354932858E-17, 0.7071067811865474617 ) ) ;
#90897=CARTESIAN_POINT ( 'NONE',  ( 48.21858077004885246, 104.0489273421469818, -10.00000000000000000 ) ) ;
#90923=ORIENTED_EDGE ( 'NONE', *, *, #1126, .F. ) ;
#90941=CARTESIAN_POINT ( 'NONE',  ( -69.40242143070358338, 43.82067236826411261, -10.00000000000000000 ) ) ;
#90944=DIRECTION ( 'NONE',  ( -0.9515606131578174809, -0.3074612162317687525, 0.000000000000000000 ) ) ;
#90949=EDGE_CURVE ( 'NONE', #71153, #15777, #62638, .T. ) ;
#90954=ORIENTED_EDGE ( 'NONE', *, *, #91136, .T. ) ;
#90969=VERTEX_POINT ( 'NONE', #40340 ) ;
#90970=EDGE_LOOP ( 'NONE', ( #71960, #80120, #25819, #62109 ) ) ;
#90971=CARTESIAN_POINT ( 'NONE',  ( -19.65312891409030271, 93.06504152958497400, -10.00000000000000888 ) ) ;
#90976=EDGE_CURVE ( 'NONE', #38656, #11056, #71279, .T. ) ;
#90977=CARTESIAN_POINT ( 'NONE',  ( -0.4668637173180778532, 25.74574839753307387, -10.00000000000000000 ) ) ;
#90981=EDGE_LOOP ( 'NONE', ( #92334, #13428, #38187, #27012 ) ) ;
#90982=CARTESIAN_POINT ( 'NONE',  ( -76.49344163160107257, 52.20945622995200353, 177.5919119679930134 ) ) ;
#90996=DIRECTION ( 'NONE',  ( 0.000000000000000000, -0.000000000000000000, -1.000000000000000000 ) ) ;
#91001=DIRECTION ( 'NONE',  ( -1.000000000000000000, 0.000000000000000000, 0.000000000000000000 ) ) ;
#91003=LINE ( 'NONE', #59536, #76916 ) ;
#91011=LINE ( 'NONE', #98596, #25380 ) ;
#91013=CARTESIAN_POINT ( 'NONE',  ( -71.61465314115659453, 63.06504152958490295, 40.00000000000000000 ) ) ;
#91022=LINE ( 'NONE', #60059, #58191 ) ;
#91027=LINE ( 'NONE', #7886, #46741 ) ;
#91028=CARTESIAN_POINT ( 'NONE',  ( -19.79358564147677413, 93.04540364847184719, 59.99999999999999289 ) ) ;
#91033=LINE ( 'NONE', #74822, #59388 ) ;
#91034=DIRECTION ( 'NONE',  ( -0.000000000000000000, -0.000000000000000000, -1.000000000000000000 ) ) ;
#91038=LINE ( 'NONE', #21606, #56257 ) ;
#91047=LINE ( 'NONE', #74836, #75034 ) ;
#91059=EDGE_CURVE ( 'NONE', #59369, #52500, #86028, .T. ) ;
#91060=CARTESIAN_POINT ( 'NONE',  ( 48.83428215874787526, 87.09189275153327969, -10.00000000000000000 ) ) ;
#91064=VERTEX_POINT ( 'NONE', #56035 ) ;
#91065=LINE ( 'NONE', #66235, #4563 ) ;
#91067=EDGE_CURVE ( 'NONE', #1734, #65735, #57047, .T. ) ;
#91070=VERTEX_POINT ( 'NONE', #10982 ) ;
#91071=FACE_OUTER_BOUND ( 'NONE', #2602, .T. ) ;
#91080=VERTEX_POINT ( 'NONE', #41852 ) ;
#91081=ORIENTED_EDGE ( 'NONE', *, *, #64611, .F. ) ;
#91097=ORIENTED_EDGE ( 'NONE', *, *, #33747, .F. ) ;
#91100=VECTOR ( 'NONE', #44283, 1000.000000000000227 ) ;
#91106=ORIENTED_EDGE ( 'NONE', *, *, #69177, .T. ) ;
#91109=CARTESIAN_POINT ( 'NONE',  ( -17.26243516413818924, 24.35187462261283997, 10.00000000000000000 ) ) ;
#91110=ORIENTED_EDGE ( 'NONE', *, *, #45619, .T. ) ;
#91120=EDGE_LOOP ( 'NONE', ( #16142, #73615, #47642, #34479 ) ) ;
#91129=DIRECTION ( 'NONE',  ( -0.3374500364938434194, -0.9413434404457831084, 0.000000000000000000 ) ) ;
#91136=EDGE_CURVE ( 'NONE', #42726, #1733, #75267, .T. ) ;
#91139=DIRECTION ( 'NONE',  ( 0.000000000000000000, -0.000000000000000000, -1.000000000000000000 ) ) ;
#91154=PLANE ( 'NONE',  #85503 ) ;
#91162=VECTOR ( 'NONE', #99362, 1000.000000000000000 ) ;
#91163=DIRECTION ( 'NONE',  ( 0.9291732088853837945, -0.3696446237802449297, 0.000000000000000000 ) ) ;
#91167=EDGE_LOOP ( 'NONE', ( #40215, #29366, #4312, #28718 ) ) ;
#91168=AXIS2_PLACEMENT_3D ( 'NONE', #84931, #78813, #24090 ) ;
#91170=ORIENTED_EDGE ( 'NONE', *, *, #85328, .F. ) ;
#91174=CARTESIAN_POINT ( 'NONE',  ( -19.65312891409030271, 93.06504152958497400, 177.5919119679930134 ) ) ;
#91180=DIRECTION ( 'NONE',  ( -0.000000000000000000, -0.000000000000000000, 1.000000000000000000 ) ) ;
#91189=DIRECTION ( 'NONE',  ( -0.000000000000000000, -0.000000000000000000, -1.000000000000000000 ) ) ;
#91191=CARTESIAN_POINT ( 'NONE',  ( 47.96820964746023463, 80.67316705762479501, -10.00000000000000000 ) ) ;
#91193=VERTEX_POINT ( 'NONE', #5606 ) ;
#91195=CYLINDRICAL_SURFACE ( 'NONE', #5513, 70.00000000000002842 ) ;
#91208=ORIENTED_EDGE ( 'NONE', *, *, #99830, .F. ) ;
#91214=DIRECTION ( 'NONE',  ( -0.000000000000000000, 0.000000000000000000, -1.000000000000000000 ) ) ;
#91230=VERTEX_POINT ( 'NONE', #98826 ) ;
#91245=ADVANCED_FACE ( 'NONE', ( #68393 ), #28917, .F. ) ;
#91247=AXIS2_PLACEMENT_3D ( 'NONE', #98533, #6310, #92442 ) ;
#91262=LINE ( 'NONE', #66436, #43422 ) ;
#91263=VERTEX_POINT ( 'NONE', #74537 ) ;
#91272=CARTESIAN_POINT ( 'NONE',  ( 24.35067441160642687, 40.23626134430272572, -10.00000000000000000 ) ) ;
#91285=DIRECTION ( 'NONE',  ( 0.9999986627203610867, -0.001635407438361276495, 0.000000000000000000 ) ) ;
#91290=CARTESIAN_POINT ( 'NONE',  ( -63.30067564770008914, 39.94154026010144065, 10.00000000000000000 ) ) ;
#91291=SHAPE_DEFINITION_REPRESENTATION ( #71797, #78010 ) ;
#91295=ADVANCED_FACE ( 'NONE', ( #62784 ), #31879, .F. ) ;
#91297=ORIENTED_EDGE ( 'NONE', *, *, #18196, .T. ) ;
#91299=LINE ( 'NONE', #69456, #89131 ) ;
#91304=ORIENTED_EDGE ( 'NONE', *, *, #3947, .F. ) ;
#91305=CARTESIAN_POINT ( 'NONE',  ( 45.05588048050944394, 66.36777381976860113, 10.00000000000000000 ) ) ;
#91307=DIRECTION ( 'NONE',  ( -1.000000000000000000, 0.000000000000000000, 0.000000000000000000 ) ) ;
#91311=DIRECTION ( 'NONE',  ( 1.000000000000000000, 0.000000000000000000, 0.000000000000000000 ) ) ;
#91318=VERTEX_POINT ( 'NONE', #498 ) ;
#91319=DIRECTION ( 'NONE',  ( -0.9762143704923794685, 0.2168075248790210796, 0.000000000000000000 ) ) ;
#91324=DIRECTION ( 'NONE',  ( 0.000000000000000000, 0.000000000000000000, 1.000000000000000000 ) ) ;
#91329=CARTESIAN_POINT ( 'NONE',  ( -15.83597077268904663, 73.66574995701986950, 13.56964096002992015 ) ) ;
#91330=DIRECTION ( 'NONE',  ( -0.5607300124661884766, 0.8279987035736640077, 0.000000000000000000 ) ) ;
#91333=VERTEX_POINT ( 'NONE', #16196 ) ;
#91346=CARTESIAN_POINT ( 'NONE',  ( 48.60927726968589013, 109.6985806698937012, 10.00000000000000000 ) ) ;
#91347=DIRECTION ( 'NONE',  ( 0.000000000000000000, 0.000000000000000000, 1.000000000000000000 ) ) ;
#91366=DIRECTION ( 'NONE',  ( 0.000000000000000000, 0.000000000000000000, 1.000000000000000000 ) ) ;
#91370=LINE ( 'NONE', #83272, #34916 ) ;
#91376=EDGE_CURVE ( 'NONE', #43419, #68946, #39465, .T. ) ;
#91379=VECTOR ( 'NONE', #67510, 1000.000000000000114 ) ;
#91384=ORIENTED_EDGE ( 'NONE', *, *, #78225, .T. ) ;
#91400=ORIENTED_EDGE ( 'NONE', *, *, #1027, .F. ) ;
#91410=DIRECTION ( 'NONE',  ( -0.5888918169447132644, 0.8082118706970062849, 0.000000000000000000 ) ) ;
#91421=VECTOR ( 'NONE', #7791, 1000.000000000000227 ) ;
#91422=CARTESIAN_POINT ( 'NONE',  ( -33.12036098009136964, 24.37273002035945169, 10.00000000000000000 ) ) ;
#91423=EDGE_CURVE ( 'NONE', #16754, #20462, #73407, .T. ) ;
#91424=EDGE_CURVE ( 'NONE', #69834, #83731, #79546, .T. ) ;
#91425=DIRECTION ( 'NONE',  ( 0.000000000000000000, -0.000000000000000000, -1.000000000000000000 ) ) ;
#91432=DIRECTION ( 'NONE',  ( -0.000000000000000000, -0.000000000000000000, -1.000000000000000000 ) ) ;
#91437=FACE_OUTER_BOUND ( 'NONE', #7817, .T. ) ;
#91438=CARTESIAN_POINT ( 'NONE',  ( 1.813001633210440611, 27.74720351945397923, -10.00000000000000000 ) ) ;
#91445=ORIENTED_EDGE ( 'NONE', *, *, #46602, .F. ) ;
#91456=LINE ( 'NONE', #31595, #41152 ) ;
#91460=ADVANCED_FACE ( 'NONE', ( #34880 ), #88658, .T. ) ;
#91463=EDGE_LOOP ( 'NONE', ( #97176, #74483, #26091, #49314 ) ) ;
#91472=CARTESIAN_POINT ( 'NONE',  ( 17.60357497223980516, 35.28838536716092023, -10.00000000000000000 ) ) ;
#91474=CARTESIAN_POINT ( 'NONE',  ( 48.61286661847091750, 84.94359857078811160, -10.00000000000000000 ) ) ;
#91478=ORIENTED_EDGE ( 'NONE', *, *, #72142, .F. ) ;
#91481=CARTESIAN_POINT ( 'NONE',  ( -5.227692231867530737, 63.12463727082348441, -10.00000000000000000 ) ) ;
#91483=EDGE_CURVE ( 'NONE', #5025, #5362, #65779, .T. ) ;
#91493=ORIENTED_EDGE ( 'NONE', *, *, #22519, .T. ) ;
#91500=EDGE_CURVE ( 'NONE', #19199, #38977, #30285, .T. ) ;
#91504=CARTESIAN_POINT ( 'NONE',  ( -48.36978223816941380, 29.22654356899180428, 10.00000000000000000 ) ) ;
#91519=AXIS2_PLACEMENT_3D ( 'NONE', #13834, #20965, #37124 ) ;
#91520=LINE ( 'NONE', #13020, #46447 ) ;
#91526=AXIS2_PLACEMENT_3D ( 'NONE', #62569, #30702, #70688 ) ;
#91528=CARTESIAN_POINT ( 'NONE',  ( 45.57373283677818421, 114.7827874512443032, -10.00000000000000000 ) ) ;
#91529=CARTESIAN_POINT ( 'NONE',  ( -46.36014901014638667, 73.28484668120856327, -10.00000000000000000 ) ) ;
#91537=VERTEX_POINT ( 'NONE', #31270 ) ;
#91549=ORIENTED_EDGE ( 'NONE', *, *, #12523, .T. ) ;
#91554=VERTEX_POINT ( 'NONE', #62661 ) ;
#91565=VECTOR ( 'NONE', #3875, 1000.000000000000000 ) ;
#91572=CARTESIAN_POINT ( 'NONE',  ( -16.22246322593621315, 60.00824852743482296, -10.00000000000000000 ) ) ;
#91581=PLANE ( 'NONE',  #30208 ) ;
#91586=AXIS2_PLACEMENT_3D ( 'NONE', #68531, #30030, #60915 ) ;
#91587=VECTOR ( 'NONE', #56075, 1000.000000000000114 ) ;
#91592=DIRECTION ( 'NONE',  ( -0.9922852870422786964, 0.1239754375649568807, 0.000000000000000000 ) ) ;
#91594=VECTOR ( 'NONE', #42001, 1000.000000000000114 ) ;
#91616=EDGE_CURVE ( 'NONE', #65525, #29175, #61168, .T. ) ;
#91625=CARTESIAN_POINT ( 'NONE',  ( -23.73952538801239598, 24.43184193311134678, -10.00000000000000000 ) ) ;
#91628=CIRCLE ( 'NONE', #47903, 70.00000000000001421 ) ;
#91631=VECTOR ( 'NONE', #31008, 1000.000000000000000 ) ;
#91671=EDGE_CURVE ( 'NONE', #3615, #64281, #72408, .T. ) ;
#91679=EDGE_LOOP ( 'NONE', ( #55379, #67329, #10326, #97206 ) ) ;
#91682=CARTESIAN_POINT ( 'NONE',  ( 43.24043327773039636, 120.8247932685368227, 10.00000000000000000 ) ) ;
#91684=CARTESIAN_POINT ( 'NONE',  ( -66.34925969370661392, 42.61035540433362456, -10.00000000000000000 ) ) ;
#91687=VERTEX_POINT ( 'NONE', #54056 ) ;
#91700=ORIENTED_EDGE ( 'NONE', *, *, #34851, .F. ) ;
#91704=VECTOR ( 'NONE', #89069, 1000.000000000000000 ) ;
#91706=FACE_OUTER_BOUND ( 'NONE', #12405, .T. ) ;
#91707=ORIENTED_EDGE ( 'NONE', *, *, #48028, .F. ) ;
#91709=FACE_BOUND ( 'NONE', #62371, .T. ) ;
#91719=VERTEX_POINT ( 'NONE', #85013 ) ;
#91720=DIRECTION ( 'NONE',  ( -0.7300871660154473197, -0.6833540297821713017, 0.000000000000000000 ) ) ;
#91721=VERTEX_POINT ( 'NONE', #15557 ) ;
#91727=CARTESIAN_POINT ( 'NONE',  ( -19.65312891409030271, 93.06504152958497400, 59.99999999999999289 ) ) ;
#91737=LINE ( 'NONE', #30398, #6563 ) ;
#91738=VERTEX_POINT ( 'NONE', #16076 ) ;
#91740=CARTESIAN_POINT ( 'NONE',  ( 46.99867368304094839, 76.19044720721625197, -10.00000000000000000 ) ) ;
#91741=FACE_OUTER_BOUND ( 'NONE', #86471, .T. ) ;
#91749=CARTESIAN_POINT ( 'NONE',  ( 45.98627256186106393, 118.1229683434676900, -10.00000000000000000 ) ) ;
#91753=DIRECTION ( 'NONE',  ( -0.000000000000000000, -0.000000000000000000, 1.000000000000000000 ) ) ;
#91756=LINE ( 'NONE', #14720, #31735 ) ;
#91758=CARTESIAN_POINT ( 'NONE',  ( -13.90296923609177959, 23.04100004375993649, -10.00000000000000000 ) ) ;
#91759=ORIENTED_EDGE ( 'NONE', *, *, #11030, .T. ) ;
#91784=CARTESIAN_POINT ( 'NONE',  ( -19.65312891409030271, 93.06504152958497400, -10.00000000000000888 ) ) ;
#91795=ORIENTED_EDGE ( 'NONE', *, *, #10271, .F. ) ;
#91802=EDGE_CURVE ( 'NONE', #52500, #25226, #61646, .T. ) ;
#91814=ORIENTED_EDGE ( 'NONE', *, *, #35525, .T. ) ;
#91819=ORIENTED_EDGE ( 'NONE', *, *, #30539, .F. ) ;
#91823=ORIENTED_EDGE ( 'NONE', *, *, #9513, .T. ) ;
#91825=DIRECTION ( 'NONE',  ( -1.000000000000000000, 0.000000000000000000, 0.000000000000000000 ) ) ;
#91826=EDGE_LOOP ( 'NONE', ( #83891, #21797, #76468, #92261, #82873, #3829, #65618, #39229, #55502, #63807, #4063, #28257, #90477, #98537, #35814, #4328, #97937, #73242, #701, #31098, #64519, #60720, #50681, #36173, #81716, #32831, #22030, #45570, #29925, #40315, #80065, #27817, #70526, #70698, #97476, #69423, #72543, #23355, #34821, #90185, #84630, #8320, #40309, #25518 ) ) ;
#91830=CARTESIAN_POINT ( 'NONE',  ( -17.01447213259276126, 75.00420231477963284, 13.39782861781775480 ) ) ;
#91833=PLANE ( 'NONE',  #6201 ) ;
#91839=CARTESIAN_POINT ( 'NONE',  ( 50.33970617970973649, 92.06352491358971690, -10.00000000000000000 ) ) ;
#91852=DIRECTION ( 'NONE',  ( -0.9606745773021526658, 0.2776767122488494333, 0.000000000000000000 ) ) ;
#91858=EDGE_CURVE ( 'NONE', #24595, #78857, #39955, .T. ) ;
#91868=EDGE_CURVE ( 'NONE', #23610, #26987, #40832, .T. ) ;
#91876=AXIS2_PLACEMENT_3D ( 'NONE', #14039, #24995, #99147 ) ;
#91886=ADVANCED_FACE ( 'NONE', ( #18070 ), #2886, .F. ) ;
#91887=LINE ( 'NONE', #62414, #64338 ) ;
#91892=VECTOR ( 'NONE', #24554, 1000.000000000000000 ) ;
#91913=AXIS2_PLACEMENT_3D ( 'NONE', #20099, #3889, #12498 ) ;
#91919=CARTESIAN_POINT ( 'NONE',  ( -76.23101443460923576, 54.01191295053621388, -10.00000000000000000 ) ) ;
#91921=CARTESIAN_POINT ( 'NONE',  ( -63.30067564770008914, 39.94154026010144065, -10.00000000000000000 ) ) ;
#91924=DIRECTION ( 'NONE',  ( 0.000000000000000000, 0.000000000000000000, 1.000000000000000000 ) ) ;
#91925=CIRCLE ( 'NONE', #48206, 70.00000000000001421 ) ;
#91932=VECTOR ( 'NONE', #34723, 1000.000000000000114 ) ;
#91935=EDGE_CURVE ( 'NONE', #65525, #72951, #62588, .T. ) ;
#91936=DIRECTION ( 'NONE',  ( -0.9839629614562445115, 0.1783728972749415165, 0.000000000000000000 ) ) ;
#91941=VECTOR ( 'NONE', #42010, 1000.000000000000000 ) ;
#91943=CARTESIAN_POINT ( 'NONE',  ( -19.65312891409030271, 93.06504152958497400, 177.5919119679930134 ) ) ;
#91946=ORIENTED_EDGE ( 'NONE', *, *, #83257, .F. ) ;
#91950=ORIENTED_EDGE ( 'NONE', *, *, #49755, .F. ) ;
#91953=FACE_OUTER_BOUND ( 'NONE', #18692, .T. ) ;
#91954=AXIS2_PLACEMENT_3D ( 'NONE', #48329, #54394, #9327 ) ;
#91964=ORIENTED_EDGE ( 'NONE', *, *, #23322, .F. ) ;
#91970=ORIENTED_EDGE ( 'NONE', *, *, #77413, .T. ) ;
#91985=ORIENTED_EDGE ( 'NONE', *, *, #40345, .F. ) ;
#91989=CARTESIAN_POINT ( 'NONE',  ( 48.21858077004885246, 104.0489273421469818, -10.00000000000000000 ) ) ;
#91993=VERTEX_POINT ( 'NONE', #13466 ) ;
#91998=DIRECTION ( 'NONE',  ( -0.04056776950001317328, 0.9991767892008870389, 0.000000000000000000 ) ) ;
#92001=VECTOR ( 'NONE', #11664, 1000.000000000000000 ) ;
#92012=VECTOR ( 'NONE', #61764, 1000.000000000000000 ) ;
#92013=EDGE_CURVE ( 'NONE', #4221, #81160, #78829, .T. ) ;
#92015=CARTESIAN_POINT ( 'NONE',  ( 49.74924850768366724, 83.93760989710260390, 177.5919119679930134 ) ) ;
#92018=LINE ( 'NONE', #76287, #63103 ) ;
#92020=VECTOR ( 'NONE', #182, 1000.000000000000114 ) ;
#92070=VECTOR ( 'NONE', #71166, 999.9999999999998863 ) ;
#92077=AXIS2_PLACEMENT_3D ( 'NONE', #96516, #43251, #27591 ) ;
#92083=VECTOR ( 'NONE', #27155, 1000.000000000000000 ) ;
#92084=AXIS2_PLACEMENT_3D ( 'NONE', #97175, #2972, #79980 ) ;
#92088=EDGE_CURVE ( 'NONE', #71618, #4371, #10161, .T. ) ;
#92092=ADVANCED_FACE ( 'NONE', ( #45811 ), #237, .F. ) ;
#92099=PLANE ( 'NONE',  #66968 ) ;
#92102=CARTESIAN_POINT ( 'NONE',  ( -24.92793671336084671, 23.00358903956173862, 10.00000000000000000 ) ) ;
#92112=ORIENTED_EDGE ( 'NONE', *, *, #30810, .T. ) ;
#92120=ORIENTED_EDGE ( 'NONE', *, *, #29455, .T. ) ;
#92123=DIRECTION ( 'NONE',  ( 0.7278481391575630788, -0.6857383512134002101, 0.000000000000000000 ) ) ;
#92127=DIRECTION ( 'NONE',  ( 0.000000000000000000, 0.000000000000000000, 1.000000000000000000 ) ) ;
#92132=VERTEX_POINT ( 'NONE', #91474 ) ;
#92137=PLANE ( 'NONE',  #64121 ) ;
#92144=AXIS2_PLACEMENT_3D ( 'NONE', #56855, #89206, #19753 ) ;
#92149=VECTOR ( 'NONE', #56397, 1000.000000000000000 ) ;
#92151=VECTOR ( 'NONE', #61040, 1000.000000000000000 ) ;
#92154=CARTESIAN_POINT ( 'NONE',  ( -19.65312891409030271, 93.06504152958497400, -10.00000000000000888 ) ) ;
#92180=DIRECTION ( 'NONE',  ( 0.000000000000000000, 0.000000000000000000, 1.000000000000000000 ) ) ;
#92184=VERTEX_POINT ( 'NONE', #44830 ) ;
#92189=CARTESIAN_POINT ( 'NONE',  ( 47.92671612011951510, 80.40884667711614497, 10.00000000000000000 ) ) ;
#92196=ORIENTED_EDGE ( 'NONE', *, *, #22653, .F. ) ;
#92200=ORIENTED_EDGE ( 'NONE', *, *, #11030, .F. ) ;
#92203=DIRECTION ( 'NONE',  ( 0.000000000000000000, 0.000000000000000000, 1.000000000000000000 ) ) ;
#92214=ADVANCED_FACE ( 'NONE', ( #99551 ), #60027, .F. ) ;
#92216=VECTOR ( 'NONE', #86011, 1000.000000000000000 ) ;
#92224=ORIENTED_EDGE ( 'NONE', *, *, #46771, .T. ) ;
#92225=CIRCLE ( 'NONE', #32287, 70.00000000000001421 ) ;
#92240=ORIENTED_EDGE ( 'NONE', *, *, #19225, .T. ) ;
#92243=CIRCLE ( 'NONE', #93826, 0.1418229129680828593 ) ;
#92250=DIRECTION ( 'NONE',  ( -0.000000000000000000, 0.000000000000000000, -1.000000000000000000 ) ) ;
#92258=PLANE ( 'NONE',  #41408 ) ;
#92261=ORIENTED_EDGE ( 'NONE', *, *, #46073, .F. ) ;
#92275=ORIENTED_EDGE ( 'NONE', *, *, #52362, .F. ) ;
#92284=CARTESIAN_POINT ( 'NONE',  ( 49.09245556086620610, 93.56363653685789927, -10.00000000000000000 ) ) ;
#92312=ADVANCED_FACE ( 'NONE', ( #46833 ), #72158, .F. ) ;
#92315=EDGE_CURVE ( 'NONE', #55159, #9356, #71651, .T. ) ;
#92316=ORIENTED_EDGE ( 'NONE', *, *, #2129, .F. ) ;
#92317=EDGE_LOOP ( 'NONE', ( #40759, #66959, #87701, #84355 ) ) ;
#92327=ADVANCED_FACE ( 'NONE', ( #77755 ), #39208, .F. ) ;
#92334=ORIENTED_EDGE ( 'NONE', *, *, #64053, .T. ) ;
#92336=CARTESIAN_POINT ( 'NONE',  ( 24.56850397818812226, 63.80763720866956845, 59.99999999999999289 ) ) ;
#92339=ORIENTED_EDGE ( 'NONE', *, *, #77199, .T. ) ;
#92340=CARTESIAN_POINT ( 'NONE',  ( -19.70352899468211660, 93.19760687392162879, 59.99999999999999289 ) ) ;
#92341=LINE ( 'NONE', #47680, #55747 ) ;
#92350=LINE ( 'NONE', #91346, #61193 ) ;
#92362=AXIS2_PLACEMENT_3D ( 'NONE', #10805, #79741, #32078 ) ;
#92378=LINE ( 'NONE', #31027, #65641 ) ;
#92390=ADVANCED_FACE ( 'NONE', ( #25025 ), #87426, .F. ) ;
#92397=CARTESIAN_POINT ( 'NONE',  ( -39.78121323716017343, 66.61922423961890161, -10.00000000000000000 ) ) ;
#92420=ORIENTED_EDGE ( 'NONE', *, *, #33722, .T. ) ;
#92422=DIRECTION ( 'NONE',  ( -1.000000000000000000, 0.000000000000000000, 0.000000000000000000 ) ) ;
#92424=EDGE_CURVE ( 'NONE', #77091, #100075, #1756, .T. ) ;
#92426=LINE ( 'NONE', #21501, #10147 ) ;
#92430=VECTOR ( 'NONE', #8398, 1000.000000000000000 ) ;
#92432=ORIENTED_EDGE ( 'NONE', *, *, #93892, .T. ) ;
#92434=CYLINDRICAL_SURFACE ( 'NONE', #28838, 70.00000000000002842 ) ;
#92441=EDGE_CURVE ( 'NONE', #11925, #50507, #48999, .T. ) ;
#92442=DIRECTION ( 'NONE',  ( -1.000000000000000000, 0.000000000000000000, 0.000000000000000000 ) ) ;
#92444=DIRECTION ( 'NONE',  ( 0.000000000000000000, 0.000000000000000000, 1.000000000000000000 ) ) ;
#92452=ORIENTED_EDGE ( 'NONE', *, *, #33636, .F. ) ;
#92458=ORIENTED_EDGE ( 'NONE', *, *, #77797, .F. ) ;
#92461=CARTESIAN_POINT ( 'NONE',  ( -71.61465314115659453, 63.06504152958490295, 60.00000000000000000 ) ) ;
#92464=DIRECTION ( 'NONE',  ( -0.8321961394790272637, 0.5544813661758195567, 0.000000000000000000 ) ) ;
#92466=FACE_OUTER_BOUND ( 'NONE', #4975, .T. ) ;
#92469=VERTEX_POINT ( 'NONE', #10350 ) ;
#92476=ORIENTED_EDGE ( 'NONE', *, *, #33121, .T. ) ;
#92479=LINE ( 'NONE', #62518, #80802 ) ;
#92484=DIRECTION ( 'NONE',  ( 1.000000000000000000, 0.000000000000000000, 0.000000000000000000 ) ) ;
#92487=EDGE_CURVE ( 'NONE', #35590, #22676, #85904, .T. ) ;
#92491=DIRECTION ( 'NONE',  ( -0.7957378174433876739, 0.6056412518070690698, 0.000000000000000000 ) ) ;
#92495=VECTOR ( 'NONE', #94292, 1000.000000000000114 ) ;
#92511=EDGE_CURVE ( 'NONE', #5086, #43088, #32122, .T. ) ;
#92518=ADVANCED_FACE ( 'NONE', ( #32634 ), #63531, .F. ) ;
#92519=ORIENTED_EDGE ( 'NONE', *, *, #96333, .F. ) ;
#92523=CARTESIAN_POINT ( 'NONE',  ( -52.33464467766007289, 32.58262665401804270, -10.00000000000000000 ) ) ;
#92536=CARTESIAN_POINT ( 'NONE',  ( -8.406493707509316238, 25.24382671950691304, 10.00000000000000000 ) ) ;
#92537=EDGE_LOOP ( 'NONE', ( #50271, #2967, #57121, #93880 ) ) ;
#92542=ADVANCED_FACE ( 'NONE', ( #88909 ), #18958, .F. ) ;
#92543=VERTEX_POINT ( 'NONE', #80794 ) ;
#92547=FACE_OUTER_BOUND ( 'NONE', #94334, .T. ) ;
#92554=VERTEX_POINT ( 'NONE', #5235 ) ;
#92556=LINE ( 'NONE', #317, #67738 ) ;
#92557=EDGE_CURVE ( 'NONE', #73949, #48810, #57928, .T. ) ;
#92558=ORIENTED_EDGE ( 'NONE', *, *, #60442, .F. ) ;
#92565=EDGE_CURVE ( 'NONE', #53210, #20188, #81770, .T. ) ;
#92568=EDGE_CURVE ( 'NONE', #75209, #34863, #95898, .T. ) ;
#92569=DIRECTION ( 'NONE',  ( 0.000000000000000000, 0.000000000000000000, 1.000000000000000000 ) ) ;
#92577=CARTESIAN_POINT ( 'NONE',  ( 0.005075371086064872639, 27.18819441265828019, 10.00000000000000000 ) ) ;
#92581=CARTESIAN_POINT ( 'NONE',  ( 15.77038241084232517, 34.14663330942826747, -10.00000000000000000 ) ) ;
#92584=DIRECTION ( 'NONE',  ( -1.000000000000000000, 0.000000000000000000, 0.000000000000000000 ) ) ;
#92589=ORIENTED_EDGE ( 'NONE', *, *, #22519, .F. ) ;
#92599=ORIENTED_EDGE ( 'NONE', *, *, #11465, .F. ) ;
#92613=ORIENTED_EDGE ( 'NONE', *, *, #45378, .F. ) ;
#92621=CARTESIAN_POINT ( 'NONE',  ( 39.64431452495993824, 58.26521502737223557, -10.00000000000000000 ) ) ;
#92625=LINE ( 'NONE', #390, #67042 ) ;
#92628=EDGE_CURVE ( 'NONE', #91687, #48146, #81279, .T. ) ;
#92641=EDGE_CURVE ( 'NONE', #6854, #84457, #50328, .T. ) ;
#92648=CARTESIAN_POINT ( 'NONE',  ( 38.04107491472451841, 53.42442038713603125, 177.5919119679930134 ) ) ;
#92652=LINE ( 'NONE', #13630, #13495 ) ;
#92666=CARTESIAN_POINT ( 'NONE',  ( 41.10245927640360719, 127.8322459559854138, 177.5919119679930134 ) ) ;
#92671=ORIENTED_EDGE ( 'NONE', *, *, #73547, .F. ) ;
#92672=ORIENTED_EDGE ( 'NONE', *, *, #15139, .T. ) ;
#92677=CIRCLE ( 'NONE', #52205, 70.00000000000001421 ) ;
#92681=DIRECTION ( 'NONE',  ( -1.000000000000000000, 0.000000000000000000, 0.000000000000000000 ) ) ;
#92683=EDGE_CURVE ( 'NONE', #76358, #56880, #75633, .T. ) ;
#92688=ORIENTED_EDGE ( 'NONE', *, *, #21816, .F. ) ;
#92689=FACE_OUTER_BOUND ( 'NONE', #19475, .T. ) ;
#92698=VECTOR ( 'NONE', #70117, 1000.000000000000000 ) ;
#92703=CARTESIAN_POINT ( 'NONE',  ( -72.30469571560091424, 48.86078274006646183, 10.00000000000000000 ) ) ;
#92707=ORIENTED_EDGE ( 'NONE', *, *, #21595, .T. ) ;
#92711=DIRECTION ( 'NONE',  ( -0.5169068966820336009, 0.8560416229147678191, 0.000000000000000000 ) ) ;
#92715=ORIENTED_EDGE ( 'NONE', *, *, #17964, .F. ) ;
#92719=VERTEX_POINT ( 'NONE', #14324 ) ;
#92720=EDGE_CURVE ( 'NONE', #21922, #48026, #45211, .T. ) ;
#92732=DIRECTION ( 'NONE',  ( 1.000000000000000000, 0.000000000000000000, 0.000000000000000000 ) ) ;
#92733=ORIENTED_EDGE ( 'NONE', *, *, #29323, .T. ) ;
#92743=DIRECTION ( 'NONE',  ( -0.6544109481086124447, -0.7561390817803210762, 0.000000000000000000 ) ) ;
#92746=AXIS2_PLACEMENT_3D ( 'NONE', #8766, #10776, #54857 ) ;
#92747=ADVANCED_FACE ( 'NONE', ( #31501 ), #15806, .F. ) ;
#92751=CARTESIAN_POINT ( 'NONE',  ( 15.54467260552930341, 34.00295985972733348, -10.00000000000000000 ) ) ;
#92756=EDGE_LOOP ( 'NONE', ( #81406, #39119, #62039, #22529 ) ) ;
#92762=CARTESIAN_POINT ( 'NONE',  ( -19.65312891409030271, 93.06504152958497400, -25.00000000000000000 ) ) ;
#92793=DIRECTION ( 'NONE',  ( -0.5280678506503699854, -0.8492021815265776707, 0.000000000000000000 ) ) ;
#92802=CARTESIAN_POINT ( 'NONE',  ( -32.04500338604974985, 25.44370296803430520, 10.00000000000000000 ) ) ;
#92806=PLANE ( 'NONE',  #85276 ) ;
#92818=CARTESIAN_POINT ( 'NONE',  ( -16.99542894172669705, 24.36904009834037765, -10.00000000000000000 ) ) ;
#92819=LINE ( 'NONE', #46162, #72535 ) ;
#92820=EDGE_LOOP ( 'NONE', ( #68754, #41438, #63374, #33604 ) ) ;
#92821=CARTESIAN_POINT ( 'NONE',  ( -16.31071837694740623, 74.13583127143270701, 13.48478556928571948 ) ) ;
#92825=LINE ( 'NONE', #23378, #38231 ) ;
#92830=VECTOR ( 'NONE', #14967, 1000.000000000000000 ) ;
#92836=DIRECTION ( 'NONE',  ( 0.000000000000000000, 0.000000000000000000, 1.000000000000000000 ) ) ;
#92839=CARTESIAN_POINT ( 'NONE',  ( 20.94669640352213236, 37.57748520232517109, -10.00000000000000000 ) ) ;
#92845=ORIENTED_EDGE ( 'NONE', *, *, #24098, .F. ) ;
#92848=DIRECTION ( 'NONE',  ( 0.5637708215276955315, -0.8259312688075124420, 0.000000000000000000 ) ) ;
#92861=LINE ( 'NONE', #33026, #77354 ) ;
#92867=ADVANCED_FACE ( 'NONE', ( #50211 ), #4108, .T. ) ;
#92868=CARTESIAN_POINT ( 'NONE',  ( -6.542761065016642341, 25.57183462804972507, 10.00000000000000000 ) ) ;
#92872=EDGE_CURVE ( 'NONE', #4561, #54647, #57801, .T. ) ;
#92875=EDGE_CURVE ( 'NONE', #67111, #98668, #89474, .T. ) ;
#92877=ORIENTED_EDGE ( 'NONE', *, *, #70534, .T. ) ;
#92878=EDGE_CURVE ( 'NONE', #19564, #38181, #35002, .T. ) ;
#92892=ORIENTED_EDGE ( 'NONE', *, *, #38725, .F. ) ;
#92902=CARTESIAN_POINT ( 'NONE',  ( 48.61286661847091040, 84.94359857078811160, 10.00000000000000000 ) ) ;
#92904=VERTEX_POINT ( 'NONE', #57307 ) ;
#92919=ORIENTED_EDGE ( 'NONE', *, *, #47722, .T. ) ;
#92926=DIRECTION ( 'NONE',  ( -0.000000000000000000, -0.000000000000000000, -1.000000000000000000 ) ) ;
#92932=ORIENTED_EDGE ( 'NONE', *, *, #22663, .T. ) ;
#92934=CARTESIAN_POINT ( 'NONE',  ( 49.10122569834316408, 93.29622288527660601, -10.00000000000000000 ) ) ;
#92936=ORIENTED_EDGE ( 'NONE', *, *, #20140, .T. ) ;
#92937=ORIENTED_EDGE ( 'NONE', *, *, #40732, .F. ) ;
#92940=ORIENTED_EDGE ( 'NONE', *, *, #92487, .T. ) ;
#92942=ORIENTED_EDGE ( 'NONE', *, *, #78554, .F. ) ;
#92949=CARTESIAN_POINT ( 'NONE',  ( -68.29659580619643577, 42.72804590294295224, 10.00000000000000000 ) ) ;
#92951=CARTESIAN_POINT ( 'NONE',  ( -10.80656490723494123, 24.88181024604956804, -10.00000000000000000 ) ) ;
#92956=ORIENTED_EDGE ( 'NONE', *, *, #78877, .F. ) ;
#92980=ORIENTED_EDGE ( 'NONE', *, *, #48161, .T. ) ;
#92992=EDGE_LOOP ( 'NONE', ( #95081, #35981, #84646, #58693 ) ) ;
#92995=CARTESIAN_POINT ( 'NONE',  ( -15.10528209597770299, 24.46087392797018722, -10.00000000000000000 ) ) ;
#93020=PLANE ( 'NONE',  #91168 ) ;
#93022=PLANE ( 'NONE',  #79908 ) ;
#93031=FACE_OUTER_BOUND ( 'NONE', #80021, .T. ) ;
#93034=DIRECTION ( 'NONE',  ( -0.000000000000000000, -0.000000000000000000, 1.000000000000000000 ) ) ;
#93038=VERTEX_POINT ( 'NONE', #43519 ) ;
#93041=VECTOR ( 'NONE', #20626, 1000.000000000000227 ) ;
#93042=EDGE_LOOP ( 'NONE', ( #29230, #38555, #85789, #10089 ) ) ;
#93044=LINE ( 'NONE', #22125, #65322 ) ;
#93045=CARTESIAN_POINT ( 'NONE',  ( -19.65312891409030271, 93.06504152958497400, 59.99999999999999289 ) ) ;
#93047=EDGE_CURVE ( 'NONE', #91263, #11929, #51116, .T. ) ;
#93050=CARTESIAN_POINT ( 'NONE',  ( 16.62988887134222438, 56.19058022948441788, 59.99999999999999289 ) ) ;
#93051=EDGE_CURVE ( 'NONE', #29881, #38656, #35426, .T. ) ;
#93052=VERTEX_POINT ( 'NONE', #19749 ) ;
#93080=DIRECTION ( 'NONE',  ( -0.9303772761487891785, -0.3666034970181814012, 0.000000000000000000 ) ) ;
#93081=EDGE_CURVE ( 'NONE', #55233, #60043, #50614, .T. ) ;
#93088=ORIENTED_EDGE ( 'NONE', *, *, #5832, .T. ) ;
#93092=LINE ( 'NONE', #24662, #52686 ) ;
#93097=ORIENTED_EDGE ( 'NONE', *, *, #81227, .F. ) ;
#93102=CARTESIAN_POINT ( 'NONE',  ( -59.29375005653867703, 35.37083770076973366, -10.00000000000000000 ) ) ;
#93104=EDGE_CURVE ( 'NONE', #30963, #90765, #73939, .T. ) ;
#93106=AXIS2_PLACEMENT_3D ( 'NONE', #75602, #98909, #91825 ) ;
#93108=PLANE ( 'NONE',  #9012 ) ;
#93117=DIRECTION ( 'NONE',  ( 0.6303371332823493045, 0.7763215174174871169, 0.000000000000000000 ) ) ;
#93127=EDGE_CURVE ( 'NONE', #36969, #79746, #37901, .T. ) ;
#93142=VECTOR ( 'NONE', #28283, 1000.000000000000000 ) ;
#93149=CARTESIAN_POINT ( 'NONE',  ( 43.54657591670569872, 62.36930841191391295, 10.00000000000000000 ) ) ;
#93176=CARTESIAN_POINT ( 'NONE',  ( -61.39381520214497101, 38.43978098112751951, 10.00000000000000000 ) ) ;
#93192=DIRECTION ( 'NONE',  ( 0.000000000000000000, 0.000000000000000000, 1.000000000000000000 ) ) ;
#93195=ORIENTED_EDGE ( 'NONE', *, *, #60113, .T. ) ;
#93197=CARTESIAN_POINT ( 'NONE',  ( -54.25663331465118233, 31.91744790946455979, 10.00000000000000000 ) ) ;
#93198=VERTEX_POINT ( 'NONE', #48532 ) ;
#93203=CARTESIAN_POINT ( 'NONE',  ( 47.03029105687463840, 114.3563895605556269, 177.5919119679930134 ) ) ;
#93204=EDGE_CURVE ( 'NONE', #47298, #14902, #19857, .T. ) ;
#93207=CARTESIAN_POINT ( 'NONE',  ( -66.55019942848203129, 42.78701949053055387, 10.00000000000000000 ) ) ;
#93208=LINE ( 'NONE', #54657, #41496 ) ;
#93209=ADVANCED_FACE ( 'NONE', ( #16123 ), #926, .F. ) ;
#93211=ORIENTED_EDGE ( 'NONE', *, *, #24012, .T. ) ;
#93213=DIRECTION ( 'NONE',  ( 1.000000000000000000, 0.000000000000000000, 0.000000000000000000 ) ) ;
#93214=DIRECTION ( 'NONE',  ( -0.9825427565607363078, 0.1860369090530953895, 0.000000000000000000 ) ) ;
#93219=CIRCLE ( 'NONE', #62425, 70.00000000000001421 ) ;
#93223=VERTEX_POINT ( 'NONE', #24714 ) ;
#93228=VECTOR ( 'NONE', #35009, 1000.000000000000000 ) ;
#93231=ORIENTED_EDGE ( 'NONE', *, *, #7828, .F. ) ;
#93234=DIRECTION ( 'NONE',  ( -0.000000000000000000, -0.000000000000000000, -1.000000000000000000 ) ) ;
#93241=EDGE_CURVE ( 'NONE', #40956, #52454, #15603, .T. ) ;
#93243=ADVANCED_FACE ( 'NONE', ( #32818 ), #86580, .F. ) ;
#93258=ORIENTED_EDGE ( 'NONE', *, *, #92315, .T. ) ;
#93260=CARTESIAN_POINT ( 'NONE',  ( 37.96661208706053969, 52.86061180733513964, -10.00000000000000000 ) ) ;
#93268=PLANE ( 'NONE',  #45686 ) ;
#93276=DIRECTION ( 'NONE',  ( 0.4803199113995043623, -0.8770933717188679202, 0.000000000000000000 ) ) ;
#93283=CARTESIAN_POINT ( 'NONE',  ( 44.95821123098110661, 116.5722627105190270, 10.00000000000000000 ) ) ;
#93287=VECTOR ( 'NONE', #78091, 1000.000000000000227 ) ;
#93296=CARTESIAN_POINT ( 'NONE',  ( -12.95261720355844126, 24.63757726406876003, -10.00000000000000000 ) ) ;
#93298=VECTOR ( 'NONE', #92464, 1000.000000000000114 ) ;
#93301=VERTEX_POINT ( 'NONE', #48011 ) ;
#93314=AXIS2_PLACEMENT_3D ( 'NONE', #90413, #18610, #1907 ) ;
#93316=VECTOR ( 'NONE', #10466, 1000.000000000000227 ) ;
#93324=CARTESIAN_POINT ( 'NONE',  ( 44.35815684012577265, 67.96982248125696913, -10.00000000000000000 ) ) ;
#93328=ORIENTED_EDGE ( 'NONE', *, *, #79163, .T. ) ;
#93329=EDGE_CURVE ( 'NONE', #27171, #23113, #80975, .T. ) ;
#93330=ORIENTED_EDGE ( 'NONE', *, *, #6391, .F. ) ;
#93337=CARTESIAN_POINT ( 'NONE',  ( 48.91227514082039107, 78.96591507484178862, -10.00000000000000000 ) ) ;
#93349=LINE ( 'NONE', #3021, #91631 ) ;
#93357=EDGE_CURVE ( 'NONE', #24937, #92554, #34448, .T. ) ;
#93366=AXIS2_PLACEMENT_3D ( 'NONE', #61754, #54141, #84123 ) ;
#93375=DIRECTION ( 'NONE',  ( 0.000000000000000000, 0.000000000000000000, 1.000000000000000000 ) ) ;
#93380=VECTOR ( 'NONE', #93590, 1000.000000000000000 ) ;
#93389=VECTOR ( 'NONE', #41198, 1000.000000000000000 ) ;
#93390=FACE_OUTER_BOUND ( 'NONE', #17042, .T. ) ;
#93391=CARTESIAN_POINT ( 'NONE',  ( 26.02075121854041839, 117.3566028095996643, 59.99999999999999289 ) ) ;
#93416=ORIENTED_EDGE ( 'NONE', *, *, #19468, .T. ) ;
#93427=DIRECTION ( 'NONE',  ( -0.000000000000000000, -0.000000000000000000, -1.000000000000000000 ) ) ;
#93430=ORIENTED_EDGE ( 'NONE', *, *, #22591, .T. ) ;
#93431=ORIENTED_EDGE ( 'NONE', *, *, #26811, .F. ) ;
#93432=CARTESIAN_POINT ( 'NONE',  ( 24.55112987542764458, 40.41347472807388641, -10.00000000000000000 ) ) ;
#93435=FACE_OUTER_BOUND ( 'NONE', #46837, .T. ) ;
#93438=CARTESIAN_POINT ( 'NONE',  ( 32.74483707338229266, 117.8038484974524351, 59.99999999999999289 ) ) ;
#93445=VECTOR ( 'NONE', #76827, 1000.000000000000114 ) ;
#93450=EDGE_CURVE ( 'NONE', #85874, #27025, #87602, .T. ) ;
#93453=EDGE_CURVE ( 'NONE', #100173, #35725, #18636, .T. ) ;
#93454=CARTESIAN_POINT ( 'NONE',  ( 42.25626477193290498, 60.39660150822810891, 10.00000000000000000 ) ) ;
#93457=VECTOR ( 'NONE', #33731, 1000.000000000000114 ) ;
#93462=EDGE_CURVE ( 'NONE', #50507, #16411, #43900, .T. ) ;
#93471=ORIENTED_EDGE ( 'NONE', *, *, #56926, .T. ) ;
#93475=DIRECTION ( 'NONE',  ( 0.000000000000000000, 0.000000000000000000, 1.000000000000000000 ) ) ;
#93489=CARTESIAN_POINT ( 'NONE',  ( 48.16808589598787904, 104.3116767361652535, 10.00000000000000000 ) ) ;
#93503=ORIENTED_EDGE ( 'NONE', *, *, #74823, .T. ) ;
#93510=AXIS2_PLACEMENT_3D ( 'NONE', #88495, #4326, #43312 ) ;
#93521=VECTOR ( 'NONE', #5020, 1000.000000000000000 ) ;
#93533=CARTESIAN_POINT ( 'NONE',  ( -19.65312891409030271, 93.06504152958497400, -10.00000000000000888 ) ) ;
#93534=DIRECTION ( 'NONE',  ( -0.9404163354663408469, -0.3400251696390412803, 0.000000000000000000 ) ) ;
#93537=ORIENTED_EDGE ( 'NONE', *, *, #18318, .T. ) ;
#93545=DIRECTION ( 'NONE',  ( -0.9042435392811322137, -0.4270171210482451296, 0.000000000000000000 ) ) ;
#93565=ORIENTED_EDGE ( 'NONE', *, *, #19237, .F. ) ;
#93574=VECTOR ( 'NONE', #97608, 1000.000000000000000 ) ;
#93575=CARTESIAN_POINT ( 'NONE',  ( -61.39381520214497101, 38.43978098112751951, -10.00000000000000000 ) ) ;
#93577=LINE ( 'NONE', #55029, #92216 ) ;
#93582=ORIENTED_EDGE ( 'NONE', *, *, #75984, .F. ) ;
#93585=CARTESIAN_POINT ( 'NONE',  ( -47.54945751754587491, 75.00082604429731248, -10.00000000000000000 ) ) ;
#93590=DIRECTION ( 'NONE',  ( 0.000000000000000000, 0.000000000000000000, 1.000000000000000000 ) ) ;
#93595=AXIS2_PLACEMENT_3D ( 'NONE', #32906, #89183, #96755 ) ;
#93601=CARTESIAN_POINT ( 'NONE',  ( -70.89022602266993545, 47.22876919346843749, 10.00000000000000000 ) ) ;
#93603=CARTESIAN_POINT ( 'NONE',  ( -70.92467617367974242, 45.40763453331954480, 177.5919119679930134 ) ) ;
#93607=ORIENTED_EDGE ( 'NONE', *, *, #27443, .F. ) ;
#93610=DIRECTION ( 'NONE',  ( -0.000000000000000000, -0.000000000000000000, -1.000000000000000000 ) ) ;
#93618=FACE_OUTER_BOUND ( 'NONE', #83112, .T. ) ;
#93619=AXIS2_PLACEMENT_3D ( 'NONE', #79183, #26938, #88801 ) ;
#93631=CARTESIAN_POINT ( 'NONE',  ( 23.64814127513154673, 118.0650415295851019, 20.00000000000000355 ) ) ;
#93637=CARTESIAN_POINT ( 'NONE',  ( -73.83803415018344651, 50.74234351129840093, -10.00000000000000000 ) ) ;
#93638=EDGE_CURVE ( 'NONE', #44012, #16902, #95975, .T. ) ;
#93642=CIRCLE ( 'NONE', #20812, 60.00000000000002132 ) ;
#93650=DIRECTION ( 'NONE',  ( -0.000000000000000000, 0.000000000000000000, 1.000000000000000000 ) ) ;
#93651=VECTOR ( 'NONE', #92836, 1000.000000000000000 ) ;
#93660=VECTOR ( 'NONE', #96820, 999.9999999999998863 ) ;
#93663=LINE ( 'NONE', #24227, #88241 ) ;
#93667=CARTESIAN_POINT ( 'NONE',  ( -0.1936345643149539608, 38.48607693945955077, 59.99999999999999289 ) ) ;
#93676=EDGE_LOOP ( 'NONE', ( #2756, #76640, #7274, #49666 ) ) ;
#93679=DIRECTION ( 'NONE',  ( 0.000000000000000000, -0.000000000000000000, -1.000000000000000000 ) ) ;
#93683=VERTEX_POINT ( 'NONE', #18516 ) ;
#93686=CYLINDRICAL_SURFACE ( 'NONE', #66228, 70.00000000000002842 ) ;
#93689=ORIENTED_EDGE ( 'NONE', *, *, #43755, .F. ) ;
#93693=CARTESIAN_POINT ( 'NONE',  ( -19.65312891409030271, 93.06504152958497400, 177.5919119679930134 ) ) ;
#93701=EDGE_CURVE ( 'NONE', #79632, #96562, #86967, .T. ) ;
#93711=VERTEX_POINT ( 'NONE', #50889 ) ;
#93715=EDGE_CURVE ( 'NONE', #1197, #39666, #76213, .T. ) ;
#93723=ORIENTED_EDGE ( 'NONE', *, *, #13674, .F. ) ;
#93738=CARTESIAN_POINT ( 'NONE',  ( -26.53413439647355787, 34.79436034334068495, 59.99999999999999289 ) ) ;
#93745=VERTEX_POINT ( 'NONE', #6789 ) ;
#93746=CARTESIAN_POINT ( 'NONE',  ( 21.15788363470973366, 37.74176219324819215, 10.00000000000000000 ) ) ;
#93747=VECTOR ( 'NONE', #199, 1000.000000000000114 ) ;
#93755=VECTOR ( 'NONE', #52865, 1000.000000000000114 ) ;
#93756=EDGE_CURVE ( 'NONE', #10181, #97433, #4815, .T. ) ;
#93758=PLANE ( 'NONE',  #22448 ) ;
#93761=EDGE_CURVE ( 'NONE', #100075, #82380, #28092, .T. ) ;
#93780=DIRECTION ( 'NONE',  ( -0.5346708562974007428, -0.8450603975019799208, 0.000000000000000000 ) ) ;
#93792=CIRCLE ( 'NONE', #95407, 0.1418229129680863287 ) ;
#93804=FACE_OUTER_BOUND ( 'NONE', #42845, .T. ) ;
#93807=EDGE_CURVE ( 'NONE', #65437, #39666, #52385, .T. ) ;
#93808=VERTEX_POINT ( 'NONE', #91422 ) ;
#93813=ORIENTED_EDGE ( 'NONE', *, *, #68341, .T. ) ;
#93820=CYLINDRICAL_SURFACE ( 'NONE', #18953, 70.00000000000002842 ) ;
#93826=AXIS2_PLACEMENT_3D ( 'NONE', #63985, #41675, #72619 ) ;
#93828=ADVANCED_FACE ( 'NONE', ( #87231 ), #70969, .T. ) ;
#93832=ORIENTED_EDGE ( 'NONE', *, *, #4718, .T. ) ;
#93838=CIRCLE ( 'NONE', #26838, 0.1418229129680828593 ) ;
#93842=CARTESIAN_POINT ( 'NONE',  ( -9.517469918280088592, 23.54023200771947799, 10.00000000000000000 ) ) ;
#93863=LINE ( 'NONE', #94358, #59613 ) ;
#93866=VERTEX_POINT ( 'NONE', #32943 ) ;
#93873=CIRCLE ( 'NONE', #16161, 70.00000000000001421 ) ;
#93876=CARTESIAN_POINT ( 'NONE',  ( 32.29521950065672087, 67.39590844996666874, 59.99999999999999289 ) ) ;
#93880=ORIENTED_EDGE ( 'NONE', *, *, #49491, .T. ) ;
#93882=CARTESIAN_POINT ( 'NONE',  ( 43.83595887736691310, 122.5461495720015677, -10.00000000000000000 ) ) ;
#93886=DIRECTION ( 'NONE',  ( -0.000000000000000000, -0.000000000000000000, -1.000000000000000000 ) ) ;
#93887=AXIS2_PLACEMENT_3D ( 'NONE', #54187, #99827, #46596 ) ;
#93891=ORIENTED_EDGE ( 'NONE', *, *, #11228, .T. ) ;
#93892=EDGE_CURVE ( 'NONE', #38792, #29884, #1571, .T. ) ;
#93900=CARTESIAN_POINT ( 'NONE',  ( -46.49770490450612215, 29.77544742692501600, -10.00000000000000000 ) ) ;
#93902=LINE ( 'NONE', #48771, #64425 ) ;
#93917=LINE ( 'NONE', #39643, #61059 ) ;
#93925=DIRECTION ( 'NONE',  ( 0.2701803667135113662, 0.9628097264997651505, 0.000000000000000000 ) ) ;
#93931=DIRECTION ( 'NONE',  ( 0.000000000000000000, 0.000000000000000000, 1.000000000000000000 ) ) ;
#93938=CARTESIAN_POINT ( 'NONE',  ( 36.10619739613039769, 52.83927550304669296, -10.00000000000000000 ) ) ;
#93941=AXIS2_PLACEMENT_3D ( 'NONE', #41919, #18639, #72354 ) ;
#93951=ORIENTED_EDGE ( 'NONE', *, *, #27580, .T. ) ;
#93953=EDGE_LOOP ( 'NONE', ( #8060, #85995, #17678, #51726 ) ) ;
#93954=ORIENTED_EDGE ( 'NONE', *, *, #35773, .F. ) ;
#93965=CYLINDRICAL_SURFACE ( 'NONE', #77428, 70.00000000000002842 ) ;
#93969=CARTESIAN_POINT ( 'NONE',  ( -30.18034446749236821, 25.12100238203592539, -10.00000000000000000 ) ) ;
#93985=EDGE_CURVE ( 'NONE', #43160, #66403, #70087, .T. ) ;
#94007=VERTEX_POINT ( 'NONE', #34936 ) ;
#94019=EDGE_CURVE ( 'NONE', #58141, #54753, #66838, .T. ) ;
#94025=VECTOR ( 'NONE', #21385, 1000.000000000000000 ) ;
#94030=DIRECTION ( 'NONE',  ( 0.08498217737243619896, 0.9963824715083259287, 0.000000000000000000 ) ) ;
#94036=CARTESIAN_POINT ( 'NONE',  ( 2.064617007569734319, 27.83817977871672511, 10.00000000000000000 ) ) ;
#94055=ORIENTED_EDGE ( 'NONE', *, *, #75659, .T. ) ;
#94057=LINE ( 'NONE', #79369, #1436 ) ;
#94064=DIRECTION ( 'NONE',  ( -0.000000000000000000, -0.000000000000000000, 1.000000000000000000 ) ) ;
#94065=CARTESIAN_POINT ( 'NONE',  ( -19.65312891409030271, 93.06504152958497400, 177.5919119679930134 ) ) ;
#94067=CARTESIAN_POINT ( 'NONE',  ( 26.18314342202568668, 41.82794442100486521, 10.00000000000000000 ) ) ;
#94068=ORIENTED_EDGE ( 'NONE', *, *, #35795, .T. ) ;
#94069=EDGE_LOOP ( 'NONE', ( #26015, #19206, #92688, #30382 ) ) ;
#94071=VERTEX_POINT ( 'NONE', #14644 ) ;
#94073=ORIENTED_EDGE ( 'NONE', *, *, #46448, .T. ) ;
#94090=ORIENTED_EDGE ( 'NONE', *, *, #94473, .T. ) ;
#94098=DIRECTION ( 'NONE',  ( 1.000000000000000000, 0.000000000000000000, 0.000000000000000000 ) ) ;
#94106=EDGE_LOOP ( 'NONE', ( #14141, #55859, #67990, #70834 ) ) ;
#94111=DIRECTION ( 'NONE',  ( -0.6600842437418951159, 0.7511915808658203852, 0.000000000000000000 ) ) ;
#94132=LINE ( 'NONE', #54073, #27491 ) ;
#94138=EDGE_CURVE ( 'NONE', #63494, #47254, #40914, .T. ) ;
#94140=DIRECTION ( 'NONE',  ( 0.000000000000000000, 0.000000000000000000, 1.000000000000000000 ) ) ;
#94145=EDGE_CURVE ( 'NONE', #16902, #95220, #38926, .T. ) ;
#94163=AXIS2_PLACEMENT_3D ( 'NONE', #87223, #87721, #51007 ) ;
#94169=ORIENTED_EDGE ( 'NONE', *, *, #82570, .F. ) ;
#94182=DIRECTION ( 'NONE',  ( -0.9923183454821337124, -0.1237105541964824140, 0.000000000000000000 ) ) ;
#94189=ORIENTED_EDGE ( 'NONE', *, *, #37322, .F. ) ;
#94190=CARTESIAN_POINT ( 'NONE',  ( -32.10208857249643444, 42.85342256331377087, 59.99999999999999289 ) ) ;
#94207=EDGE_CURVE ( 'NONE', #83607, #72764, #70845, .T. ) ;
#94213=DIRECTION ( 'NONE',  ( 0.5609510170580086497, 0.8278489937552534483, 0.000000000000000000 ) ) ;
#94219=EDGE_CURVE ( 'NONE', #54945, #77851, #33340, .T. ) ;
#94221=DIRECTION ( 'NONE',  ( -0.6879669212057208938, -0.7257420446182799578, 0.000000000000000000 ) ) ;
#94222=AXIS2_PLACEMENT_3D ( 'NONE', #89317, #19872, #81694 ) ;
#94229=CARTESIAN_POINT ( 'NONE',  ( 45.16679497745494132, 120.1723871950187714, -10.00000000000000000 ) ) ;
#94230=ORIENTED_EDGE ( 'NONE', *, *, #37322, .T. ) ;
#94236=DIRECTION ( 'NONE',  ( 0.4737039832092607705, 0.8806841296921844586, 0.000000000000000000 ) ) ;
#94239=DIRECTION ( 'NONE',  ( -0.000000000000000000, -0.000000000000000000, -1.000000000000000000 ) ) ;
#94246=ORIENTED_EDGE ( 'NONE', *, *, #77543, .T. ) ;
#94253=EDGE_CURVE ( 'NONE', #9430, #25628, #442, .T. ) ;
#94261=ORIENTED_EDGE ( 'NONE', *, *, #64204, .F. ) ;
#94268=DIRECTION ( 'NONE',  ( 1.000000000000000000, 0.000000000000000000, 0.000000000000000000 ) ) ;
#94280=DIRECTION ( 'NONE',  ( 1.000000000000000000, 0.000000000000000000, 0.000000000000000000 ) ) ;
#94283=DIRECTION ( 'NONE',  ( 0.9171038997749326738, -0.3986482622784278118, 0.000000000000000000 ) ) ;
#94291=CARTESIAN_POINT ( 'NONE',  ( -19.15453390681661716, 24.31945705462846163, -10.00000000000000000 ) ) ;
#94292=DIRECTION ( 'NONE',  ( 0.9954067278227226589, -0.09573633691164461224, 0.000000000000000000 ) ) ;
#94310=ORIENTED_EDGE ( 'NONE', *, *, #7043, .F. ) ;
#94314=ORIENTED_EDGE ( 'NONE', *, *, #45141, .T. ) ;
#94315=CARTESIAN_POINT ( 'NONE',  ( 30.77278128771378007, 63.06390461086555632, 59.99999999999999289 ) ) ;
#94317=LINE ( 'NONE', #78596, #40241 ) ;
#94321=EDGE_CURVE ( 'NONE', #79865, #66165, #96181, .T. ) ;
#94323=LINE ( 'NONE', #69970, #44537 ) ;
#94328=EDGE_CURVE ( 'NONE', #37845, #23277, #10550, .T. ) ;
#94334=EDGE_LOOP ( 'NONE', ( #15257, #37599, #92432, #54027 ) ) ;
#94337=CARTESIAN_POINT ( 'NONE',  ( -52.57320609282758994, 32.70376883311632810, -10.00000000000000000 ) ) ;
#94338=ORIENTED_EDGE ( 'NONE', *, *, #64505, .T. ) ;
#94344=CARTESIAN_POINT ( 'NONE',  ( 21.20245638554209222, 36.22472881207375650, -10.00000000000000000 ) ) ;
#94352=ORIENTED_EDGE ( 'NONE', *, *, #85582, .T. ) ;
#94358=CARTESIAN_POINT ( 'NONE',  ( 19.39999966495784989, 36.48715600906564305, 10.00000000000000000 ) ) ;
#94361=ORIENTED_EDGE ( 'NONE', *, *, #37923, .F. ) ;
#94381=ADVANCED_FACE ( 'NONE', ( #91071 ), #52517, .F. ) ;
#94393=DIRECTION ( 'NONE',  ( 1.000000000000000000, 0.000000000000000000, 0.000000000000000000 ) ) ;
#94397=DIRECTION ( 'NONE',  ( -0.2270762630343793331, 0.9738769792773321887, 0.000000000000000000 ) ) ;
#94399=VERTEX_POINT ( 'NONE', #76344 ) ;
#94401=FACE_OUTER_BOUND ( 'NONE', #56804, .T. ) ;
#94405=CARTESIAN_POINT ( 'NONE',  ( 21.04740724657494866, 61.13308837878306434, 59.99999999999999289 ) ) ;
#94407=DIRECTION ( 'NONE',  ( 1.000000000000000000, 0.000000000000000000, 0.000000000000000000 ) ) ;
#94413=LINE ( 'NONE', #71598, #27754 ) ;
#94419=FACE_OUTER_BOUND ( 'NONE', #99395, .T. ) ;
#94421=AXIS2_PLACEMENT_3D ( 'NONE', #93667, #8531, #86586 ) ;
#94422=LINE ( 'NONE', #62458, #16643 ) ;
#94439=ORIENTED_EDGE ( 'NONE', *, *, #87652, .F. ) ;
#94453=VERTEX_POINT ( 'NONE', #67224 ) ;
#94467=ORIENTED_EDGE ( 'NONE', *, *, #66263, .F. ) ;
#94472=DIRECTION ( 'NONE',  ( -0.000000000000000000, -0.000000000000000000, 1.000000000000000000 ) ) ;
#94473=EDGE_CURVE ( 'NONE', #21753, #29279, #99185, .T. ) ;
#94476=ORIENTED_EDGE ( 'NONE', *, *, #10512, .F. ) ;
#94483=DIRECTION ( 'NONE',  ( 0.3666034970181715202, -0.9303772761487929532, 0.000000000000000000 ) ) ;
#94484=DIRECTION ( 'NONE',  ( 0.4245406647209822304, 0.9054088711727241723, 0.000000000000000000 ) ) ;
#94495=VECTOR ( 'NONE', #30746, 1000.000000000000000 ) ;
#94503=FACE_OUTER_BOUND ( 'NONE', #78962, .T. ) ;
#94504=ORIENTED_EDGE ( 'NONE', *, *, #74967, .F. ) ;
#94507=AXIS2_PLACEMENT_3D ( 'NONE', #18417, #41182, #95465 ) ;
#94509=DIRECTION ( 'NONE',  ( 0.000000000000000000, -0.000000000000000000, -1.000000000000000000 ) ) ;
#94521=EDGE_LOOP ( 'NONE', ( #66113, #64242, #89945, #19640 ) ) ;
#94526=CARTESIAN_POINT ( 'NONE',  ( -56.06787742410712383, 34.75406423768147590, -10.00000000000000000 ) ) ;
#94538=VERTEX_POINT ( 'NONE', #57507 ) ;
#94542=DIRECTION ( 'NONE',  ( 1.000000000000000000, 0.000000000000000000, 0.000000000000000000 ) ) ;
#94544=ORIENTED_EDGE ( 'NONE', *, *, #92088, .F. ) ;
#94548=ORIENTED_EDGE ( 'NONE', *, *, #95672, .T. ) ;
#94550=ADVANCED_FACE ( 'NONE', ( #26127 ), #58014, .F. ) ;
#94562=ORIENTED_EDGE ( 'NONE', *, *, #37703, .F. ) ;
#94566=VECTOR ( 'NONE', #79714, 999.9999999999998863 ) ;
#94567=VERTEX_POINT ( 'NONE', #19549 ) ;
#94570=ORIENTED_EDGE ( 'NONE', *, *, #5521, .T. ) ;
#94574=DIRECTION ( 'NONE',  ( -0.3105719460338542404, -0.9505498757754611283, 0.000000000000000000 ) ) ;
#94577=DIRECTION ( 'NONE',  ( 0.000000000000000000, 0.000000000000000000, 1.000000000000000000 ) ) ;
#94578=CIRCLE ( 'NONE', #3937, 0.1418229129683812317 ) ;
#94582=ORIENTED_EDGE ( 'NONE', *, *, #43684, .T. ) ;
#94587=DIRECTION ( 'NONE',  ( -0.8806841296921844586, 0.4737039832092607705, 0.000000000000000000 ) ) ;
#94588=LINE ( 'NONE', #24645, #23783 ) ;
#94589=CARTESIAN_POINT ( 'NONE',  ( 9.242171499132833645, 29.30720582267293040, 177.5919119679930134 ) ) ;
#94592=ADVANCED_FACE ( 'NONE', ( #37685 ), #89950, .F. ) ;
#94603=DIRECTION ( 'NONE',  ( 0.8965230319888196631, -0.4429971254010276471, 0.000000000000000000 ) ) ;
#94605=DIRECTION ( 'NONE',  ( 0.000000000000000000, 0.000000000000000000, 1.000000000000000000 ) ) ;
#94611=ORIENTED_EDGE ( 'NONE', *, *, #74365, .F. ) ;
#94618=DIRECTION ( 'NONE',  ( -0.000000000000000000, 0.000000000000000000, -1.000000000000000000 ) ) ;
#94635=FACE_OUTER_BOUND ( 'NONE', #71359, .T. ) ;
#94642=CARTESIAN_POINT ( 'NONE',  ( -36.26652983198114555, 26.35523046909639788, 10.00000000000000000 ) ) ;
#94645=AXIS2_PLACEMENT_3D ( 'NONE', #56844, #32558, #54844 ) ;
#94648=CARTESIAN_POINT ( 'NONE',  ( 49.28760614098965931, 105.1966139777580338, 177.5919119679930134 ) ) ;
#94669=ORIENTED_EDGE ( 'NONE', *, *, #58430, .F. ) ;
#94673=ORIENTED_EDGE ( 'NONE', *, *, #39516, .F. ) ;
#94678=CARTESIAN_POINT ( 'NONE',  ( 34.05451400132101014, 48.17084265633775431, -10.00000000000000000 ) ) ;
#94679=VERTEX_POINT ( 'NONE', #697 ) ;
#94680=VECTOR ( 'NONE', #12304, 1000.000000000000114 ) ;
#94700=DIRECTION ( 'NONE',  ( -0.3402761906661169178, -0.9403255362191098587, 0.000000000000000000 ) ) ;
#94701=CARTESIAN_POINT ( 'NONE',  ( -9.693023484072631035, 23.77726266618848072, -10.00000000000000000 ) ) ;
#94702=ORIENTED_EDGE ( 'NONE', *, *, #98341, .T. ) ;
#94709=ADVANCED_FACE ( 'NONE', ( #54370 ), #14890, .T. ) ;
#94712=VECTOR ( 'NONE', #8313, 1000.000000000000000 ) ;
#94717=EDGE_CURVE ( 'NONE', #39405, #28901, #7032, .T. ) ;
#94718=ORIENTED_EDGE ( 'NONE', *, *, #23190, .F. ) ;
#94719=ADVANCED_FACE ( 'NONE', ( #15376 ), #39667, .F. ) ;
#94720=AXIS2_PLACEMENT_3D ( 'NONE', #77300, #22096, #37783 ) ;
#94732=ORIENTED_EDGE ( 'NONE', *, *, #86488, .T. ) ;
#94740=ORIENTED_EDGE ( 'NONE', *, *, #23137, .F. ) ;
#94747=CARTESIAN_POINT ( 'NONE',  ( 37.96661208706053969, 52.86061180733513964, 10.00000000000000000 ) ) ;
#94749=CARTESIAN_POINT ( 'NONE',  ( -72.48190909937210336, 49.06123820388767598, -10.00000000000000000 ) ) ;
#94758=DIRECTION ( 'NONE',  ( 0.000000000000000000, 0.000000000000000000, 1.000000000000000000 ) ) ;
#94766=AXIS2_PLACEMENT_3D ( 'NONE', #14417, #92444, #84841 ) ;
#94769=LINE ( 'NONE', #26345, #52515 ) ;
#94783=LINE ( 'NONE', #24840, #69306 ) ;
#94788=CARTESIAN_POINT ( 'NONE',  ( -21.88991730065903596, 40.08839396453016235, 59.99999999999999289 ) ) ;
#94795=DIRECTION ( 'NONE',  ( 0.2500151307524129396, -0.9682419296822740717, 0.000000000000000000 ) ) ;
#94796=CARTESIAN_POINT ( 'NONE',  ( 18.75993726342624157, 49.68311261143426805, 59.99999999999999289 ) ) ;
#94802=CARTESIAN_POINT ( 'NONE',  ( -67.91103796225580425, 44.10201266000169795, 10.00000000000000000 ) ) ;
#94805=ORIENTED_EDGE ( 'NONE', *, *, #3423, .F. ) ;
#94812=CARTESIAN_POINT ( 'NONE',  ( -19.65312891409030271, 93.06504152958497400, 10.00000000000000888 ) ) ;
#94818=DIRECTION ( 'NONE',  ( -0.5544813661758285495, -0.8321961394790213795, 0.000000000000000000 ) ) ;
#94825=CARTESIAN_POINT ( 'NONE',  ( 23.99212445955422623, 54.95143152255312913, 59.99999999999999289 ) ) ;
#94828=CARTESIAN_POINT ( 'NONE',  ( -54.25663331465118233, 31.91744790946455979, -10.00000000000000000 ) ) ;
#94834=ORIENTED_EDGE ( 'NONE', *, *, #25276, .F. ) ;
#94847=EDGE_LOOP ( 'NONE', ( #66175, #8794, #62089, #86627 ) ) ;
#94851=AXIS2_PLACEMENT_3D ( 'NONE', #44233, #27071, #65061 ) ;
#94855=ORIENTED_EDGE ( 'NONE', *, *, #97124, .T. ) ;
#94859=DIRECTION ( 'NONE',  ( -0.000000000000000000, 0.000000000000000000, -1.000000000000000000 ) ) ;
#94864=DIRECTION ( 'NONE',  ( 0.9805290675673896672, 0.1963739994383812415, 0.000000000000000000 ) ) ;
#94878=VERTEX_POINT ( 'NONE', #93438 ) ;
#94881=CIRCLE ( 'NONE', #65768, 11.91750000000000043 ) ;
#94889=CARTESIAN_POINT ( 'NONE',  ( 22.66956910419568061, 38.88013629349136835, -10.00000000000000000 ) ) ;
#94910=CARTESIAN_POINT ( 'NONE',  ( -71.61465314115659453, 63.06504152958490295, 60.00000000000000000 ) ) ;
#94911=VERTEX_POINT ( 'NONE', #80759 ) ;
#94913=DIRECTION ( 'NONE',  ( 1.000000000000000000, 0.000000000000000000, 0.000000000000000000 ) ) ;
#94917=FACE_OUTER_BOUND ( 'NONE', #35989, .T. ) ;
#94918=VECTOR ( 'NONE', #34856, 1000.000000000000000 ) ;
#94923=EDGE_CURVE ( 'NONE', #43843, #72251, #26511, .T. ) ;
#94926=CIRCLE ( 'NONE', #7514, 70.00000000000001421 ) ;
#94930=EDGE_LOOP ( 'NONE', ( #3880, #85204, #30477, #47843 ) ) ;
#94937=DIRECTION ( 'NONE',  ( 0.000000000000000000, 0.000000000000000000, 1.000000000000000000 ) ) ;
#94956=ORIENTED_EDGE ( 'NONE', *, *, #51194, .F. ) ;
#94957=EDGE_CURVE ( 'NONE', #32826, #96593, #42674, .T. ) ;
#94962=LINE ( 'NONE', #57914, #98700 ) ;
#94964=EDGE_CURVE ( 'NONE', #88235, #36466, #65007, .T. ) ;
#94965=DIRECTION ( 'NONE',  ( -0.2942337105004269593, -0.9557335003049495237, 0.000000000000000000 ) ) ;
#94966=EDGE_LOOP ( 'NONE', ( #23001, #83595, #55124, #5691 ) ) ;
#94974=VECTOR ( 'NONE', #42058, 1000.000000000000000 ) ;
#94976=EDGE_CURVE ( 'NONE', #6051, #44888, #96442, .T. ) ;
#94985=ORIENTED_EDGE ( 'NONE', *, *, #41323, .T. ) ;
#94987=DIRECTION ( 'NONE',  ( -0.000000000000000000, -0.000000000000000000, -1.000000000000000000 ) ) ;
#94988=CARTESIAN_POINT ( 'NONE',  ( 36.67532856725514989, 51.07057046370195508, -10.00000000000000000 ) ) ;
#94989=DIRECTION ( 'NONE',  ( 0.9888308262251265246, -0.1490422661761876266, 0.000000000000000000 ) ) ;
#95000=UNCERTAINTY_MEASURE_WITH_UNIT (LENGTH_MEASURE( 1.000000000000000082E-05 ), #76207, 'distance_accuracy_value', 'NONE');
#95004=VECTOR ( 'NONE', #43664, 1000.000000000000000 ) ;
#95007=DIRECTION ( 'NONE',  ( 0.000000000000000000, 0.000000000000000000, 1.000000000000000000 ) ) ;
#95014=ORIENTED_EDGE ( 'NONE', *, *, #87119, .T. ) ;
#95023=ADVANCED_FACE ( 'NONE', ( #58383 ), #66980, .F. ) ;
#95034=DIRECTION ( 'NONE',  ( 0.000000000000000000, 0.000000000000000000, 1.000000000000000000 ) ) ;
#95035=PLANE ( 'NONE',  #37125 ) ;
#95036=PLANE ( 'NONE',  #44097 ) ;
#95038=ORIENTED_EDGE ( 'NONE', *, *, #85046, .F. ) ;
#95041=CIRCLE ( 'NONE', #28677, 0.1418229129681557177 ) ;
#95042=CARTESIAN_POINT ( 'NONE',  ( 33.63888670793727442, 47.67824751478843126, -10.00000000000000000 ) ) ;
#95045=VERTEX_POINT ( 'NONE', #27985 ) ;
#95048=AXIS2_PLACEMENT_3D ( 'NONE', #96577, #2344, #27142 ) ;
#95050=EDGE_CURVE ( 'NONE', #62248, #8715, #45176, .T. ) ;
#95052=EDGE_CURVE ( 'NONE', #36208, #40063, #20409, .T. ) ;
#95057=VECTOR ( 'NONE', #87541, 1000.000000000000000 ) ;
#95063=ORIENTED_EDGE ( 'NONE', *, *, #42677, .F. ) ;
#95067=ORIENTED_EDGE ( 'NONE', *, *, #39468, .F. ) ;
#95071=FACE_OUTER_BOUND ( 'NONE', #47860, .T. ) ;
#95072=AXIS2_PLACEMENT_3D ( 'NONE', #32354, #9061, #2475 ) ;
#95076=EDGE_CURVE ( 'NONE', #36862, #11831, #35594, .T. ) ;
#95081=ORIENTED_EDGE ( 'NONE', *, *, #76524, .T. ) ;
#95090=DIRECTION ( 'NONE',  ( 0.3400251696390307887, -0.9404163354663445107, 0.000000000000000000 ) ) ;
#95092=DIRECTION ( 'NONE',  ( 0.4552093898365223712, -0.8903844177683372108, 0.000000000000000000 ) ) ;
#95104=LINE ( 'NONE', #94589, #67369 ) ;
#95114=CARTESIAN_POINT ( 'NONE',  ( 13.90223112049948639, 33.06302660730329279, -10.00000000000000000 ) ) ;
#95115=VERTEX_POINT ( 'NONE', #13786 ) ;
#95116=DIRECTION ( 'NONE',  ( -0.000000000000000000, 0.000000000000000000, -1.000000000000000000 ) ) ;
#95125=CIRCLE ( 'NONE', #15800, 70.00000000000001421 ) ;
#95132=DIRECTION ( 'NONE',  ( 0.02225111142182467291, 0.9997524133706773286, 0.000000000000000000 ) ) ;
#95139=VECTOR ( 'NONE', #91189, 1000.000000000000000 ) ;
#95141=AXIS2_PLACEMENT_3D ( 'NONE', #93324, #23877, #85757 ) ;
#95143=CARTESIAN_POINT ( 'NONE',  ( 20.27804331926714809, 58.17879771734714467, 59.99999999999999289 ) ) ;
#95161=CARTESIAN_POINT ( 'NONE',  ( -59.82327302696293003, 35.73826312759338464, 177.5919119679930134 ) ) ;
#95163=DIRECTION ( 'NONE',  ( 1.000000000000000000, 1.135996059125383208E-13, 0.000000000000000000 ) ) ;
#95174=DIRECTION ( 'NONE',  ( -0.5372068985985076761, -0.8434505012732950169, 0.000000000000000000 ) ) ;
#95178=ORIENTED_EDGE ( 'NONE', *, *, #84316, .F. ) ;
#95186=ORIENTED_EDGE ( 'NONE', *, *, #16900, .F. ) ;
#95187=CARTESIAN_POINT ( 'NONE',  ( -19.42194755839791753, 24.31068691715150010, -10.00000000000000000 ) ) ;
#95199=ORIENTED_EDGE ( 'NONE', *, *, #90683, .T. ) ;
#95201=CARTESIAN_POINT ( 'NONE',  ( -13.90296923609177959, 23.04100004375993649, 10.00000000000000000 ) ) ;
#95207=DIRECTION ( 'NONE',  ( -1.000000000000000000, 0.000000000000000000, 0.000000000000000000 ) ) ;
#95210=CARTESIAN_POINT ( 'NONE',  ( -19.51758400505583069, 93.02331244766838836, 59.99999999999999289 ) ) ;
#95212=CARTESIAN_POINT ( 'NONE',  ( 38.65784837781280459, 56.65029301956751340, 10.00000000000000000 ) ) ;
#95219=CARTESIAN_POINT ( 'NONE',  ( 48.23560136428437772, 110.1272893647940379, -10.00000000000000000 ) ) ;
#95220=VERTEX_POINT ( 'NONE', #34962 ) ;
#95225=EDGE_CURVE ( 'NONE', #91333, #50922, #52529, .T. ) ;
#95227=FACE_OUTER_BOUND ( 'NONE', #89961, .T. ) ;
#95230=DIRECTION ( 'NONE',  ( -0.001368469433204011270, 0.9999990636452668058, 0.000000000000000000 ) ) ;
#95232=VECTOR ( 'NONE', #86232, 1000.000000000000000 ) ;
#95233=VERTEX_POINT ( 'NONE', #83479 ) ;
#95237=LINE ( 'NONE', #19705, #20893 ) ;
#95242=ORIENTED_EDGE ( 'NONE', *, *, #88222, .T. ) ;
#95248=DIRECTION ( 'NONE',  ( -0.000000000000000000, -0.000000000000000000, -1.000000000000000000 ) ) ;
#95251=DIRECTION ( 'NONE',  ( 0.000000000000000000, 0.000000000000000000, 1.000000000000000000 ) ) ;
#95252=ORIENTED_EDGE ( 'NONE', *, *, #46324, .T. ) ;
#95263=VERTEX_POINT ( 'NONE', #59439 ) ;
#95267=AXIS2_PLACEMENT_3D ( 'NONE', #34338, #87617, #18146 ) ;
#95271=CARTESIAN_POINT ( 'NONE',  ( 49.10122569834316408, 93.29622288527660601, -10.00000000000000000 ) ) ;
#95275=DIRECTION ( 'NONE',  ( -0.6141984594095433181, -0.7891516029629184192, 0.000000000000000000 ) ) ;
#95276=CARTESIAN_POINT ( 'NONE',  ( -19.65312891409030271, 93.06504152958497400, 177.5919119679930134 ) ) ;
#95282=ORIENTED_EDGE ( 'NONE', *, *, #99360, .F. ) ;
#95284=DIRECTION ( 'NONE',  ( -1.000000000000000000, 0.000000000000000000, 0.000000000000000000 ) ) ;
#95288=AXIS2_PLACEMENT_3D ( 'NONE', #44870, #82931, #75309 ) ;
#95296=CARTESIAN_POINT ( 'NONE',  ( -62.95439910331221256, 68.06504152958493137, -45.00000000000001421 ) ) ;
#95301=EDGE_CURVE ( 'NONE', #14010, #33732, #45845, .T. ) ;
#95305=EDGE_CURVE ( 'NONE', #98479, #93808, #97683, .T. ) ;
#95310=CARTESIAN_POINT ( 'NONE',  ( -5.928083997560643859, 82.72996031218040969, 13.41116729756204329 ) ) ;
#95321=VERTEX_POINT ( 'NONE', #69553 ) ;
#95332=ORIENTED_EDGE ( 'NONE', *, *, #47887, .T. ) ;
#95334=CARTESIAN_POINT ( 'NONE',  ( -19.68616313074564417, 93.20296353353185737, 59.99999999999999289 ) ) ;
#95335=DIRECTION ( 'NONE',  ( -0.9997524133706772176, 0.02225111142182466945, 0.000000000000000000 ) ) ;
#95366=ORIENTED_EDGE ( 'NONE', *, *, #45986, .F. ) ;
#95372=ADVANCED_FACE ( 'NONE', ( #44741 ), #23439, .F. ) ;
#95379=VERTEX_POINT ( 'NONE', #67556 ) ;
#95381=CARTESIAN_POINT ( 'NONE',  ( 48.53010236944518851, 101.9116055364396090, -10.00000000000000000 ) ) ;
#95388=LINE ( 'NONE', #47704, #86754 ) ;
#95394=LINE ( 'NONE', #27916, #54686 ) ;
#95400=DIRECTION ( 'NONE',  ( 0.000000000000000000, 0.000000000000000000, 1.000000000000000000 ) ) ;
#95401=CARTESIAN_POINT ( 'NONE',  ( -44.74834796241764678, 29.05375577536863929, 10.00000000000000000 ) ) ;
#95403=DIRECTION ( 'NONE',  ( 0.9403255362191060840, -0.3402761906661271873, 0.000000000000000000 ) ) ;
#95406=ORIENTED_EDGE ( 'NONE', *, *, #56178, .T. ) ;
#95407=AXIS2_PLACEMENT_3D ( 'NONE', #70039, #652, #55332 ) ;
#95411=VECTOR ( 'NONE', #25979, 1000.000000000000000 ) ;
#95425=EDGE_CURVE ( 'NONE', #2862, #47702, #54328, .T. ) ;
#95426=VECTOR ( 'NONE', #23728, 1000.000000000000114 ) ;
#95429=DIRECTION ( 'NONE',  ( 0.2774202615135334393, -0.9607486656258038549, 0.000000000000000000 ) ) ;
#95432=DIRECTION ( 'NONE',  ( -1.000000000000000000, -4.892646582054824097E-14, 0.000000000000000000 ) ) ;
#95438=PLANE ( 'NONE',  #35470 ) ;
#95441=CARTESIAN_POINT ( 'NONE',  ( -19.65312891409030271, 93.06504152958497400, 10.00000000000000888 ) ) ;
#95445=AXIS2_PLACEMENT_3D ( 'NONE', #51009, #43407, #35818 ) ;
#95455=DIRECTION ( 'NONE',  ( -0.8435938723211519052, -0.5369817302126803638, 0.000000000000000000 ) ) ;
#95457=ORIENTED_EDGE ( 'NONE', *, *, #12722, .F. ) ;
#95465=DIRECTION ( 'NONE',  ( 0.3002896333693371722, 0.9538480676139722281, 0.000000000000000000 ) ) ;
#95467=CARTESIAN_POINT ( 'NONE',  ( 44.08135397534552880, 118.8355609772188188, -10.00000000000000000 ) ) ;
#95468=ORIENTED_EDGE ( 'NONE', *, *, #28127, .F. ) ;
#95471=CARTESIAN_POINT ( 'NONE',  ( 45.19716250472275476, 70.24742367233086782, -10.00000000000000000 ) ) ;
#95472=VERTEX_POINT ( 'NONE', #45251 ) ;
#95480=VERTEX_POINT ( 'NONE', #30052 ) ;
#95486=AXIS2_PLACEMENT_3D ( 'NONE', #17539, #8446, #92584 ) ;
#95489=ORIENTED_EDGE ( 'NONE', *, *, #83861, .T. ) ;
#95490=FACE_OUTER_BOUND ( 'NONE', #26516, .T. ) ;
#95499=CARTESIAN_POINT ( 'NONE',  ( -19.65312891409030271, 93.06504152958497400, 203.6502102582797420 ) ) ;
#95501=CARTESIAN_POINT ( 'NONE',  ( -19.65312891409030271, 93.06504152958497400, -10.00000000000000888 ) ) ;
#95506=VECTOR ( 'NONE', #98599, 999.9999999999998863 ) ;
#95511=EDGE_CURVE ( 'NONE', #91554, #8241, #84302, .T. ) ;
#95518=CIRCLE ( 'NONE', #38811, 0.1418229129680897982 ) ;
#95521=VERTEX_POINT ( 'NONE', #76659 ) ;
#95544=ORIENTED_EDGE ( 'NONE', *, *, #75666, .T. ) ;
#95551=AXIS2_PLACEMENT_3D ( 'NONE', #35275, #67166, #59549 ) ;
#95553=CARTESIAN_POINT ( 'NONE',  ( 28.70170512279456076, 111.4490886171364821, 59.99999999999999289 ) ) ;
#95554=DIRECTION ( 'NONE',  ( 0.9999580202055560196, 0.009162850352631533510, 0.000000000000000000 ) ) ;
#95555=DIRECTION ( 'NONE',  ( -0.9755587037855265597, 0.2197389712097134185, 0.000000000000000000 ) ) ;
#95560=CARTESIAN_POINT ( 'NONE',  ( -63.52717814648517702, 65.65608168532926925, 59.99999999999999289 ) ) ;
#95561=DIRECTION ( 'NONE',  ( -0.6444573283589029034, 0.7646402761589956576, 0.000000000000000000 ) ) ;
#95571=VECTOR ( 'NONE', #89282, 1000.000000000000000 ) ;
#95577=ORIENTED_EDGE ( 'NONE', *, *, #50652, .F. ) ;
#95581=ORIENTED_EDGE ( 'NONE', *, *, #37258, .T. ) ;
#95589=ORIENTED_EDGE ( 'NONE', *, *, #33178, .T. ) ;
#95594=ORIENTED_EDGE ( 'NONE', *, *, #99668, .T. ) ;
#95597=VERTEX_POINT ( 'NONE', #47735 ) ;
#95608=ADVANCED_FACE ( 'NONE', ( #56843 ), #78671, .F. ) ;
#95611=LINE ( 'NONE', #26160, #17396 ) ;
#95622=VERTEX_POINT ( 'NONE', #39626 ) ;
#95623=CARTESIAN_POINT ( 'NONE',  ( 33.47037235539275457, 49.41749479597460493, 10.00000000000000000 ) ) ;
#95625=EDGE_LOOP ( 'NONE', ( #51685, #36078, #94310, #17280 ) ) ;
#95627=EDGE_CURVE ( 'NONE', #48481, #27644, #24944, .T. ) ;
#95632=DIRECTION ( 'NONE',  ( 1.000000000000000000, 0.000000000000000000, 0.000000000000000000 ) ) ;
#95635=ORIENTED_EDGE ( 'NONE', *, *, #65273, .F. ) ;
#95638=EDGE_CURVE ( 'NONE', #97801, #6804, #23943, .T. ) ;
#95641=DIRECTION ( 'NONE',  ( 0.000000000000000000, 0.000000000000000000, -1.000000000000000000 ) ) ;
#95642=CIRCLE ( 'NONE', #29278, 0.1418229129681557177 ) ;
#95654=DIRECTION ( 'NONE',  ( 0.6361630342459738685, -0.7715546603183444097, 0.000000000000000000 ) ) ;
#95658=LINE ( 'NONE', #51485, #25592 ) ;
#95669=CARTESIAN_POINT ( 'NONE',  ( 13.67211979723576931, 32.92651376809308772, 10.00000000000000000 ) ) ;
#95670=FACE_OUTER_BOUND ( 'NONE', #22659, .T. ) ;
#95672=EDGE_CURVE ( 'NONE', #5345, #79622, #5638, .T. ) ;
#95682=CARTESIAN_POINT ( 'NONE',  ( 42.55442611339157821, 60.96799964870728417, 10.00000000000000000 ) ) ;
#95683=EDGE_CURVE ( 'NONE', #59100, #37455, #68923, .T. ) ;
#95686=DIRECTION ( 'NONE',  ( -1.000000000000000000, 0.000000000000000000, 0.000000000000000000 ) ) ;
#95688=FACE_OUTER_BOUND ( 'NONE', #97699, .T. ) ;
#95692=ORIENTED_EDGE ( 'NONE', *, *, #44824, .F. ) ;
#95701=CARTESIAN_POINT ( 'NONE',  ( 42.65610334793076674, 64.00004027534475881, 10.00000000000000000 ) ) ;
#95705=EDGE_LOOP ( 'NONE', ( #62789, #41926, #90728, #26578 ) ) ;
#95708=CARTESIAN_POINT ( 'NONE',  ( -19.65312891409030271, 93.06504152958497400, 177.5919119679930134 ) ) ;
#95710=ORIENTED_EDGE ( 'NONE', *, *, #28666, .T. ) ;
#95712=ORIENTED_EDGE ( 'NONE', *, *, #93204, .F. ) ;
#95724=ORIENTED_EDGE ( 'NONE', *, *, #36636, .F. ) ;
#95725=DIRECTION ( 'NONE',  ( 0.000000000000000000, -0.000000000000000000, -1.000000000000000000 ) ) ;
#95738=EDGE_LOOP ( 'NONE', ( #42713, #61599, #14191, #59663 ) ) ;
#95752=EDGE_CURVE ( 'NONE', #7444, #66626, #98864, .T. ) ;
#95763=DIRECTION ( 'NONE',  ( 1.000000000000000000, 0.000000000000000000, 0.000000000000000000 ) ) ;
#95769=LINE ( 'NONE', #94747, #49881 ) ;
#95773=AXIS2_PLACEMENT_3D ( 'NONE', #79601, #62332, #30947 ) ;
#95774=EDGE_CURVE ( 'NONE', #24730, #72762, #82698, .T. ) ;
#95777=ORIENTED_EDGE ( 'NONE', *, *, #34860, .T. ) ;
#95790=DIRECTION ( 'NONE',  ( -0.9506327454577400138, -0.3103181967972222788, 0.000000000000000000 ) ) ;
#95793=EDGE_CURVE ( 'NONE', #37421, #6372, #58798, .T. ) ;
#95797=LINE ( 'NONE', #42034, #37745 ) ;
#95801=ORIENTED_EDGE ( 'NONE', *, *, #9504, .T. ) ;
#95805=ORIENTED_EDGE ( 'NONE', *, *, #31086, .F. ) ;
#95814=ORIENTED_EDGE ( 'NONE', *, *, #39399, .F. ) ;
#95822=CYLINDRICAL_SURFACE ( 'NONE', #54943, 60.00000000000002132 ) ;
#95823=DIRECTION ( 'NONE',  ( -0.7226656227773308183, -0.6911977992267138715, 0.000000000000000000 ) ) ;
#95827=DIRECTION ( 'NONE',  ( -1.000000000000000000, 0.000000000000000000, 0.000000000000000000 ) ) ;
#95831=PLANE ( 'NONE',  #80443 ) ;
#95838=VERTEX_POINT ( 'NONE', #63831 ) ;
#95840=ORIENTED_EDGE ( 'NONE', *, *, #74715, .F. ) ;
#95848=CARTESIAN_POINT ( 'NONE',  ( -19.65312891409030271, 93.06504152958497400, -10.00000000000000888 ) ) ;
#95849=ORIENTED_EDGE ( 'NONE', *, *, #14071, .F. ) ;
#95850=FACE_OUTER_BOUND ( 'NONE', #75843, .T. ) ;
#95853=DIRECTION ( 'NONE',  ( 1.000000000000000000, 0.000000000000000000, 0.000000000000000000 ) ) ;
#95898=CIRCLE ( 'NONE', #68357, 60.00000000000002132 ) ;
#95900=CARTESIAN_POINT ( 'NONE',  ( 29.30989995549245464, 44.80713248141895377, -10.00000000000000000 ) ) ;
#95905=CARTESIAN_POINT ( 'NONE',  ( 46.80869107419874098, 110.6443039040113092, -10.00000000000000000 ) ) ;
#95913=CARTESIAN_POINT ( 'NONE',  ( -19.65312891409030271, 93.06504152958497400, -10.00000000000000888 ) ) ;
#95915=CYLINDRICAL_SURFACE ( 'NONE', #13486, 70.00000000000002842 ) ;
#95927=ADVANCED_FACE ( 'NONE', ( #52133 ), #35936, .T. ) ;
#95931=PLANE ( 'NONE',  #83001 ) ;
#95935=CARTESIAN_POINT ( 'NONE',  ( 37.34220537994157496, 54.61056725541210710, 10.00000000000000000 ) ) ;
#95949=ORIENTED_EDGE ( 'NONE', *, *, #36937, .F. ) ;
#95960=LINE ( 'NONE', #41190, #82757 ) ;
#95966=ORIENTED_EDGE ( 'NONE', *, *, #10322, .T. ) ;
#95972=DIRECTION ( 'NONE',  ( 0.000000000000000000, -0.000000000000000000, 1.000000000000000000 ) ) ;
#95975=CIRCLE ( 'NONE', #26440, 0.1418229129680897982 ) ;
#95976=ORIENTED_EDGE ( 'NONE', *, *, #88010, .F. ) ;
#95982=ORIENTED_EDGE ( 'NONE', *, *, #54191, .T. ) ;
#95983=VERTEX_POINT ( 'NONE', #67849 ) ;
#95995=EDGE_CURVE ( 'NONE', #70584, #38287, #36938, .T. ) ;
#95997=ADVANCED_FACE ( 'NONE', ( #74478 ), #37832, .F. ) ;
#96011=CARTESIAN_POINT ( 'NONE',  ( 49.54000814145099696, 103.6626726051169527, 10.00000000000000000 ) ) ;
#96016=ORIENTED_EDGE ( 'NONE', *, *, #42541, .F. ) ;
#96019=CARTESIAN_POINT ( 'NONE',  ( 5.181765596169280563, 27.61866642244642733, -10.00000000000000000 ) ) ;
#96023=CARTESIAN_POINT ( 'NONE',  ( -24.40473831032599961, 23.22649767201583515, -10.00000000000000000 ) ) ;
#96025=AXIS2_PLACEMENT_3D ( 'NONE', #90177, #20752, #28325 ) ;
#96032=FACE_OUTER_BOUND ( 'NONE', #16207, .T. ) ;
#96033=VECTOR ( 'NONE', #63092, 1000.000000000000000 ) ;
#96038=VECTOR ( 'NONE', #53716, 1000.000000000000000 ) ;
#96039=DIRECTION ( 'NONE',  ( 0.8902628732232650277, -0.4554470513245822971, 0.000000000000000000 ) ) ;
#96041=CARTESIAN_POINT ( 'NONE',  ( 11.84209618866182190, 52.02562058438156356, 59.99999999999999289 ) ) ;
#96042=ORIENTED_EDGE ( 'NONE', *, *, #33375, .F. ) ;
#96046=PLANE ( 'NONE',  #23217 ) ;
#96053=LINE ( 'NONE', #58000, #97340 ) ;
#96054=CARTESIAN_POINT ( 'NONE',  ( 48.16808589598787904, 104.3116767361652535, -10.00000000000000000 ) ) ;
#96065=CARTESIAN_POINT ( 'NONE',  ( -44.49648453423614569, 28.96346851210257967, -10.00000000000000000 ) ) ;
#96076=ORIENTED_EDGE ( 'NONE', *, *, #34637, .F. ) ;
#96080=CARTESIAN_POINT ( 'NONE',  ( 31.78345146745886751, 98.58241053160183753, 59.99999999999999289 ) ) ;
#96082=ORIENTED_EDGE ( 'NONE', *, *, #43187, .T. ) ;
#96088=DIRECTION ( 'NONE',  ( 1.000000000000000000, 0.000000000000000000, 0.000000000000000000 ) ) ;
#96089=LINE ( 'NONE', #97086, #22678 ) ;
#96091=DIRECTION ( 'NONE',  ( -0.9458118053197299702, 0.3247153044096216523, 0.000000000000000000 ) ) ;
#96095=CLOSED_SHELL ( 'NONE', ( #95997, #13969, #92312, #54742, #8921, #3780, #67974, #92518, #46291, #89425, #86061, #91245, #44052, #74986, #92542, #69015, #47458, #42489, #27470, #26187, #58736, #38966, #55772, #28210, #12592, #80328, #70318, #20088, #88910, #88366, #23517, #29118, #39972, #90127, #68391, #44494, #17819, #3901, #17026, #92092, #99281, #65310, #23883, #86947, #11105, #55452, #12785, #65068, #74911, #41731, #40014, #14112, #23645, #49131, #48581, #51403, #46388, #88946, #25051, #37149, #8072, #12017, #37460, #16864, #98131, #33764, #46628, #35027, #52072, #63407, #23980, #57717, #46171, #75933, #42805, #54342, #97144, #96779, #18467, #42926, #55535, #14287, #71707, #23893, #96877, #85248, #34921, #74152, #94709, #76885, #13296, #65864, #83631, #76530, #22792, #26019, #82048, #18816, #10150, #89145, #43322, #60936, #6516, #84063, #5359, #75388, #37019, #82744, #61630, #79731, #92867, #4550, #64284, #55755, #83556, #42074, #95927, #93828, #69533, #36111, #96162, #38267, #73814, #78932, #70662, #18842, #76251, #19492, #26442, #2705, #63876, #68542, #91460, #82748, #31976, #41116, #82010, #35441, #65376, #89798, #42312, #21474, #84944, #7396, #60294, #83503, #48326, #24171, #78183, #53016, #12559, #67814, #74726, #23733, #89074, #20587, #8235, #67053, #43097, #65795, #16580, #46982, #59178, #56691, #51455, #44125, #54070, #8232, #14943, #85108, #47494, #60351, #21944, #58971, #53614, #83254, #80543, #5497, #80082, #59108, #68761, #89154, #16990, #72200, #82124, #54000, #23133, #70411, #53820, #58558, #89098, #31842, #5476, #27214, #37446, #98224, #34520, #61632, #3042, #16431, #16181, #15586, #29001, #27708, #27123, #69797, #2760, #67557, #24440, #43640, #33930, #86993, #6727, #85729, #60867, #68924, #74908, #75225, #52029, #93243, #86800, #66438, #99037, #21948, #76654, #54750, #15836, #40332, #33136, #2409, #6340, #43506, #74804, #26447, #94719, #94592, #71310, #42861, #16342, #91886, #99392, #7480, #53668, #20651, #877, #82932, #37938, #26389, #99800, #40656, #60473, #33721, #40405, #85000, #65818, #52743, #52804, #57292, #80078, #67507, #67944, #99603, #41555, #796, #84635, #39318, #73029, #33255, #51515, #72854, #37135, #64740, #54625, #20131, #5988, #52574, #95023, #34087, #10115, #33168, #3960, #66411, #58655, #49562, #13364, #31207, #8465, #49014, #73294, #63798, #27055, #24429, #67715, #60184, #3529, #70473, #1754, #65189, #12835, #96929, #60566, #91295, #99266, #8118, #56604, #29786, #62262, #49729, #38138, #16922, #66502, #65173, #96870, #36626, #22665, #73149, #52375, #51381, #62059, #5391, #92747, #9496, #6011, #36007, #59299, #81553, #29710, #67788, #83423, #38213, #19595, #95608, #98109, #36126, #41141, #67632, #72407, #65633, #7405, #24636, #53466, #52481, #78906, #14837, #52648, #59807, #84756, #72003, #14516, #98710, #48236, #20545, #61440, #41284, #56022, #5790, #27740, #25830, #66529, #12597, #89365, #16105, #58544, #4912, #62733, #10191, #99977, #3112, #8733, #34515, #84010, #3612, #92327, #21289, #40213, #78249, #71441, #9568, #81313, #35123, #44319, #84783, #58394, #30074, #20718, #33426, #94381, #22730, #43445, #60361, #45705, #61591, #52878, #15447, #73266, #51062, #39974, #3896, #21218, #68490, #50079, #69720, #79535, #627, #72786, #98717, #19794, #95372, #92390, #19068, #19561, #61376, #60305, #30774, #63234, #3099, #68456, #210, #49630, #64794, #20248, #60567, #87688, #2073, #73583, #26707, #4501, #96301, #63221, #78304, #56980, #81914, #40910, #92214, #87578, #99934, #22036, #20270, #62940, #63518, #18278, #51926, #86924, #61332, #99607, #69756, #89749, #76297, #93209, #94550, #78792, #47347, #83239, #77926, #41685, #52461, #74679, #86523, #40219, #81355, #28250, #5130, #73998, #7080, #24252, #75157, #56132, #18605, #46577, #16799, #15329, #41162, #24107, #71130, #15767, #18032, #51585, #75854, #4329, #13289, #100179, #5826, #71499, #18013, #40097, #32488, #84664, #15726, #13597 ) ) ;
#96097=VERTEX_POINT ( 'NONE', #36431 ) ;
#96104=( GEOMETRIC_REPRESENTATION_CONTEXT ( 3 ) GLOBAL_UNCERTAINTY_ASSIGNED_CONTEXT ( ( #9879 ) ) GLOBAL_UNIT_ASSIGNED_CONTEXT ( ( #84711, #79620, #10184 ) ) REPRESENTATION_CONTEXT ( 'NONE', 'WORKASPACE' ) );
#96111=VERTEX_POINT ( 'NONE', #20260 ) ;
#96112=FACE_OUTER_BOUND ( 'NONE', #76004, .T. ) ;
#96113=EDGE_CURVE ( 'NONE', #70676, #58533, #63740, .T. ) ;
#96119=CARTESIAN_POINT ( 'NONE',  ( -67.91103796225580425, 44.10201266000169795, 10.00000000000000000 ) ) ;
#96121=DIRECTION ( 'NONE',  ( -0.000000000000000000, -0.000000000000000000, -1.000000000000000000 ) ) ;
#96122=ORIENTED_EDGE ( 'NONE', *, *, #76284, .T. ) ;
#96129=CARTESIAN_POINT ( 'NONE',  ( 18.97183685527354413, 49.87166901558443044, 59.99999999999999289 ) ) ;
#96147=CARTESIAN_POINT ( 'NONE',  ( -19.65312891409030271, 93.06504152958497400, 10.00000000000000888 ) ) ;
#96152=EDGE_CURVE ( 'NONE', #65825, #17797, #66981, .T. ) ;
#96156=ORIENTED_EDGE ( 'NONE', *, *, #44947, .F. ) ;
#96162=ADVANCED_FACE ( 'NONE', ( #44020 ), #74963, .T. ) ;
#96163=ORIENTED_EDGE ( 'NONE', *, *, #42407, .F. ) ;
#96164=CARTESIAN_POINT ( 'NONE',  ( -19.65312891409030271, 93.06504152958497400, 59.99999999999999289 ) ) ;
#96170=ORIENTED_EDGE ( 'NONE', *, *, #72576, .T. ) ;
#96174=CARTESIAN_POINT ( 'NONE',  ( 41.49446470602975978, 58.46153712902343358, 10.00000000000000000 ) ) ;
#96175=EDGE_CURVE ( 'NONE', #75021, #98005, #90188, .T. ) ;
#96181=LINE ( 'NONE', #33867, #45781 ) ;
#96185=ORIENTED_EDGE ( 'NONE', *, *, #58991, .F. ) ;
#96190=EDGE_CURVE ( 'NONE', #21282, #934, #97736, .T. ) ;
#96199=DIRECTION ( 'NONE',  ( 0.9171038997749326738, -0.3986482622784278673, 0.000000000000000000 ) ) ;
#96203=CARTESIAN_POINT ( 'NONE',  ( -71.61465314115659453, 63.06504152958490295, -20.00000000000001776 ) ) ;
#96213=DIRECTION ( 'NONE',  ( -1.000000000000000000, 0.000000000000000000, 0.000000000000000000 ) ) ;
#96215=CARTESIAN_POINT ( 'NONE',  ( -19.66077996331566524, 93.20665791313032855, 59.99999999999999289 ) ) ;
#96220=ORIENTED_EDGE ( 'NONE', *, *, #93357, .T. ) ;
#96228=PLANE ( 'NONE',  #9197 ) ;
#96229=ORIENTED_EDGE ( 'NONE', *, *, #60001, .F. ) ;
#96237=LINE ( 'NONE', #81052, #64557 ) ;
#96241=CARTESIAN_POINT ( 'NONE',  ( -66.43946475426807297, 58.88062878445797566, 59.99999999999999289 ) ) ;
#96248=VECTOR ( 'NONE', #15907, 1000.000000000000000 ) ;
#96272=FACE_OUTER_BOUND ( 'NONE', #21674, .T. ) ;
#96275=DIRECTION ( 'NONE',  ( 0.000000000000000000, 0.000000000000000000, 1.000000000000000000 ) ) ;
#96277=DIRECTION ( 'NONE',  ( 0.8902628732232650277, -0.4554470513245822971, 0.000000000000000000 ) ) ;
#96287=DIRECTION ( 'NONE',  ( -1.000000000000000000, 0.000000000000000000, 0.000000000000000000 ) ) ;
#96292=CARTESIAN_POINT ( 'NONE',  ( -71.61465314115659453, 63.06504152958490295, 40.00000000000000000 ) ) ;
#96295=CARTESIAN_POINT ( 'NONE',  ( -19.65312891409030271, 93.06504152958497400, 177.5919119679930134 ) ) ;
#96297=EDGE_CURVE ( 'NONE', #9798, #14868, #68716, .T. ) ;
#96299=CARTESIAN_POINT ( 'NONE',  ( -19.65312891409030271, 93.06504152958497400, 10.00000000000000888 ) ) ;
#96301=ADVANCED_FACE ( 'NONE', ( #99140 ), #52518, .F. ) ;
#96304=AXIS2_PLACEMENT_3D ( 'NONE', #52915, #83867, #6326 ) ;
#96306=EDGE_LOOP ( 'NONE', ( #95038, #58212, #56556, #96076 ) ) ;
#96325=FACE_BOUND ( 'NONE', #91463, .T. ) ;
#96332=ORIENTED_EDGE ( 'NONE', *, *, #27783, .F. ) ;
#96333=EDGE_CURVE ( 'NONE', #14660, #29175, #99640, .T. ) ;
#96348=LINE ( 'NONE', #20822, #46408 ) ;
#96352=VERTEX_POINT ( 'NONE', #15500 ) ;
#96355=DIRECTION ( 'NONE',  ( 0.000000000000000000, 0.000000000000000000, 1.000000000000000000 ) ) ;
#96359=DIRECTION ( 'NONE',  ( -1.000000000000000000, 0.000000000000000000, 0.000000000000000000 ) ) ;
#96380=ORIENTED_EDGE ( 'NONE', *, *, #97480, .F. ) ;
#96381=EDGE_CURVE ( 'NONE', #92554, #98025, #93044, .T. ) ;
#96382=VECTOR ( 'NONE', #89561, 1000.000000000000000 ) ;
#96389=FACE_OUTER_BOUND ( 'NONE', #22263, .T. ) ;
#96401=CARTESIAN_POINT ( 'NONE',  ( -19.65312891409030271, 93.06504152958497400, 10.00000000000000888 ) ) ;
#96412=CARTESIAN_POINT ( 'NONE',  ( -36.52772323645827868, 26.41323893245352039, -10.00000000000000000 ) ) ;
#96415=DIRECTION ( 'NONE',  ( 0.000000000000000000, -0.000000000000000000, -1.000000000000000000 ) ) ;
#96420=ORIENTED_EDGE ( 'NONE', *, *, #60755, .F. ) ;
#96425=EDGE_CURVE ( 'NONE', #11558, #100173, #83466, .T. ) ;
#96426=ORIENTED_EDGE ( 'NONE', *, *, #50619, .T. ) ;
#96434=VERTEX_POINT ( 'NONE', #80365 ) ;
#96441=ORIENTED_EDGE ( 'NONE', *, *, #22653, .T. ) ;
#96442=LINE ( 'NONE', #55866, #5461 ) ;
#96448=AXIS2_PLACEMENT_3D ( 'NONE', #97595, #96121, #80424 ) ;
#96450=CARTESIAN_POINT ( 'NONE',  ( 10.06845959268932411, 31.07446838803123157, -10.00000000000000000 ) ) ;
#96451=ORIENTED_EDGE ( 'NONE', *, *, #95638, .F. ) ;
#96459=ORIENTED_EDGE ( 'NONE', *, *, #93892, .F. ) ;
#96466=CYLINDRICAL_SURFACE ( 'NONE', #11132, 70.00000000000002842 ) ;
#96478=DIRECTION ( 'NONE',  ( 0.000000000000000000, 0.000000000000000000, -1.000000000000000000 ) ) ;
#96494=CARTESIAN_POINT ( 'NONE',  ( 46.30674614090289509, 112.4688969640381231, -10.00000000000000000 ) ) ;
#96516=CARTESIAN_POINT ( 'NONE',  ( 32.47331203838563596, 45.95596728736418868, -10.00000000000000000 ) ) ;
#96532=FACE_OUTER_BOUND ( 'NONE', #31517, .T. ) ;
#96534=ORIENTED_EDGE ( 'NONE', *, *, #60630, .T. ) ;
#96538=LINE ( 'NONE', #13885, #70935 ) ;
#96548=EDGE_CURVE ( 'NONE', #34660, #85223, #41809, .T. ) ;
#96553=FACE_OUTER_BOUND ( 'NONE', #55272, .T. ) ;
#96554=EDGE_CURVE ( 'NONE', #14044, #38349, #65119, .T. ) ;
#96556=CARTESIAN_POINT ( 'NONE',  ( -71.61465314115659453, 63.06504152958490295, -20.00000000000001776 ) ) ;
#96558=DIRECTION ( 'NONE',  ( -0.3958915996110536351, -0.9182972510888840478, 0.000000000000000000 ) ) ;
#96562=VERTEX_POINT ( 'NONE', #40298 ) ;
#96568=ORIENTED_EDGE ( 'NONE', *, *, #81984, .T. ) ;
#96571=AXIS2_PLACEMENT_3D ( 'NONE', #29776, #37363, #60649 ) ;
#96577=CARTESIAN_POINT ( 'NONE',  ( -77.42978507651396569, 55.80833764325424085, -10.00000000000000000 ) ) ;
#96578=VECTOR ( 'NONE', #97686, 1000.000000000000000 ) ;
#96593=VERTEX_POINT ( 'NONE', #17009 ) ;
#96599=VECTOR ( 'NONE', #15784, 1000.000000000000114 ) ;
#96601=CARTESIAN_POINT ( 'NONE',  ( -43.70040200909112116, 27.32518560721127088, -10.00000000000000000 ) ) ;
#96612=ORIENTED_EDGE ( 'NONE', *, *, #2461, .F. ) ;
#96616=DIRECTION ( 'NONE',  ( 0.000000000000000000, 0.000000000000000000, 1.000000000000000000 ) ) ;
#96621=ORIENTED_EDGE ( 'NONE', *, *, #8219, .T. ) ;
#96627=LINE ( 'NONE', #66185, #93574 ) ;
#96632=DIRECTION ( 'NONE',  ( -1.000000000000000000, 0.000000000000000000, 0.000000000000000000 ) ) ;
#96634=VECTOR ( 'NONE', #26691, 1000.000000000000227 ) ;
#96643=AXIS2_PLACEMENT_3D ( 'NONE', #47939, #9466, #94098 ) ;
#96656=ORIENTED_EDGE ( 'NONE', *, *, #42251, .F. ) ;
#96660=CARTESIAN_POINT ( 'NONE',  ( 30.80155721116056355, 46.36891074996812989, -10.00000000000000000 ) ) ;
#96670=ORIENTED_EDGE ( 'NONE', *, *, #15197, .T. ) ;
#96676=ORIENTED_EDGE ( 'NONE', *, *, #69523, .T. ) ;
#96683=DIRECTION ( 'NONE',  ( -0.000000000000000000, -0.000000000000000000, -1.000000000000000000 ) ) ;
#96688=DIRECTION ( 'NONE',  ( -0.8263106059122556912, -0.5632146860273805622, 0.000000000000000000 ) ) ;
#96691=DIRECTION ( 'NONE',  ( 0.000000000000000000, 0.000000000000000000, 1.000000000000000000 ) ) ;
#96695=CARTESIAN_POINT ( 'NONE',  ( -19.65312891409030271, 93.06504152958497400, 177.5919119679930134 ) ) ;
#96697=DIRECTION ( 'NONE',  ( 0.2942337105004269593, 0.9557335003049495237, 0.000000000000000000 ) ) ;
#96700=FACE_OUTER_BOUND ( 'NONE', #60138, .T. ) ;
#96701=DIRECTION ( 'NONE',  ( -1.000000000000000000, 0.000000000000000000, 0.000000000000000000 ) ) ;
#96706=VECTOR ( 'NONE', #52187, 1000.000000000000000 ) ;
#96718=VECTOR ( 'NONE', #58727, 1000.000000000000000 ) ;
#96720=CARTESIAN_POINT ( 'NONE',  ( 6.117390533544194930, 29.33055864014943026, 10.00000000000000000 ) ) ;
#96727=DIRECTION ( 'NONE',  ( 0.000000000000000000, 0.000000000000000000, 1.000000000000000000 ) ) ;
#96739=LINE ( 'NONE', #57182, #2897 ) ;
#96749=EDGE_CURVE ( 'NONE', #53524, #88734, #57508, .T. ) ;
#96750=DIRECTION ( 'NONE',  ( -0.000000000000000000, 0.000000000000000000, -1.000000000000000000 ) ) ;
#96755=DIRECTION ( 'NONE',  ( 1.000000000000000000, 0.000000000000000000, 0.000000000000000000 ) ) ;
#96762=AXIS2_PLACEMENT_3D ( 'NONE', #89690, #42035, #26351 ) ;
#96764=FACE_OUTER_BOUND ( 'NONE', #28597, .T. ) ;
#96775=VECTOR ( 'NONE', #96558, 1000.000000000000227 ) ;
#96779=ADVANCED_FACE ( 'NONE', ( #11935 ), #75227, .T. ) ;
#96782=CARTESIAN_POINT ( 'NONE',  ( 11.76667899187106059, 31.90941714274742580, -10.00000000000000000 ) ) ;
#96786=FACE_OUTER_BOUND ( 'NONE', #58109, .T. ) ;
#96788=ORIENTED_EDGE ( 'NONE', *, *, #78042, .F. ) ;
#96791=CARTESIAN_POINT ( 'NONE',  ( -9.674045898528673249, 85.30406559775344988, 14.22504367373031364 ) ) ;
#96803=ORIENTED_EDGE ( 'NONE', *, *, #24300, .F. ) ;
#96818=ORIENTED_EDGE ( 'NONE', *, *, #35158, .F. ) ;
#96820=DIRECTION ( 'NONE',  ( -0.6303371332823576312, -0.7763215174174805666, 0.000000000000000000 ) ) ;
#96826=ORIENTED_EDGE ( 'NONE', *, *, #19477, .T. ) ;
#96828=EDGE_LOOP ( 'NONE', ( #80610, #37691, #78319, #1080 ) ) ;
#96841=ORIENTED_EDGE ( 'NONE', *, *, #19363, .F. ) ;
#96843=CARTESIAN_POINT ( 'NONE',  ( -79.28667360730980818, 56.40661347651924729, 177.5919119679930134 ) ) ;
#96846=CIRCLE ( 'NONE', #27313, 70.00000000000001421 ) ;
#96851=LINE ( 'NONE', #3625, #75243 ) ;
#96854=AXIS2_PLACEMENT_3D ( 'NONE', #13203, #91214, #82138 ) ;
#96856=VERTEX_POINT ( 'NONE', #44789 ) ;
#96858=DIRECTION ( 'NONE',  ( 0.5270369400482041167, 0.8498423758701525443, 0.000000000000000000 ) ) ;
#96863=LINE ( 'NONE', #27431, #95571 ) ;
#96866=AXIS2_PLACEMENT_3D ( 'NONE', #61083, #46372, #77302 ) ;
#96867=CARTESIAN_POINT ( 'NONE',  ( -50.81821011400020183, 81.52126639084015380, -10.00000000000000000 ) ) ;
#96870=ADVANCED_FACE ( 'NONE', ( #91953 ), #29610, .F. ) ;
#96872=DIRECTION ( 'NONE',  ( -1.000000000000000000, 0.000000000000000000, 0.000000000000000000 ) ) ;
#96877=ADVANCED_FACE ( 'NONE', ( #21516 ), #99024, .T. ) ;
#96878=DIRECTION ( 'NONE',  ( 0.9890802632347824863, -0.1473778574936323582, 0.000000000000000000 ) ) ;
#96883=VECTOR ( 'NONE', #44600, 1000.000000000000000 ) ;
#96890=AXIS2_PLACEMENT_3D ( 'NONE', #17334, #68165, #61555 ) ;
#96897=PLANE ( 'NONE',  #14114 ) ;
#96899=EDGE_CURVE ( 'NONE', #16029, #44653, #61492, .T. ) ;
#96910=LINE ( 'NONE', #65464, #27416 ) ;
#96918=CARTESIAN_POINT ( 'NONE',  ( -19.65312891409030271, 93.06504152958497400, -45.00000000000001421 ) ) ;
#96919=AXIS2_PLACEMENT_3D ( 'NONE', #57647, #89133, #96701 ) ;
#96923=CARTESIAN_POINT ( 'NONE',  ( 2.064617007569734319, 27.83817977871672511, -10.00000000000000000 ) ) ;
#96926=ORIENTED_EDGE ( 'NONE', *, *, #70067, .F. ) ;
#96929=ADVANCED_FACE ( 'NONE', ( #40179 ), #85871, .F. ) ;
#96936=ORIENTED_EDGE ( 'NONE', *, *, #26318, .T. ) ;
#96951=ORIENTED_EDGE ( 'NONE', *, *, #24320, .F. ) ;
#96961=ORIENTED_EDGE ( 'NONE', *, *, #74590, .T. ) ;
#96962=FACE_OUTER_BOUND ( 'NONE', #68481, .T. ) ;
#96967=DIRECTION ( 'NONE',  ( -0.9439450758449140499, 0.3301025504114431519, 0.000000000000000000 ) ) ;
#96972=ORIENTED_EDGE ( 'NONE', *, *, #15571, .T. ) ;
#96985=ORIENTED_EDGE ( 'NONE', *, *, #66377, .F. ) ;
#96987=DIRECTION ( 'NONE',  ( 0.000000000000000000, 0.000000000000000000, 1.000000000000000000 ) ) ;
#96995=VECTOR ( 'NONE', #93931, 1000.000000000000000 ) ;
#97000=CARTESIAN_POINT ( 'NONE',  ( -62.95439910331221256, 68.06504152958493137, 20.00000000000000355 ) ) ;
#97001=VERTEX_POINT ( 'NONE', #10310 ) ;
#97017=AXIS2_PLACEMENT_3D ( 'NONE', #79968, #49034, #77036 ) ;
#97021=LINE ( 'NONE', #66568, #48354 ) ;
#97024=LINE ( 'NONE', #20490, #20749 ) ;
#97030=DIRECTION ( 'NONE',  ( -0.000000000000000000, -0.000000000000000000, -1.000000000000000000 ) ) ;
#97034=LINE ( 'NONE', #34680, #59706 ) ;
#97035=CARTESIAN_POINT ( 'NONE',  ( 17.55280445478281592, 33.77154675864928635, 10.00000000000000000 ) ) ;
#97045=EDGE_LOOP ( 'NONE', ( #94562, #98784, #12873, #35216 ) ) ;
#97053=CARTESIAN_POINT ( 'NONE',  ( -79.28667360730979397, 56.40661347651924729, 10.00000000000000000 ) ) ;
#97060=FACE_OUTER_BOUND ( 'NONE', #6821, .T. ) ;
#97061=VERTEX_POINT ( 'NONE', #46028 ) ;
#97062=AXIS2_PLACEMENT_3D ( 'NONE', #26100, #40766, #16977 ) ;
#97072=ORIENTED_EDGE ( 'NONE', *, *, #35055, .T. ) ;
#97073=ORIENTED_EDGE ( 'NONE', *, *, #29040, .F. ) ;
#97074=LINE ( 'NONE', #97553, #2830 ) ;
#97075=ORIENTED_EDGE ( 'NONE', *, *, #9716, .F. ) ;
#97077=ORIENTED_EDGE ( 'NONE', *, *, #6397, .F. ) ;
#97079=VECTOR ( 'NONE', #81805, 1000.000000000000000 ) ;
#97084=DIRECTION ( 'NONE',  ( -0.5632146860273895550, 0.8263106059122495850, 0.000000000000000000 ) ) ;
#97085=EDGE_CURVE ( 'NONE', #63052, #70901, #33000, .T. ) ;
#97086=CARTESIAN_POINT ( 'NONE',  ( 36.67532856725514989, 51.07057046370195508, 10.00000000000000000 ) ) ;
#97097=ORIENTED_EDGE ( 'NONE', *, *, #20597, .F. ) ;
#97120=ORIENTED_EDGE ( 'NONE', *, *, #95225, .F. ) ;
#97124=EDGE_CURVE ( 'NONE', #74676, #91738, #85090, .T. ) ;
#97125=FACE_OUTER_BOUND ( 'NONE', #90476, .T. ) ;
#97129=EDGE_CURVE ( 'NONE', #13582, #88229, #61739, .T. ) ;
#97143=CIRCLE ( 'NONE', #89150, 0.1418229129680828593 ) ;
#97144=ADVANCED_FACE ( 'NONE', ( #92689 ), #46532, .T. ) ;
#97145=DIRECTION ( 'NONE',  ( -0.000000000000000000, 0.000000000000000000, -1.000000000000000000 ) ) ;
#97146=EDGE_CURVE ( 'NONE', #7311, #55128, #56648, .T. ) ;
#97155=LINE ( 'NONE', #28707, #41853 ) ;
#97157=ORIENTED_EDGE ( 'NONE', *, *, #45604, .T. ) ;
#97159=CARTESIAN_POINT ( 'NONE',  ( 49.07419501245632176, 91.40403951869188859, 10.00000000000000000 ) ) ;
#97164=DIRECTION ( 'NONE',  ( -0.000000000000000000, 0.000000000000000000, -1.000000000000000000 ) ) ;
#97175=CARTESIAN_POINT ( 'NONE',  ( -19.65312891409030271, 93.06504152958497400, 10.00000000000000888 ) ) ;
#97176=ORIENTED_EDGE ( 'NONE', *, *, #27729, .F. ) ;
#97182=EDGE_CURVE ( 'NONE', #40677, #49707, #33878, .T. ) ;
#97188=ORIENTED_EDGE ( 'NONE', *, *, #37215, .F. ) ;
#97202=FACE_OUTER_BOUND ( 'NONE', #6826, .T. ) ;
#97206=ORIENTED_EDGE ( 'NONE', *, *, #98229, .F. ) ;
#97208=CARTESIAN_POINT ( 'NONE',  ( 49.63464994930628649, 103.0251469596019120, 10.00000000000000000 ) ) ;
#97212=ORIENTED_EDGE ( 'NONE', *, *, #40586, .T. ) ;
#97213=AXIS2_PLACEMENT_3D ( 'NONE', #9350, #45824, #1766 ) ;
#97216=ORIENTED_EDGE ( 'NONE', *, *, #55034, .T. ) ;
#97234=CARTESIAN_POINT ( 'NONE',  ( -51.91772629337628331, 101.0347834704168122, -10.00000000000000000 ) ) ;
#97237=DIRECTION ( 'NONE',  ( -0.000000000000000000, -0.000000000000000000, 1.000000000000000000 ) ) ;
#97246=DIRECTION ( 'NONE',  ( 0.6647600172776847449, -0.7470569720101488675, 0.000000000000000000 ) ) ;
#97267=DIRECTION ( 'NONE',  ( -0.3851501363289908109, 0.9228539280329036698, 0.000000000000000000 ) ) ;
#97274=CARTESIAN_POINT ( 'NONE',  ( -11.84316977508124857, 85.52578825423026387, 14.70342373635102895 ) ) ;
#97277=ORIENTED_EDGE ( 'NONE', *, *, #14742, .T. ) ;
#97291=ORIENTED_EDGE ( 'NONE', *, *, #2200, .F. ) ;
#97299=ORIENTED_EDGE ( 'NONE', *, *, #11480, .F. ) ;
#97312=FACE_BOUND ( 'NONE', #95705, .T. ) ;
#97315=DIRECTION ( 'NONE',  ( -0.3693965786901617365, 0.9292718480896766664, 0.000000000000000000 ) ) ;
#97323=CYLINDRICAL_SURFACE ( 'NONE', #8133, 70.00000000000002842 ) ;
#97324=LINE ( 'NONE', #66397, #49949 ) ;
#97330=LINE ( 'NONE', #4608, #10505 ) ;
#97340=VECTOR ( 'NONE', #26612, 1000.000000000000114 ) ;
#97342=ORIENTED_EDGE ( 'NONE', *, *, #34570, .T. ) ;
#97344=DIRECTION ( 'NONE',  ( 0.000000000000000000, 0.000000000000000000, 1.000000000000000000 ) ) ;
#97350=EDGE_CURVE ( 'NONE', #61085, #68592, #14047, .T. ) ;
#97386=DIRECTION ( 'NONE',  ( -0.03004293549037833494, -0.9995486091367047354, 0.000000000000000000 ) ) ;
#97389=DIRECTION ( 'NONE',  ( 1.000000000000000000, 0.000000000000000000, 0.000000000000000000 ) ) ;
#97392=LINE ( 'NONE', #27960, #43438 ) ;
#97395=EDGE_CURVE ( 'NONE', #20462, #56406, #81642, .T. ) ;
#97397=ORIENTED_EDGE ( 'NONE', *, *, #25039, .F. ) ;
#97400=EDGE_CURVE ( 'NONE', #64662, #84833, #28239, .T. ) ;
#97403=CARTESIAN_POINT ( 'NONE',  ( -19.65312891409030271, 93.06504152958497400, 59.99999999999999289 ) ) ;
#97407=ORIENTED_EDGE ( 'NONE', *, *, #46259, .T. ) ;
#97421=VERTEX_POINT ( 'NONE', #27259 ) ;
#97432=DIRECTION ( 'NONE',  ( -0.9213551052231903071, 0.3887219701524006754, 0.000000000000000000 ) ) ;
#97433=VERTEX_POINT ( 'NONE', #15020 ) ;
#97436=DIRECTION ( 'NONE',  ( 0.9439450758449176027, -0.3301025504114332709, 0.000000000000000000 ) ) ;
#97442=EDGE_LOOP ( 'NONE', ( #90086, #67473, #72059, #47158 ) ) ;
#97445=AXIS2_PLACEMENT_3D ( 'NONE', #44047, #74503, #5081 ) ;
#97448=DIRECTION ( 'NONE',  ( 1.000000000000000000, 0.000000000000000000, 0.000000000000000000 ) ) ;
#97449=ORIENTED_EDGE ( 'NONE', *, *, #11405, .F. ) ;
#97469=EDGE_CURVE ( 'NONE', #45532, #94007, #64645, .T. ) ;
#97475=ORIENTED_EDGE ( 'NONE', *, *, #44629, .T. ) ;
#97476=ORIENTED_EDGE ( 'NONE', *, *, #11542, .T. ) ;
#97480=EDGE_CURVE ( 'NONE', #37072, #43568, #94578, .T. ) ;
#97488=ORIENTED_EDGE ( 'NONE', *, *, #48028, .T. ) ;
#97501=ORIENTED_EDGE ( 'NONE', *, *, #91868, .T. ) ;
#97503=DIRECTION ( 'NONE',  ( 0.000000000000000000, 0.000000000000000000, 1.000000000000000000 ) ) ;
#97511=LINE ( 'NONE', #19524, #17359 ) ;
#97515=DIRECTION ( 'NONE',  ( -0.8074371744834166753, -0.5899535653441180250, 0.000000000000000000 ) ) ;
#97516=DIRECTION ( 'NONE',  ( -0.9689885751534038638, -0.2471055264905585858, 0.000000000000000000 ) ) ;
#97519=DIRECTION ( 'NONE',  ( -0.2877784213863818774, 0.9576970189910596343, 0.000000000000000000 ) ) ;
#97526=LINE ( 'NONE', #12924, #68226 ) ;
#97528=CARTESIAN_POINT ( 'NONE',  ( -71.61465314115659453, 63.06504152958490295, -25.00000000000000000 ) ) ;
#97530=CARTESIAN_POINT ( 'NONE',  ( 35.43817338645655468, 49.87999306568065805, -10.00000000000000000 ) ) ;
#97533=VERTEX_POINT ( 'NONE', #88497 ) ;
#97537=ORIENTED_EDGE ( 'NONE', *, *, #48115, .F. ) ;
#97540=DIRECTION ( 'NONE',  ( -0.6911977992267216431, 0.7226656227773233798, 0.000000000000000000 ) ) ;
#97545=EDGE_LOOP ( 'NONE', ( #57385, #37948, #13853, #89452 ) ) ;
#97551=EDGE_CURVE ( 'NONE', #95379, #24879, #88001, .T. ) ;
#97553=CARTESIAN_POINT ( 'NONE',  ( -9.093968788749004162, 61.55273967620898645, -10.00000000000000000 ) ) ;
#97555=ORIENTED_EDGE ( 'NONE', *, *, #41492, .F. ) ;
#97565=LINE ( 'NONE', #26650, #51536 ) ;
#97579=DIRECTION ( 'NONE',  ( -0.000000000000000000, 0.000000000000000000, -1.000000000000000000 ) ) ;
#97583=EDGE_CURVE ( 'NONE', #47298, #18338, #49429, .T. ) ;
#97592=DIRECTION ( 'NONE',  ( -0.9820299053580078263, -0.1887253692075926415, 0.000000000000000000 ) ) ;
#97593=DIRECTION ( 'NONE',  ( -0.5544813661758285495, -0.8321961394790213795, 0.000000000000000000 ) ) ;
#97595=CARTESIAN_POINT ( 'NONE',  ( -19.65312891409030271, 93.06504152958497400, 177.5919119679930134 ) ) ;
#97596=ORIENTED_EDGE ( 'NONE', *, *, #27995, .T. ) ;
#97598=EDGE_CURVE ( 'NONE', #65714, #49571, #29138, .T. ) ;
#97599=VERTEX_POINT ( 'NONE', #90482 ) ;
#97602=CARTESIAN_POINT ( 'NONE',  ( -19.65312891409030271, 93.06504152958497400, 10.00000000000000888 ) ) ;
#97604=EDGE_CURVE ( 'NONE', #59369, #93038, #65625, .T. ) ;
#97605=LINE ( 'NONE', #38109, #15787 ) ;
#97608=DIRECTION ( 'NONE',  ( -0.3696446237802352708, -0.9291732088853876803, 0.000000000000000000 ) ) ;
#97626=EDGE_CURVE ( 'NONE', #32206, #1197, #28124, .T. ) ;
#97653=ORIENTED_EDGE ( 'NONE', *, *, #27395, .F. ) ;
#97658=ORIENTED_EDGE ( 'NONE', *, *, #87771, .T. ) ;
#97660=CARTESIAN_POINT ( 'NONE',  ( 46.89542285554266954, 70.53237680267110932, -10.00000000000000000 ) ) ;
#97670=EDGE_CURVE ( 'NONE', #25798, #1197, #27649, .T. ) ;
#97671=ORIENTED_EDGE ( 'NONE', *, *, #45339, .F. ) ;
#97672=ORIENTED_EDGE ( 'NONE', *, *, #79077, .T. ) ;
#97678=VECTOR ( 'NONE', #8633, 1000.000000000000114 ) ;
#97683=CIRCLE ( 'NONE', #37758, 70.00000000000001421 ) ;
#97686=DIRECTION ( 'NONE',  ( -0.9909246428798921258, -0.1344185706417024839, 0.000000000000000000 ) ) ;
#97688=ORIENTED_EDGE ( 'NONE', *, *, #49730, .F. ) ;
#97697=EDGE_CURVE ( 'NONE', #58893, #87878, #20048, .T. ) ;
#97699=EDGE_LOOP ( 'NONE', ( #96621, #57249, #54039, #70183 ) ) ;
#97705=CARTESIAN_POINT ( 'NONE',  ( -55.34571675428254878, 55.61878071410718150, 59.99999999999999289 ) ) ;
#97731=AXIS2_PLACEMENT_3D ( 'NONE', #12176, #5561, #6567 ) ;
#97735=CARTESIAN_POINT ( 'NONE',  ( 49.03918259513505973, 79.59780946358317522, 177.5919119679930134 ) ) ;
#97736=CIRCLE ( 'NONE', #52372, 70.00000000000001421 ) ;
#97757=ORIENTED_EDGE ( 'NONE', *, *, #9635, .T. ) ;
#97759=ORIENTED_EDGE ( 'NONE', *, *, #27411, .F. ) ;
#97771=ORIENTED_EDGE ( 'NONE', *, *, #40293, .F. ) ;
#97774=FACE_OUTER_BOUND ( 'NONE', #43435, .T. ) ;
#97779=EDGE_CURVE ( 'NONE', #19199, #82529, #99537, .T. ) ;
#97782=EDGE_CURVE ( 'NONE', #81073, #75787, #22517, .T. ) ;
#97783=ORIENTED_EDGE ( 'NONE', *, *, #1363, .T. ) ;
#97787=ORIENTED_EDGE ( 'NONE', *, *, #12101, .F. ) ;
#97792=EDGE_CURVE ( 'NONE', #45532, #1725, #91456, .T. ) ;
#97797=LINE ( 'NONE', #82633, #12239 ) ;
#97801=VERTEX_POINT ( 'NONE', #93454 ) ;
#97804=DIRECTION ( 'NONE',  ( 0.000000000000000000, 0.000000000000000000, 1.000000000000000000 ) ) ;
#97806=ORIENTED_EDGE ( 'NONE', *, *, #23137, .T. ) ;
#97816=CARTESIAN_POINT ( 'NONE',  ( -72.92390943388483038, 47.25396573843040926, -10.00000000000000000 ) ) ;
#97818=DIRECTION ( 'NONE',  ( -0.9172102815913020235, -0.3984034379158949979, 0.000000000000000000 ) ) ;
#97820=DIRECTION ( 'NONE',  ( -0.4831861483251571054, -0.8755176446347036068, 0.000000000000000000 ) ) ;
#97821=CARTESIAN_POINT ( 'NONE',  ( 50.00170217996129907, 86.12209509027381671, -10.00000000000000000 ) ) ;
#97822=CARTESIAN_POINT ( 'NONE',  ( 49.19475937879462890, 79.05079877653317055, -10.00000000000000000 ) ) ;
#97826=ORIENTED_EDGE ( 'NONE', *, *, #91500, .F. ) ;
#97832=FACE_OUTER_BOUND ( 'NONE', #43454, .T. ) ;
#97833=ORIENTED_EDGE ( 'NONE', *, *, #53336, .F. ) ;
#97848=CARTESIAN_POINT ( 'NONE',  ( 19.18375657693640335, 36.32959363016014720, -10.00000000000000000 ) ) ;
#97852=DIRECTION ( 'NONE',  ( -0.9805290675673918876, -0.1963739994383708332, 0.000000000000000000 ) ) ;
#97862=DIRECTION ( 'NONE',  ( -1.000000000000000000, 0.000000000000000000, 0.000000000000000000 ) ) ;
#97868=VECTOR ( 'NONE', #49221, 1000.000000000000000 ) ;
#97877=VECTOR ( 'NONE', #38028, 1000.000000000000000 ) ;
#97888=ORIENTED_EDGE ( 'NONE', *, *, #33579, .F. ) ;
#97892=VERTEX_POINT ( 'NONE', #33115 ) ;
#97895=LINE ( 'NONE', #51267, #21813 ) ;
#97902=ORIENTED_EDGE ( 'NONE', *, *, #58991, .T. ) ;
#97905=FACE_OUTER_BOUND ( 'NONE', #57388, .T. ) ;
#97910=ORIENTED_EDGE ( 'NONE', *, *, #92628, .T. ) ;
#97916=ORIENTED_EDGE ( 'NONE', *, *, #66147, .T. ) ;
#97921=ORIENTED_EDGE ( 'NONE', *, *, #59683, .F. ) ;
#97926=CARTESIAN_POINT ( 'NONE',  ( -19.65312891409030271, 93.06504152958497400, -10.00000000000000888 ) ) ;
#97935=DIRECTION ( 'NONE',  ( -0.2776767122488493222, -0.9606745773021527768, 0.000000000000000000 ) ) ;
#97937=ORIENTED_EDGE ( 'NONE', *, *, #20259, .F. ) ;
#97938=LINE ( 'NONE', #14806, #17548 ) ;
#97944=DIRECTION ( 'NONE',  ( 0.2774202615135334393, -0.9607486656258038549, 0.000000000000000000 ) ) ;
#97948=VERTEX_POINT ( 'NONE', #10826 ) ;
#97969=DIRECTION ( 'NONE',  ( -0.9738769792773346312, -0.2270762630343691746, 0.000000000000000000 ) ) ;
#97988=VECTOR ( 'NONE', #68009, 1000.000000000000227 ) ;
#97995=PLANE ( 'NONE',  #86966 ) ;
#97999=ORIENTED_EDGE ( 'NONE', *, *, #26832, .F. ) ;
#98001=CARTESIAN_POINT ( 'NONE',  ( -51.75017079496729622, 30.85748650210271293, -10.00000000000000000 ) ) ;
#98005=VERTEX_POINT ( 'NONE', #78730 ) ;
#98008=VECTOR ( 'NONE', #68702, 1000.000000000000000 ) ;
#98009=EDGE_CURVE ( 'NONE', #89564, #39796, #7172, .T. ) ;
#98012=VECTOR ( 'NONE', #37614, 1000.000000000000000 ) ;
#98018=LINE ( 'NONE', #50401, #84268 ) ;
#98020=CARTESIAN_POINT ( 'NONE',  ( -20.51833308425736391, 22.81063138990083061, -10.00000000000000000 ) ) ;
#98023=CARTESIAN_POINT ( 'NONE',  ( -59.85755863633952600, 35.44530052843370527, -10.00000000000000000 ) ) ;
#98024=CARTESIAN_POINT ( 'NONE',  ( 9.830230629461709668, 30.95267373526312227, -10.00000000000000000 ) ) ;
#98025=VERTEX_POINT ( 'NONE', #71135 ) ;
#98030=CARTESIAN_POINT ( 'NONE',  ( -14.06329310883398875, 23.28858607597029007, -10.00000000000000000 ) ) ;
#98037=ORIENTED_EDGE ( 'NONE', *, *, #303, .F. ) ;
#98057=CIRCLE ( 'NONE', #44641, 70.00000000000001421 ) ;
#98066=AXIS2_PLACEMENT_3D ( 'NONE', #52692, #46585, #77523 ) ;
#98075=LINE ( 'NONE', #73281, #80653 ) ;
#98080=EDGE_CURVE ( 'NONE', #88625, #98426, #11345, .T. ) ;
#98082=EDGE_LOOP ( 'NONE', ( #81750, #51657, #35170, #99871 ) ) ;
#98085=FACE_OUTER_BOUND ( 'NONE', #90120, .T. ) ;
#98088=CARTESIAN_POINT ( 'NONE',  ( 44.10470679282202866, 121.9603419428074602, -10.00000000000000000 ) ) ;
#98092=CYLINDRICAL_SURFACE ( 'NONE', #6179, 70.00000000000002842 ) ;
#98097=EDGE_CURVE ( 'NONE', #30966, #17413, #27024, .T. ) ;
#98104=EDGE_CURVE ( 'NONE', #58060, #94071, #33072, .T. ) ;
#98107=DIRECTION ( 'NONE',  ( 0.8434505012732891327, -0.5372068985985168910, 0.000000000000000000 ) ) ;
#98109=ADVANCED_FACE ( 'NONE', ( #96962 ), #27528, .F. ) ;
#98111=CARTESIAN_POINT ( 'NONE',  ( -66.69146994933839778, 41.22495595238228105, 10.00000000000000000 ) ) ;
#98121=VECTOR ( 'NONE', #88408, 1000.000000000000000 ) ;
#98128=VECTOR ( 'NONE', #57039, 1000.000000000000000 ) ;
#98131=ADVANCED_FACE ( 'NONE', ( #19927 ), #50799, .T. ) ;
#98133=VECTOR ( 'NONE', #42331, 1000.000000000000000 ) ;
#98155=PLANE ( 'NONE',  #1319 ) ;
#98156=PLANE ( 'NONE',  #12471 ) ;
#98159=AXIS2_PLACEMENT_3D ( 'NONE', #86060, #24191, #79933 ) ;
#98160=DIRECTION ( 'NONE',  ( 1.000000000000000000, 0.000000000000000000, 0.000000000000000000 ) ) ;
#98169=CARTESIAN_POINT ( 'NONE',  ( -12.68721568607400485, 24.67147432707382748, -10.00000000000000000 ) ) ;
#98179=FACE_OUTER_BOUND ( 'NONE', #80910, .T. ) ;
#98189=ORIENTED_EDGE ( 'NONE', *, *, #61760, .T. ) ;
#98192=ORIENTED_EDGE ( 'NONE', *, *, #8507, .T. ) ;
#98194=DIRECTION ( 'NONE',  ( 0.000000000000000000, 0.000000000000000000, 1.000000000000000000 ) ) ;
#98196=VECTOR ( 'NONE', #38953, 1000.000000000000114 ) ;
#98200=DIRECTION ( 'NONE',  ( 0.3002896333693469422, 0.9538480676139692305, 0.000000000000000000 ) ) ;
#98209=LINE ( 'NONE', #29302, #13939 ) ;
#98224=ADVANCED_FACE ( 'NONE', ( #96272 ), #55702, .F. ) ;
#98229=EDGE_CURVE ( 'NONE', #19444, #10367, #94769, .T. ) ;
#98234=CARTESIAN_POINT ( 'NONE',  ( 43.83595887736691310, 122.5461495720015677, 10.00000000000000000 ) ) ;
#98248=LINE ( 'NONE', #45015, #23464 ) ;
#98266=VECTOR ( 'NONE', #4259, 1000.000000000000000 ) ;
#98268=VERTEX_POINT ( 'NONE', #3555 ) ;
#98274=EDGE_CURVE ( 'NONE', #11685, #92469, #72963, .T. ) ;
#98279=VERTEX_POINT ( 'NONE', #95296 ) ;
#98290=VERTEX_POINT ( 'NONE', #26840 ) ;
#98298=FACE_BOUND ( 'NONE', #5223, .T. ) ;
#98305=VERTEX_POINT ( 'NONE', #10649 ) ;
#98310=DIRECTION ( 'NONE',  ( -0.9213551052231903071, 0.3887219701524006754, 0.000000000000000000 ) ) ;
#98315=LINE ( 'NONE', #8461, #69112 ) ;
#98317=LINE ( 'NONE', #53554, #59107 ) ;
#98327=CARTESIAN_POINT ( 'NONE',  ( 4.061437313896076873, 69.78113336816737444, -10.00000000000000000 ) ) ;
#98332=VECTOR ( 'NONE', #66202, 1000.000000000000227 ) ;
#98338=AXIS2_PLACEMENT_3D ( 'NONE', #6154, #82214, #98875 ) ;
#98341=EDGE_CURVE ( 'NONE', #38602, #45464, #23365, .T. ) ;
#98354=AXIS2_PLACEMENT_3D ( 'NONE', #18663, #49543, #1956 ) ;
#98362=DIRECTION ( 'NONE',  ( 0.1857746241280557320, -0.9825923819316327856, 0.000000000000000000 ) ) ;
#98363=CARTESIAN_POINT ( 'NONE',  ( -61.61048871844075592, 38.59675092633816007, 10.00000000000000000 ) ) ;
#98372=EDGE_CURVE ( 'NONE', #57256, #56387, #43520, .T. ) ;
#98376=LINE ( 'NONE', #52245, #75947 ) ;
#98395=FACE_OUTER_BOUND ( 'NONE', #6690, .T. ) ;
#98405=VECTOR ( 'NONE', #50970, 1000.000000000000114 ) ;
#98411=AXIS2_PLACEMENT_3D ( 'NONE', #74298, #66659, #27682 ) ;
#98414=VERTEX_POINT ( 'NONE', #14130 ) ;
#98426=VERTEX_POINT ( 'NONE', #68315 ) ;
#98440=CARTESIAN_POINT ( 'NONE',  ( 41.82599275875796252, 62.29945068332010294, 10.00000000000000000 ) ) ;
#98454=VECTOR ( 'NONE', #74861, 1000.000000000000000 ) ;
#98459=DIRECTION ( 'NONE',  ( 1.000000000000000000, 0.000000000000000000, 0.000000000000000000 ) ) ;
#98479=VERTEX_POINT ( 'NONE', #62705 ) ;
#98481=EDGE_CURVE ( 'NONE', #90103, #54173, #40896, .T. ) ;
#98502=FACE_OUTER_BOUND ( 'NONE', #46266, .T. ) ;
#98514=CONICAL_SURFACE ( 'NONE', #51561, 11.91750000000000043, 0.7853981633974482790 ) ;
#98523=ORIENTED_EDGE ( 'NONE', *, *, #84952, .T. ) ;
#98529=DIRECTION ( 'NONE',  ( -0.000000000000000000, 0.000000000000000000, 1.000000000000000000 ) ) ;
#98533=CARTESIAN_POINT ( 'NONE',  ( -19.65312891409030271, 93.06504152958497400, 177.5919119679930134 ) ) ;
#98535=EDGE_CURVE ( 'NONE', #49424, #50507, #93663, .T. ) ;
#98537=ORIENTED_EDGE ( 'NONE', *, *, #66425, .T. ) ;
#98545=VERTEX_POINT ( 'NONE', #95682 ) ;
#98547=VERTEX_POINT ( 'NONE', #26229 ) ;
#98554=AXIS2_PLACEMENT_3D ( 'NONE', #64550, #17443, #2262 ) ;
#98556=EDGE_CURVE ( 'NONE', #14427, #89858, #13039, .T. ) ;
#98564=AXIS2_PLACEMENT_3D ( 'NONE', #49591, #3995, #3030 ) ;
#98565=EDGE_LOOP ( 'NONE', ( #96042, #4695, #47346, #76167 ) ) ;
#98567=AXIS2_PLACEMENT_3D ( 'NONE', #12233, #57808, #11250 ) ;
#98569=ORIENTED_EDGE ( 'NONE', *, *, #72669, .T. ) ;
#98574=CARTESIAN_POINT ( 'NONE',  ( 40.96864935082037817, 128.0650415295850735, -10.00000000000000888 ) ) ;
#98578=ORIENTED_EDGE ( 'NONE', *, *, #83687, .F. ) ;
#98596=CARTESIAN_POINT ( 'NONE',  ( -33.12036098009135543, 24.37273002035946590, 177.5919119679930134 ) ) ;
#98597=EDGE_CURVE ( 'NONE', #32823, #42173, #21136, .T. ) ;
#98599=DIRECTION ( 'NONE',  ( -0.3177184104407523857, 0.9481851146622171100, 0.000000000000000000 ) ) ;
#98605=CARTESIAN_POINT ( 'NONE',  ( -19.42194755839791753, 24.31068691715150010, 10.00000000000000000 ) ) ;
#98607=EDGE_CURVE ( 'NONE', #55413, #29620, #74346, .T. ) ;
#98612=CARTESIAN_POINT ( 'NONE',  ( -38.55282132941486140, 44.90941061628357289, 59.99999999999999289 ) ) ;
#98614=CARTESIAN_POINT ( 'NONE',  ( -19.54314961412049811, 92.97549661224779527, 59.99999999999999289 ) ) ;
#98615=DIRECTION ( 'NONE',  ( -0.000000000000000000, 0.000000000000000000, 1.000000000000000000 ) ) ;
#98618=CARTESIAN_POINT ( 'NONE',  ( 46.99867368304095550, 76.19044720721625197, 10.00000000000000000 ) ) ;
#98621=DIRECTION ( 'NONE',  ( -0.000000000000000000, -0.000000000000000000, 1.000000000000000000 ) ) ;
#98635=DIRECTION ( 'NONE',  ( -0.8660254037844378194, -0.5000000000000013323, -0.000000000000000000 ) ) ;
#98636=ORIENTED_EDGE ( 'NONE', *, *, #19298, .T. ) ;
#98638=LINE ( 'NONE', #36301, #28057 ) ;
#98640=DIRECTION ( 'NONE',  ( 0.6879669212057208938, 0.7257420446182799578, 0.000000000000000000 ) ) ;
#98642=DIRECTION ( 'NONE',  ( 0.000000000000000000, -0.000000000000000000, 1.000000000000000000 ) ) ;
#98644=LINE ( 'NONE', #29228, #66306 ) ;
#98647=VERTEX_POINT ( 'NONE', #42401 ) ;
#98660=VECTOR ( 'NONE', #59596, 999.9999999999998863 ) ;
#98661=PLANE ( 'NONE',  #56104 ) ;
#98667=CARTESIAN_POINT ( 'NONE',  ( -6.542761065016642341, 25.57183462804972507, -10.00000000000000000 ) ) ;
#98668=VERTEX_POINT ( 'NONE', #15484 ) ;
#98687=ORIENTED_EDGE ( 'NONE', *, *, #1085, .F. ) ;
#98689=EDGE_CURVE ( 'NONE', #61758, #85319, #100125, .T. ) ;
#98690=CARTESIAN_POINT ( 'NONE',  ( 35.19234511847571412, 113.9167680888089080, 59.99999999999999289 ) ) ;
#98698=CARTESIAN_POINT ( 'NONE',  ( 32.30839531297598910, 123.0650415295850593, 10.00000000000000888 ) ) ;
#98700=VECTOR ( 'NONE', #95972, 1000.000000000000000 ) ;
#98704=CARTESIAN_POINT ( 'NONE',  ( -49.59353317285164309, 78.63960484736190892, -10.00000000000000000 ) ) ;
#98709=PLANE ( 'NONE',  #64293 ) ;
#98710=ADVANCED_FACE ( 'NONE', ( #33076 ), #63969, .F. ) ;
#98715=DIRECTION ( 'NONE',  ( 0.9724945078367536189, 0.2329258084183680466, 0.000000000000000000 ) ) ;
#98717=ADVANCED_FACE ( 'NONE', ( #11303 ), #18387, .F. ) ;
#98724=LINE ( 'NONE', #91625, #72197 ) ;
#98746=LINE ( 'NONE', #28826, #2212 ) ;
#98755=LINE ( 'NONE', #59199, #28309 ) ;
#98761=ORIENTED_EDGE ( 'NONE', *, *, #51100, .T. ) ;
#98764=AXIS2_PLACEMENT_3D ( 'NONE', #37062, #83202, #21863 ) ;
#98766=ORIENTED_EDGE ( 'NONE', *, *, #7196, .F. ) ;
#98772=CARTESIAN_POINT ( 'NONE',  ( -48.62867196056776464, 76.78809661315139579, -10.00000000000000000 ) ) ;
#98782=ORIENTED_EDGE ( 'NONE', *, *, #39427, .T. ) ;
#98784=ORIENTED_EDGE ( 'NONE', *, *, #98229, .T. ) ;
#98786=DIRECTION ( 'NONE',  ( -0.8615733660689046669, -0.5076330711061851630, 0.000000000000000000 ) ) ;
#98789=CARTESIAN_POINT ( 'NONE',  ( -13.42108286626701386, 23.34301056334149038, 10.00000000000000000 ) ) ;
#98790=CYLINDRICAL_SURFACE ( 'NONE', #45156, 70.00000000000002842 ) ;
#98795=ORIENTED_EDGE ( 'NONE', *, *, #8469, .F. ) ;
#98802=EDGE_LOOP ( 'NONE', ( #86443, #73956, #30250, #1143 ) ) ;
#98826=CARTESIAN_POINT ( 'NONE',  ( 41.82599275875796252, 62.29945068332010294, 10.00000000000000000 ) ) ;
#98832=EDGE_CURVE ( 'NONE', #24657, #1218, #812, .T. ) ;
#98833=DIRECTION ( 'NONE',  ( -0.000000000000000000, -0.000000000000000000, -1.000000000000000000 ) ) ;
#98850=AXIS2_PLACEMENT_3D ( 'NONE', #86856, #78710, #17388 ) ;
#98864=LINE ( 'NONE', #98363, #83150 ) ;
#98875=DIRECTION ( 'NONE',  ( -0.8218955677251095215, -0.5696381972391070247, 0.000000000000000000 ) ) ;
#98876=CARTESIAN_POINT ( 'NONE',  ( 48.98810889288134263, 89.24608170897542436, 10.00000000000000000 ) ) ;
#98895=VERTEX_POINT ( 'NONE', #90811 ) ;
#98903=CARTESIAN_POINT ( 'NONE',  ( -11.09347868418370631, 60.95190685555260046, -10.00000000000000000 ) ) ;
#98905=CARTESIAN_POINT ( 'NONE',  ( 44.73065482718366326, 120.5373619841236774, 177.5919119679930134 ) ) ;
#98909=DIRECTION ( 'NONE',  ( 0.000000000000000000, 0.000000000000000000, 1.000000000000000000 ) ) ;
#98910=ORIENTED_EDGE ( 'NONE', *, *, #7775, .T. ) ;
#98912=CARTESIAN_POINT ( 'NONE',  ( -34.16292631813982439, 25.86630820016798538, -10.00000000000000000 ) ) ;
#98913=ORIENTED_EDGE ( 'NONE', *, *, #64890, .T. ) ;
#98914=EDGE_CURVE ( 'NONE', #26456, #2381, #21365, .T. ) ;
#98921=CIRCLE ( 'NONE', #8295, 70.00000000000001421 ) ;
#98923=EDGE_CURVE ( 'NONE', #38705, #14302, #47636, .T. ) ;
#98934=CARTESIAN_POINT ( 'NONE',  ( 45.29894525614688661, 66.96469553601603764, -10.00000000000000000 ) ) ;
#98936=LINE ( 'NONE', #29518, #81696 ) ;
#98939=ORIENTED_EDGE ( 'NONE', *, *, #62630, .F. ) ;
#98947=DIRECTION ( 'NONE',  ( -0.000000000000000000, -0.000000000000000000, 1.000000000000000000 ) ) ;
#98953=CARTESIAN_POINT ( 'NONE',  ( 34.05451400132101014, 48.17084265633776852, 177.5919119679930134 ) ) ;
#98958=DIRECTION ( 'NONE',  ( -0.9515606131578207005, -0.3074612162317590380, 0.000000000000000000 ) ) ;
#98966=FACE_OUTER_BOUND ( 'NONE', #37570, .T. ) ;
#98968=LINE ( 'NONE', #83284, #32131 ) ;
#98982=DIRECTION ( 'NONE',  ( -0.8755176446347037178, 0.4831861483251572165, 0.000000000000000000 ) ) ;
#98998=ORIENTED_EDGE ( 'NONE', *, *, #13604, .F. ) ;
#99002=DIRECTION ( 'NONE',  ( -0.9919422576440852790, -0.1266907948509091164, 0.000000000000000000 ) ) ;
#99004=ORIENTED_EDGE ( 'NONE', *, *, #10512, .T. ) ;
#99009=LINE ( 'NONE', #29595, #3727 ) ;
#99022=EDGE_LOOP ( 'NONE', ( #56488, #57442, #29637, #80158 ) ) ;
#99024=CYLINDRICAL_SURFACE ( 'NONE', #91247, 70.00000000000002842 ) ;
#99028=ORIENTED_EDGE ( 'NONE', *, *, #7007, .F. ) ;
#99037=ADVANCED_FACE ( 'NONE', ( #11178 ), #33455, .F. ) ;
#99040=VERTEX_POINT ( 'NONE', #57733 ) ;
#99043=VERTEX_POINT ( 'NONE', #19282 ) ;
#99056=DIRECTION ( 'NONE',  ( -0.000000000000000000, 0.000000000000000000, -1.000000000000000000 ) ) ;
#99063=CARTESIAN_POINT ( 'NONE',  ( -19.65312891409030271, 93.06504152958497400, 59.99999999999999289 ) ) ;
#99081=VERTEX_POINT ( 'NONE', #55720 ) ;
#99082=CARTESIAN_POINT ( 'NONE',  ( -19.65312891409030271, 93.06504152958497400, 177.5919119679930134 ) ) ;
#99096=VECTOR ( 'NONE', #78172, 1000.000000000000000 ) ;
#99113=VECTOR ( 'NONE', #3554, 1000.000000000000227 ) ;
#99114=PLANE ( 'NONE',  #40370 ) ;
#99122=ORIENTED_EDGE ( 'NONE', *, *, #6573, .T. ) ;
#99124=LINE ( 'NONE', #29220, #71771 ) ;
#99133=ORIENTED_EDGE ( 'NONE', *, *, #7018, .F. ) ;
#99140=FACE_OUTER_BOUND ( 'NONE', #71564, .T. ) ;
#99147=DIRECTION ( 'NONE',  ( -0.5609510170580175314, -0.8278489937552474531, 0.000000000000000000 ) ) ;
#99149=ORIENTED_EDGE ( 'NONE', *, *, #87123, .T. ) ;
#99162=EDGE_CURVE ( 'NONE', #66118, #51689, #86708, .T. ) ;
#99166=VERTEX_POINT ( 'NONE', #9676 ) ;
#99167=CYLINDRICAL_SURFACE ( 'NONE', #67378, 70.00000000000002842 ) ;
#99171=VECTOR ( 'NONE', #85012, 1000.000000000000114 ) ;
#99179=ORIENTED_EDGE ( 'NONE', *, *, #30810, .F. ) ;
#99181=ORIENTED_EDGE ( 'NONE', *, *, #2461, .T. ) ;
#99183=EDGE_LOOP ( 'NONE', ( #10880, #44279, #80141, #64111 ) ) ;
#99185=CIRCLE ( 'NONE', #11840, 70.00000000000001421 ) ;
#99190=CARTESIAN_POINT ( 'NONE',  ( 3.113790753877906159, 26.87087736965100859, 177.5919119679930134 ) ) ;
#99199=LINE ( 'NONE', #44471, #28753 ) ;
#99203=LINE ( 'NONE', #76409, #41756 ) ;
#99206=CARTESIAN_POINT ( 'NONE',  ( -25.62627769214124740, 24.57763045674671432, 10.00000000000000000 ) ) ;
#99212=FACE_OUTER_BOUND ( 'NONE', #60359, .T. ) ;
#99214=FACE_OUTER_BOUND ( 'NONE', #73531, .T. ) ;
#99242=PLANE ( 'NONE',  #8866 ) ;
#99252=LINE ( 'NONE', #83078, #27246 ) ;
#99255=DIRECTION ( 'NONE',  ( -0.000000000000000000, -0.000000000000000000, -1.000000000000000000 ) ) ;
#99265=EDGE_CURVE ( 'NONE', #53524, #48279, #90356, .T. ) ;
#99266=ADVANCED_FACE ( 'NONE', ( #82265 ), #50803, .F. ) ;
#99268=DIRECTION ( 'NONE',  ( -0.2168075248790319320, -0.9762143704923770260, 0.000000000000000000 ) ) ;
#99281=ADVANCED_FACE ( 'NONE', ( #81753 ), #43191, .F. ) ;
#99285=VERTEX_POINT ( 'NONE', #91839 ) ;
#99295=EDGE_CURVE ( 'NONE', #98305, #3124, #61387, .T. ) ;
#99304=LINE ( 'NONE', #68870, #73754 ) ;
#99317=DIRECTION ( 'NONE',  ( -1.000000000000000000, 0.000000000000000000, 0.000000000000000000 ) ) ;
#99321=CARTESIAN_POINT ( 'NONE',  ( -56.06787742410713093, 34.75406423768147590, -10.00000000000000000 ) ) ;
#99322=ORIENTED_EDGE ( 'NONE', *, *, #47301, .T. ) ;
#99330=AXIS2_PLACEMENT_3D ( 'NONE', #65832, #73959, #51652 ) ;
#99335=DIRECTION ( 'NONE',  ( 0.9377374661009790779, 0.3473448497826262527, 0.000000000000000000 ) ) ;
#99337=EDGE_CURVE ( 'NONE', #10175, #73010, #92341, .T. ) ;
#99340=DIRECTION ( 'NONE',  ( 1.000000000000000000, 0.000000000000000000, 0.000000000000000000 ) ) ;
#99360=EDGE_CURVE ( 'NONE', #21753, #78482, #69494, .T. ) ;
#99362=DIRECTION ( 'NONE',  ( 0.5344452582589497291, -0.8452030915256549815, 0.000000000000000000 ) ) ;
#99369=CARTESIAN_POINT ( 'NONE',  ( 25.34687108590969729, 93.06504152958497400, -20.00000000000000355 ) ) ;
#99379=ORIENTED_EDGE ( 'NONE', *, *, #36636, .T. ) ;
#99389=VECTOR ( 'NONE', #29811, 1000.000000000000114 ) ;
#99391=VERTEX_POINT ( 'NONE', #30993 ) ;
#99392=ADVANCED_FACE ( 'NONE', ( #86254 ), #15785, .F. ) ;
#99394=DIRECTION ( 'NONE',  ( -1.000000000000000000, 0.000000000000000000, 0.000000000000000000 ) ) ;
#99395=EDGE_LOOP ( 'NONE', ( #90832, #35744, #80398, #66737 ) ) ;
#99400=ORIENTED_EDGE ( 'NONE', *, *, #98372, .T. ) ;
#99402=VECTOR ( 'NONE', #4849, 1000.000000000000000 ) ;
#99403=EDGE_CURVE ( 'NONE', #76337, #47702, #16793, .T. ) ;
#99406=DIRECTION ( 'NONE',  ( -0.8099771808667467488, -0.5864613938488684175, 0.000000000000000000 ) ) ;
#99415=ORIENTED_EDGE ( 'NONE', *, *, #84509, .F. ) ;
#99416=EDGE_LOOP ( 'NONE', ( #33462, #29105, #28028, #95840 ) ) ;
#99427=CARTESIAN_POINT ( 'NONE',  ( 49.93886538132678510, 83.40144735776343055, 10.00000000000000000 ) ) ;
#99433=DIRECTION ( 'NONE',  ( 0.1577859398657057433, -0.9874733399847793747, 0.000000000000000000 ) ) ;
#99450=DIRECTION ( 'NONE',  ( 0.000000000000000000, -0.000000000000000000, -1.000000000000000000 ) ) ;
#99454=CARTESIAN_POINT ( 'NONE',  ( -47.89831220414404811, 41.63518499402012196, 59.99999999999999289 ) ) ;
#99458=CARTESIAN_POINT ( 'NONE',  ( -19.65312891409030271, 93.06504152958497400, 177.5919119679930134 ) ) ;
#99462=LINE ( 'NONE', #83282, #30091 ) ;
#99463=LINE ( 'NONE', #53339, #24034 ) ;
#99468=VECTOR ( 'NONE', #98640, 999.9999999999998863 ) ;
#99469=EDGE_CURVE ( 'NONE', #28472, #91263, #55766, .T. ) ;
#99479=CARTESIAN_POINT ( 'NONE',  ( -64.54732778733693976, 39.35739861417317087, 10.00000000000000000 ) ) ;
#99498=FACE_OUTER_BOUND ( 'NONE', #4688, .T. ) ;
#99505=DIRECTION ( 'NONE',  ( 0.000000000000000000, 0.000000000000000000, 1.000000000000000000 ) ) ;
#99506=DIRECTION ( 'NONE',  ( 0.000000000000000000, -0.000000000000000000, 1.000000000000000000 ) ) ;
#99511=EDGE_CURVE ( 'NONE', #81619, #38416, #36386, .T. ) ;
#99530=ORIENTED_EDGE ( 'NONE', *, *, #10359, .F. ) ;
#99535=AXIS2_PLACEMENT_3D ( 'NONE', #40185, #63505, #72125 ) ;
#99536=ORIENTED_EDGE ( 'NONE', *, *, #4231, .T. ) ;
#99537=LINE ( 'NONE', #70100, #96248 ) ;
#99548=VERTEX_POINT ( 'NONE', #56341 ) ;
#99551=FACE_OUTER_BOUND ( 'NONE', #69872, .T. ) ;
#99553=EDGE_CURVE ( 'NONE', #19564, #7924, #67127, .T. ) ;
#99559=PLANE ( 'NONE',  #46738 ) ;
#99572=ORIENTED_EDGE ( 'NONE', *, *, #30809, .F. ) ;
#99573=DIRECTION ( 'NONE',  ( -0.000000000000000000, -0.000000000000000000, 1.000000000000000000 ) ) ;
#99576=AXIS2_PLACEMENT_3D ( 'NONE', #24170, #87036, #79914 ) ;
#99586=DIRECTION ( 'NONE',  ( -1.000000000000000000, 0.000000000000000000, 0.000000000000000000 ) ) ;
#99591=CIRCLE ( 'NONE', #94766, 0.1418229129681591871 ) ;
#99599=ORIENTED_EDGE ( 'NONE', *, *, #28134, .T. ) ;
#99601=VECTOR ( 'NONE', #57632, 1000.000000000000000 ) ;
#99603=ADVANCED_FACE ( 'NONE', ( #70548 ), #48256, .F. ) ;
#99607=ADVANCED_FACE ( 'NONE', ( #9263 ), #24945, .F. ) ;
#99617=DIRECTION ( 'NONE',  ( 0.000000000000000000, 0.000000000000000000, 1.000000000000000000 ) ) ;
#99625=CARTESIAN_POINT ( 'NONE',  ( -19.55020206325906074, 92.96747205679382375, 59.99999999999999289 ) ) ;
#99629=CARTESIAN_POINT ( 'NONE',  ( 44.18794977381974576, 118.5901545549086791, -10.00000000000000000 ) ) ;
#99631=CARTESIAN_POINT ( 'NONE',  ( 43.24043327773039636, 120.8247932685368227, -10.00000000000000000 ) ) ;
#99640=LINE ( 'NONE', #69214, #673 ) ;
#99645=DIRECTION ( 'NONE',  ( 0.000000000000000000, 0.000000000000000000, 1.000000000000000000 ) ) ;
#99646=CARTESIAN_POINT ( 'NONE',  ( -3.153128914090298274, 64.48620320469859735, 0.000000000000000000 ) ) ;
#99650=ORIENTED_EDGE ( 'NONE', *, *, #39996, .T. ) ;
#99660=CARTESIAN_POINT ( 'NONE',  ( 6.792688375875571616, 72.93695720651483327, -10.00000000000000000 ) ) ;
#99665=DIRECTION ( 'NONE',  ( -0.000000000000000000, -0.000000000000000000, -1.000000000000000000 ) ) ;
#99668=EDGE_CURVE ( 'NONE', #5812, #79283, #19869, .T. ) ;
#99669=EDGE_LOOP ( 'NONE', ( #37307, #51802, #15148, #42699 ) ) ;
#99676=EDGE_LOOP ( 'NONE', ( #30254, #14159, #6817, #9237 ) ) ;
#99677=VECTOR ( 'NONE', #56456, 1000.000000000000227 ) ;
#99680=LINE ( 'NONE', #30263, #23671 ) ;
#99681=ORIENTED_EDGE ( 'NONE', *, *, #68758, .F. ) ;
#99697=FACE_OUTER_BOUND ( 'NONE', #88868, .T. ) ;
#99704=DIRECTION ( 'NONE',  ( -0.8492021815265776707, 0.5280678506503699854, 0.000000000000000000 ) ) ;
#99707=VECTOR ( 'NONE', #86031, 1000.000000000000114 ) ;
#99724=LINE ( 'NONE', #37395, #51480 ) ;
#99741=LINE ( 'NONE', #30326, #42843 ) ;
#99748=CARTESIAN_POINT ( 'NONE',  ( -25.58123355786713660, 60.36368672610149844, -10.00000000000000000 ) ) ;
#99750=LINE ( 'NONE', #55611, #33765 ) ;
#99752=CARTESIAN_POINT ( 'NONE',  ( -35.27139336136212933, 24.82964151130202879, 10.00000000000000000 ) ) ;
#99759=CARTESIAN_POINT ( 'NONE',  ( 17.38248943320504836, 35.13769309531820539, -10.00000000000000000 ) ) ;
#99761=CARTESIAN_POINT ( 'NONE',  ( -2.073866539663252073, 26.60322154129611505, 10.00000000000000000 ) ) ;
#99764=DIRECTION ( 'NONE',  ( 0.000000000000000000, 0.000000000000000000, 1.000000000000000000 ) ) ;
#99776=CARTESIAN_POINT ( 'NONE',  ( 46.43574122514301195, 74.10519008736565638, -10.00000000000000000 ) ) ;
#99777=CARTESIAN_POINT ( 'NONE',  ( -12.95261720355844126, 24.63757726406876714, 10.00000000000000000 ) ) ;
#99778=CARTESIAN_POINT ( 'NONE',  ( -19.65312891409030271, 93.06504152958497400, -10.00000000000000888 ) ) ;
#99779=CIRCLE ( 'NONE', #20530, 70.00000000000001421 ) ;
#99782=DIRECTION ( 'NONE',  ( -1.000000000000000000, 0.000000000000000000, 0.000000000000000000 ) ) ;
#99785=FACE_BOUND ( 'NONE', #87379, .T. ) ;
#99799=ORIENTED_EDGE ( 'NONE', *, *, #83257, .T. ) ;
#99800=ADVANCED_FACE ( 'NONE', ( #39387 ), #13739, .F. ) ;
#99804=CIRCLE ( 'NONE', #56091, 70.00000000000001421 ) ;
#99815=DIRECTION ( 'NONE',  ( 0.4829524219151267173, -0.8756465943326184886, 0.000000000000000000 ) ) ;
#99827=DIRECTION ( 'NONE',  ( -0.9995565931350001154, -0.02977611660965746171, 0.000000000000000000 ) ) ;
#99828=CARTESIAN_POINT ( 'NONE',  ( 4.102725850843912170, 28.55253618238880620, 10.00000000000000000 ) ) ;
#99830=EDGE_CURVE ( 'NONE', #54647, #72257, #38398, .T. ) ;
#99840=EDGE_CURVE ( 'NONE', #511, #41280, #33310, .T. ) ;
#99857=DIRECTION ( 'NONE',  ( -0.9954322480537355355, -0.09547062131716987921, 0.000000000000000000 ) ) ;
#99861=DIRECTION ( 'NONE',  ( -0.2776767122488493222, -0.9606745773021527768, 0.000000000000000000 ) ) ;
#99863=DIRECTION ( 'NONE',  ( 0.9171038997749326738, -0.3986482622784278118, 0.000000000000000000 ) ) ;
#99869=DIRECTION ( 'NONE',  ( -0.6056412518070772855, -0.7957378174433814566, 0.000000000000000000 ) ) ;
#99871=ORIENTED_EDGE ( 'NONE', *, *, #30860, .T. ) ;
#99872=VECTOR ( 'NONE', #4223, 999.9999999999998863 ) ;
#99885=VECTOR ( 'NONE', #24943, 1000.000000000000000 ) ;
#99891=DIRECTION ( 'NONE',  ( -0.8321961394790272637, 0.5544813661758195567, 0.000000000000000000 ) ) ;
#99895=EDGE_CURVE ( 'NONE', #37415, #8628, #88079, .T. ) ;
#99899=ORIENTED_EDGE ( 'NONE', *, *, #85082, .F. ) ;
#99905=CARTESIAN_POINT ( 'NONE',  ( -18.09909136273254404, 77.89501454298846284, 13.64121249152874960 ) ) ;
#99908=LINE ( 'NONE', #83738, #62810 ) ;
#99910=VERTEX_POINT ( 'NONE', #57596 ) ;
#99921=CIRCLE ( 'NONE', #80575, 70.00000000000001421 ) ;
#99922=LINE ( 'NONE', #29514, #51031 ) ;
#99934=ADVANCED_FACE ( 'NONE', ( #21128 ), #44884, .F. ) ;
#99938=ORIENTED_EDGE ( 'NONE', *, *, #13785, .T. ) ;
#99959=DIRECTION ( 'NONE',  ( 0.000000000000000000, -0.000000000000000000, 1.000000000000000000 ) ) ;
#99967=VERTEX_POINT ( 'NONE', #13521 ) ;
#99971=EDGE_CURVE ( 'NONE', #66165, #28346, #12522, .T. ) ;
#99977=ADVANCED_FACE ( 'NONE', ( #20122 ), #13031, .F. ) ;
#99991=DIRECTION ( 'NONE',  ( 1.000000000000000000, 0.000000000000000000, 0.000000000000000000 ) ) ;
#99996=ORIENTED_EDGE ( 'NONE', *, *, #91059, .T. ) ;
#100003=CIRCLE ( 'NONE', #62873, 60.00000000000002132 ) ;
#100012=DIRECTION ( 'NONE',  ( -0.4340522123146939859, 0.9008877160804890094, 0.000000000000000000 ) ) ;
#100014=ORIENTED_EDGE ( 'NONE', *, *, #14543, .T. ) ;
#100020=CARTESIAN_POINT ( 'NONE',  ( -74.97640825042664403, 52.25402898078436920, -10.00000000000000000 ) ) ;
#100021=CIRCLE ( 'NONE', #54482, 70.00000000000001421 ) ;
#100024=VERTEX_POINT ( 'NONE', #67199 ) ;
#100031=VERTEX_POINT ( 'NONE', #59582 ) ;
#100039=VECTOR ( 'NONE', #16338, 1000.000000000000114 ) ;
#100054=EDGE_CURVE ( 'NONE', #28472, #79765, #46370, .T. ) ;
#100057=EDGE_CURVE ( 'NONE', #58260, #8715, #34865, .T. ) ;
#100064=CARTESIAN_POINT ( 'NONE',  ( 44.28334795397206847, 122.1950543691075808, -10.00000000000000000 ) ) ;
#100066=DIRECTION ( 'NONE',  ( -0.8099771808667467488, -0.5864613938488684175, 0.000000000000000000 ) ) ;
#100068=CARTESIAN_POINT ( 'NONE',  ( -19.78222480474015654, 93.12376111456400452, 59.99999999999999289 ) ) ;
#100070=AXIS2_PLACEMENT_3D ( 'NONE', #44558, #59251, #51170 ) ;
#100075=VERTEX_POINT ( 'NONE', #61582 ) ;
#100076=CIRCLE ( 'NONE', #15949, 14.99999999999967848 ) ;
#100082=VECTOR ( 'NONE', #78610, 1000.000000000000000 ) ;
#100083=CARTESIAN_POINT ( 'NONE',  ( 48.16808589598787904, 104.3116767361652535, -10.00000000000000000 ) ) ;
#100085=EDGE_CURVE ( 'NONE', #88206, #11558, #46123, .T. ) ;
#100101=DIRECTION ( 'NONE',  ( -0.9954322480537355355, -0.09547062131716987921, 0.000000000000000000 ) ) ;
#100106=ORIENTED_EDGE ( 'NONE', *, *, #97400, .F. ) ;
#100113=DIRECTION ( 'NONE',  ( -0.9377374661009826307, -0.3473448497826164827, 0.000000000000000000 ) ) ;
#100120=DIRECTION ( 'NONE',  ( 0.000000000000000000, 0.000000000000000000, 1.000000000000000000 ) ) ;
#100125=LINE ( 'NONE', #99625, #99468 ) ;
#100130=LINE ( 'NONE', #69204, #17711 ) ;
#100135=ORIENTED_EDGE ( 'NONE', *, *, #8988, .T. ) ;
#100139=ORIENTED_EDGE ( 'NONE', *, *, #39316, .T. ) ;
#100140=VECTOR ( 'NONE', #88060, 1000.000000000000000 ) ;
#100147=VECTOR ( 'NONE', #90011, 1000.000000000000114 ) ;
#100148=DIRECTION ( 'NONE',  ( -1.000000000000000000, 0.000000000000000000, 0.000000000000000000 ) ) ;
#100167=EDGE_CURVE ( 'NONE', #83607, #51970, #60667, .T. ) ;
#100173=VERTEX_POINT ( 'NONE', #84438 ) ;
#100179=ADVANCED_FACE ( 'NONE', ( #38276 ), #31181, .F. ) ;
#100187=CARTESIAN_POINT ( 'NONE',  ( -19.65312891409030271, 93.06504152958497400, -10.00000000000000888 ) ) ;
#100194=DIRECTION ( 'NONE',  ( -0.4340522123146939859, 0.9008877160804890094, 0.000000000000000000 ) ) ;
#100202=DIRECTION ( 'NONE',  ( -1.000000000000000000, 0.000000000000000000, 0.000000000000000000 ) ) ;
#100219=DIRECTION ( 'NONE',  ( 1.000000000000000000, 4.361590453884542650E-15, 0.000000000000000000 ) ) ;
#100231=EDGE_CURVE ( 'NONE', #24879, #13459, #7319, .T. ) ;
#100242=DIRECTION ( 'NONE',  ( 0.000000000000000000, 0.000000000000000000, 1.000000000000000000 ) ) ;
#100244=DIRECTION ( 'NONE',  ( -0.6623377501714527993, 0.7492053821868994712, 0.000000000000000000 ) ) ;
#100252=VERTEX_POINT ( 'NONE', #98001 ) ;
#100256=ORIENTED_EDGE ( 'NONE', *, *, #6649, .F. ) ;
#100262=ORIENTED_EDGE ( 'NONE', *, *, #10832, .F. ) ;
#100267=CARTESIAN_POINT ( 'NONE',  ( -19.65312891409030271, 93.06504152958497400, 59.99999999999999289 ) ) ;
#100269=EDGE_LOOP ( 'NONE', ( #1821, #51960, #26731, #85868 ) ) ;
#100278=VECTOR ( 'NONE', #84251, 1000.000000000000114 ) ;
#100304=COLOUR_RGB('Dark Blue',0.08,0.2,0.34);
#100305=FILL_AREA_STYLE_COLOUR('',#100304);
#100306=FILL_AREA_STYLE('',(#100305));
#100307=SURFACE_STYLE_FILL_AREA(#100306);
#100308=SURFACE_SIDE_STYLE('',(#100307));
#100309=SURFACE_STYLE_USAGE(.BOTH.,#100308);
#100310=PRESENTATION_STYLE_ASSIGNMENT((#100309));
ENDSEC;
END-ISO-10303-21;
